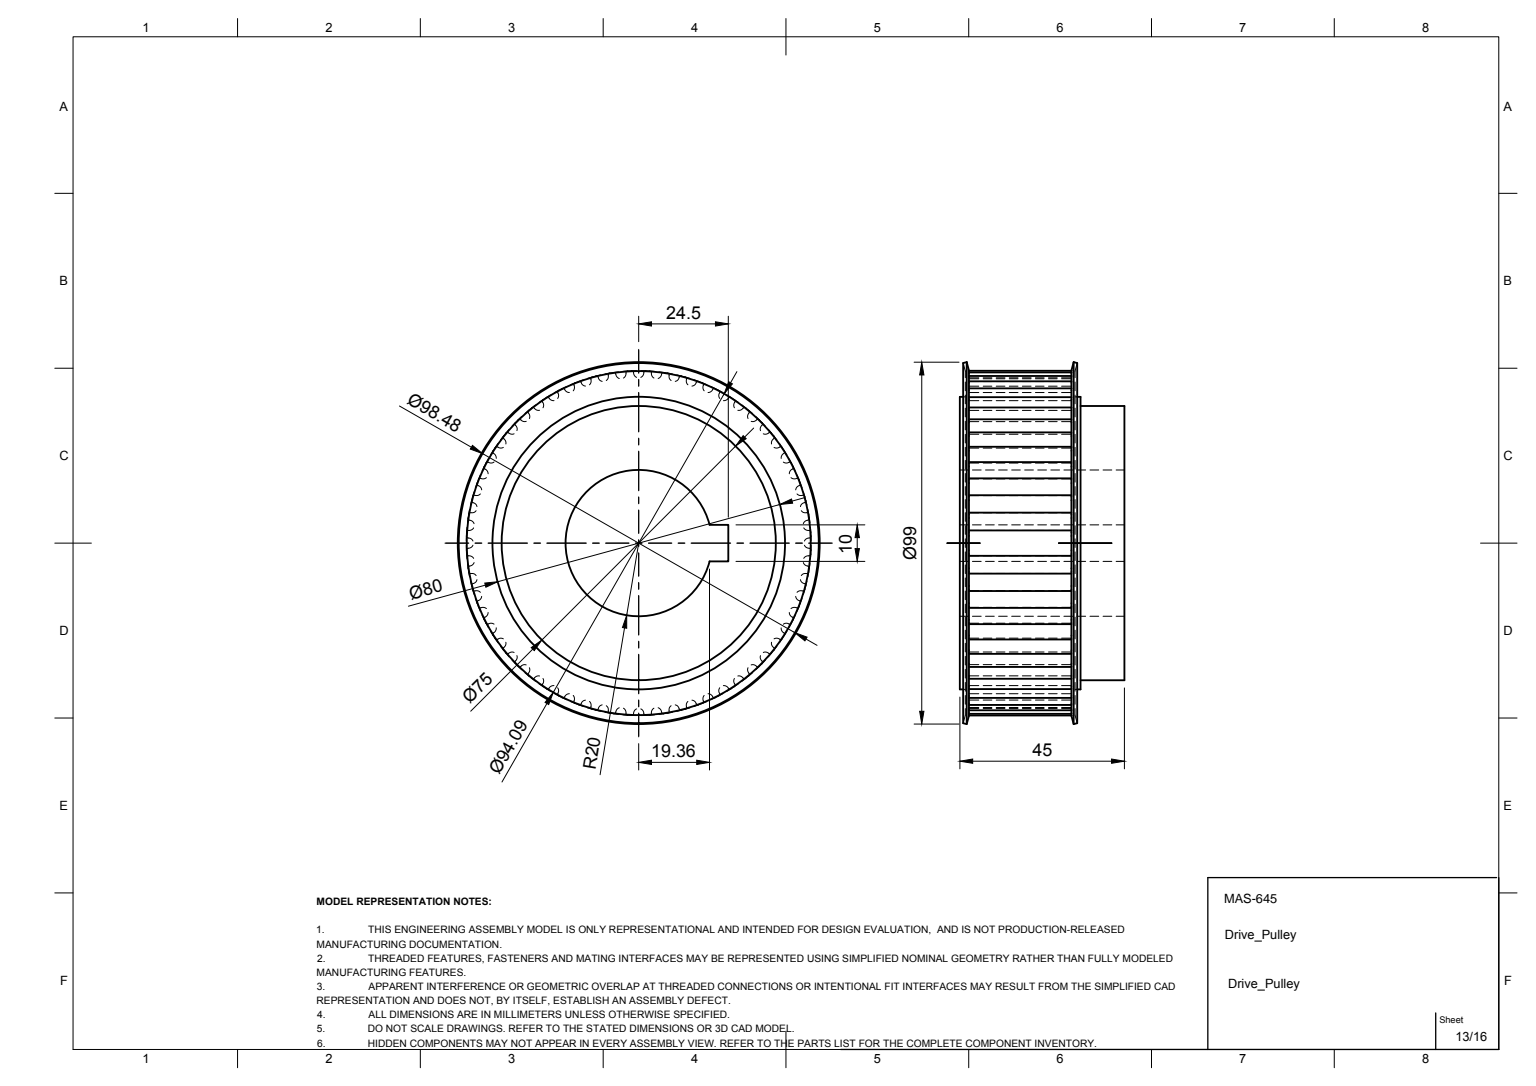
ISO-10303-21;
HEADER;
FILE_DESCRIPTION((''),'2;1');
FILE_NAME('Drive_Pulley.step','2026-10-09T10:54:55-07:00',(''),(''),'','','');
FILE_SCHEMA (('AUTOMOTIVE_DESIGN { 1 0 10303 214 3 1 1 }'));
ENDSEC;
DATA;
#10=MECHANICAL_DESIGN_GEOMETRIC_PRESENTATION_REPRESENTATION('',(#603),#63824);
#573=SHAPE_REPRESENTATION_RELATIONSHIP('SRR','None',#63887,#588) ;
#588=ADVANCED_BREP_SHAPE_REPRESENTATION('',(#618),#63817) ;
#603=STYLED_ITEM('',(#63965),#618) ;
#618=MANIFOLD_SOLID_BREP('Body1',#15502) ;
#750=FACE_BOUND('',#2823,.T.) ;
#751=FACE_BOUND('',#2886,.T.) ;
#752=FACE_BOUND('',#2894,.T.) ;
#753=FACE_BOUND('',#2897,.T.) ;
#754=FACE_BOUND('',#2900,.T.) ;
#908=PLANE('',#16209) ;
#909=PLANE('',#16210) ;
#910=PLANE('',#16211) ;
#911=PLANE('',#16212) ;
#912=PLANE('',#16397) ;
#913=PLANE('',#16536) ;
#914=PLANE('',#16540) ;
#915=PLANE('',#16544) ;
#916=PLANE('',#16546) ;
#917=PLANE('',#16550) ;
#918=PLANE('',#16557) ;
#919=PLANE('',#16561) ;
#920=PLANE('',#16568) ;
#921=PLANE('',#16572) ;
#922=PLANE('',#16579) ;
#923=PLANE('',#16583) ;
#924=PLANE('',#16590) ;
#925=PLANE('',#16594) ;
#926=PLANE('',#16601) ;
#927=PLANE('',#16605) ;
#928=PLANE('',#16612) ;
#929=PLANE('',#16616) ;
#930=PLANE('',#16623) ;
#931=PLANE('',#16627) ;
#932=PLANE('',#16634) ;
#933=PLANE('',#16638) ;
#934=PLANE('',#16645) ;
#935=PLANE('',#16649) ;
#936=PLANE('',#16656) ;
#937=PLANE('',#16660) ;
#938=PLANE('',#16667) ;
#939=PLANE('',#16671) ;
#940=PLANE('',#16678) ;
#941=PLANE('',#16682) ;
#942=PLANE('',#16689) ;
#943=PLANE('',#16693) ;
#944=PLANE('',#16700) ;
#945=PLANE('',#16704) ;
#946=PLANE('',#16711) ;
#947=PLANE('',#16715) ;
#948=PLANE('',#16722) ;
#949=PLANE('',#16726) ;
#950=PLANE('',#16733) ;
#951=PLANE('',#16737) ;
#952=PLANE('',#16744) ;
#953=PLANE('',#16748) ;
#954=PLANE('',#16755) ;
#955=PLANE('',#16759) ;
#956=PLANE('',#16766) ;
#957=PLANE('',#16770) ;
#958=PLANE('',#16777) ;
#959=PLANE('',#16781) ;
#960=PLANE('',#16788) ;
#961=PLANE('',#16792) ;
#962=PLANE('',#16799) ;
#963=PLANE('',#16803) ;
#964=PLANE('',#16810) ;
#965=PLANE('',#16814) ;
#966=PLANE('',#16821) ;
#967=PLANE('',#16825) ;
#968=PLANE('',#16832) ;
#969=PLANE('',#16836) ;
#970=PLANE('',#16843) ;
#971=PLANE('',#16847) ;
#972=PLANE('',#16854) ;
#973=PLANE('',#16858) ;
#974=PLANE('',#16865) ;
#975=PLANE('',#16869) ;
#976=PLANE('',#16876) ;
#977=PLANE('',#16880) ;
#978=PLANE('',#16887) ;
#979=PLANE('',#16891) ;
#980=PLANE('',#16898) ;
#981=PLANE('',#16902) ;
#982=PLANE('',#16909) ;
#983=PLANE('',#16913) ;
#984=PLANE('',#16920) ;
#985=PLANE('',#16924) ;
#986=PLANE('',#16931) ;
#987=PLANE('',#16935) ;
#988=PLANE('',#16942) ;
#989=PLANE('',#16946) ;
#990=PLANE('',#16953) ;
#991=PLANE('',#16957) ;
#992=PLANE('',#16964) ;
#993=PLANE('',#16968) ;
#994=PLANE('',#16975) ;
#995=PLANE('',#16979) ;
#996=PLANE('',#16986) ;
#997=PLANE('',#16990) ;
#998=PLANE('',#16997) ;
#999=PLANE('',#17001) ;
#1000=PLANE('',#17008) ;
#1001=PLANE('',#17012) ;
#1002=PLANE('',#17019) ;
#1003=PLANE('',#17023) ;
#1004=PLANE('',#17030) ;
#1005=PLANE('',#17034) ;
#1006=PLANE('',#17041) ;
#1007=PLANE('',#17045) ;
#1008=PLANE('',#17052) ;
#1009=PLANE('',#17056) ;
#1010=PLANE('',#17063) ;
#1011=PLANE('',#17067) ;
#1012=PLANE('',#17074) ;
#1013=PLANE('',#17078) ;
#1014=PLANE('',#17085) ;
#1015=PLANE('',#17089) ;
#1016=PLANE('',#17096) ;
#1017=PLANE('',#17100) ;
#1018=PLANE('',#17107) ;
#1019=PLANE('',#17111) ;
#1020=PLANE('',#17118) ;
#1021=PLANE('',#17122) ;
#1022=PLANE('',#17129) ;
#1023=PLANE('',#17133) ;
#1024=PLANE('',#17140) ;
#1025=PLANE('',#17144) ;
#1026=PLANE('',#17151) ;
#1027=PLANE('',#17155) ;
#1028=PLANE('',#17162) ;
#1029=PLANE('',#17166) ;
#1030=PLANE('',#17173) ;
#1031=PLANE('',#17177) ;
#1032=PLANE('',#17184) ;
#1033=PLANE('',#17188) ;
#1034=PLANE('',#17195) ;
#1035=PLANE('',#17199) ;
#1264=CYLINDRICAL_SURFACE('',#16215,47.175) ;
#1265=CYLINDRICAL_SURFACE('',#16218,47.175) ;
#1266=CYLINDRICAL_SURFACE('',#16221,47.175) ;
#1267=CYLINDRICAL_SURFACE('',#16224,47.175) ;
#1268=CYLINDRICAL_SURFACE('',#16227,47.175) ;
#1269=CYLINDRICAL_SURFACE('',#16230,47.175) ;
#1270=CYLINDRICAL_SURFACE('',#16233,47.175) ;
#1271=CYLINDRICAL_SURFACE('',#16236,47.175) ;
#1272=CYLINDRICAL_SURFACE('',#16239,47.175) ;
#1273=CYLINDRICAL_SURFACE('',#16242,47.175) ;
#1274=CYLINDRICAL_SURFACE('',#16245,47.175) ;
#1275=CYLINDRICAL_SURFACE('',#16248,47.175) ;
#1276=CYLINDRICAL_SURFACE('',#16251,47.175) ;
#1277=CYLINDRICAL_SURFACE('',#16254,47.175) ;
#1278=CYLINDRICAL_SURFACE('',#16257,47.175) ;
#1279=CYLINDRICAL_SURFACE('',#16260,47.175) ;
#1280=CYLINDRICAL_SURFACE('',#16263,47.175) ;
#1281=CYLINDRICAL_SURFACE('',#16266,47.175) ;
#1282=CYLINDRICAL_SURFACE('',#16269,47.175) ;
#1283=CYLINDRICAL_SURFACE('',#16272,47.175) ;
#1284=CYLINDRICAL_SURFACE('',#16275,47.175) ;
#1285=CYLINDRICAL_SURFACE('',#16278,47.175) ;
#1286=CYLINDRICAL_SURFACE('',#16281,47.175) ;
#1287=CYLINDRICAL_SURFACE('',#16284,47.175) ;
#1288=CYLINDRICAL_SURFACE('',#16287,47.175) ;
#1289=CYLINDRICAL_SURFACE('',#16290,47.175) ;
#1290=CYLINDRICAL_SURFACE('',#16293,47.175) ;
#1291=CYLINDRICAL_SURFACE('',#16296,47.175) ;
#1292=CYLINDRICAL_SURFACE('',#16299,47.175) ;
#1293=CYLINDRICAL_SURFACE('',#16302,47.175) ;
#1294=CYLINDRICAL_SURFACE('',#16305,47.175) ;
#1295=CYLINDRICAL_SURFACE('',#16308,47.175) ;
#1296=CYLINDRICAL_SURFACE('',#16311,47.175) ;
#1297=CYLINDRICAL_SURFACE('',#16314,47.175) ;
#1298=CYLINDRICAL_SURFACE('',#16317,47.175) ;
#1299=CYLINDRICAL_SURFACE('',#16320,47.175) ;
#1300=CYLINDRICAL_SURFACE('',#16323,47.175) ;
#1301=CYLINDRICAL_SURFACE('',#16326,47.175) ;
#1302=CYLINDRICAL_SURFACE('',#16329,47.175) ;
#1303=CYLINDRICAL_SURFACE('',#16332,47.175) ;
#1304=CYLINDRICAL_SURFACE('',#16335,47.175) ;
#1305=CYLINDRICAL_SURFACE('',#16338,47.175) ;
#1306=CYLINDRICAL_SURFACE('',#16341,47.175) ;
#1307=CYLINDRICAL_SURFACE('',#16344,47.175) ;
#1308=CYLINDRICAL_SURFACE('',#16347,47.175) ;
#1309=CYLINDRICAL_SURFACE('',#16350,47.175) ;
#1310=CYLINDRICAL_SURFACE('',#16353,47.175) ;
#1311=CYLINDRICAL_SURFACE('',#16356,47.175) ;
#1312=CYLINDRICAL_SURFACE('',#16359,47.175) ;
#1313=CYLINDRICAL_SURFACE('',#16362,47.175) ;
#1314=CYLINDRICAL_SURFACE('',#16365,47.175) ;
#1315=CYLINDRICAL_SURFACE('',#16368,47.175) ;
#1316=CYLINDRICAL_SURFACE('',#16371,47.175) ;
#1317=CYLINDRICAL_SURFACE('',#16374,47.175) ;
#1318=CYLINDRICAL_SURFACE('',#16377,47.175) ;
#1319=CYLINDRICAL_SURFACE('',#16380,47.175) ;
#1320=CYLINDRICAL_SURFACE('',#16383,47.175) ;
#1321=CYLINDRICAL_SURFACE('',#16386,47.175) ;
#1322=CYLINDRICAL_SURFACE('',#16389,47.175) ;
#1323=CYLINDRICAL_SURFACE('',#16392,47.175) ;
#1324=CYLINDRICAL_SURFACE('',#16395,40.) ;
#1325=CYLINDRICAL_SURFACE('',#16538,40.) ;
#1326=CYLINDRICAL_SURFACE('',#16542,37.5) ;
#1327=CYLINDRICAL_SURFACE('',#16554,0.539999999999996) ;
#1328=CYLINDRICAL_SURFACE('',#16555,1.4) ;
#1329=CYLINDRICAL_SURFACE('',#16556,0.539999999999986) ;
#1330=CYLINDRICAL_SURFACE('',#16565,0.539999999999996) ;
#1331=CYLINDRICAL_SURFACE('',#16566,1.4) ;
#1332=CYLINDRICAL_SURFACE('',#16567,0.539999999999986) ;
#1333=CYLINDRICAL_SURFACE('',#16576,0.539999999999996) ;
#1334=CYLINDRICAL_SURFACE('',#16577,1.4) ;
#1335=CYLINDRICAL_SURFACE('',#16578,0.539999999999986) ;
#1336=CYLINDRICAL_SURFACE('',#16587,0.539999999999996) ;
#1337=CYLINDRICAL_SURFACE('',#16588,1.4) ;
#1338=CYLINDRICAL_SURFACE('',#16589,0.539999999999986) ;
#1339=CYLINDRICAL_SURFACE('',#16598,0.539999999999996) ;
#1340=CYLINDRICAL_SURFACE('',#16599,1.4) ;
#1341=CYLINDRICAL_SURFACE('',#16600,0.539999999999986) ;
#1342=CYLINDRICAL_SURFACE('',#16609,0.539999999999996) ;
#1343=CYLINDRICAL_SURFACE('',#16610,1.4) ;
#1344=CYLINDRICAL_SURFACE('',#16611,0.539999999999986) ;
#1345=CYLINDRICAL_SURFACE('',#16620,0.539999999999996) ;
#1346=CYLINDRICAL_SURFACE('',#16621,1.4) ;
#1347=CYLINDRICAL_SURFACE('',#16622,0.539999999999986) ;
#1348=CYLINDRICAL_SURFACE('',#16631,0.539999999999996) ;
#1349=CYLINDRICAL_SURFACE('',#16632,1.4) ;
#1350=CYLINDRICAL_SURFACE('',#16633,0.539999999999986) ;
#1351=CYLINDRICAL_SURFACE('',#16642,0.539999999999996) ;
#1352=CYLINDRICAL_SURFACE('',#16643,1.4) ;
#1353=CYLINDRICAL_SURFACE('',#16644,0.539999999999986) ;
#1354=CYLINDRICAL_SURFACE('',#16653,0.539999999999996) ;
#1355=CYLINDRICAL_SURFACE('',#16654,1.4) ;
#1356=CYLINDRICAL_SURFACE('',#16655,0.539999999999986) ;
#1357=CYLINDRICAL_SURFACE('',#16664,0.539999999999996) ;
#1358=CYLINDRICAL_SURFACE('',#16665,1.4) ;
#1359=CYLINDRICAL_SURFACE('',#16666,0.539999999999986) ;
#1360=CYLINDRICAL_SURFACE('',#16675,0.539999999999996) ;
#1361=CYLINDRICAL_SURFACE('',#16676,1.4) ;
#1362=CYLINDRICAL_SURFACE('',#16677,0.539999999999986) ;
#1363=CYLINDRICAL_SURFACE('',#16686,0.539999999999996) ;
#1364=CYLINDRICAL_SURFACE('',#16687,1.4) ;
#1365=CYLINDRICAL_SURFACE('',#16688,0.539999999999986) ;
#1366=CYLINDRICAL_SURFACE('',#16697,0.539999999999996) ;
#1367=CYLINDRICAL_SURFACE('',#16698,1.4) ;
#1368=CYLINDRICAL_SURFACE('',#16699,0.539999999999986) ;
#1369=CYLINDRICAL_SURFACE('',#16708,0.539999999999996) ;
#1370=CYLINDRICAL_SURFACE('',#16709,1.4) ;
#1371=CYLINDRICAL_SURFACE('',#16710,0.539999999999986) ;
#1372=CYLINDRICAL_SURFACE('',#16719,0.539999999999996) ;
#1373=CYLINDRICAL_SURFACE('',#16720,1.4) ;
#1374=CYLINDRICAL_SURFACE('',#16721,0.539999999999986) ;
#1375=CYLINDRICAL_SURFACE('',#16730,0.539999999999996) ;
#1376=CYLINDRICAL_SURFACE('',#16731,1.4) ;
#1377=CYLINDRICAL_SURFACE('',#16732,0.539999999999986) ;
#1378=CYLINDRICAL_SURFACE('',#16741,0.539999999999996) ;
#1379=CYLINDRICAL_SURFACE('',#16742,1.4) ;
#1380=CYLINDRICAL_SURFACE('',#16743,0.539999999999986) ;
#1381=CYLINDRICAL_SURFACE('',#16752,0.539999999999996) ;
#1382=CYLINDRICAL_SURFACE('',#16753,1.4) ;
#1383=CYLINDRICAL_SURFACE('',#16754,0.539999999999986) ;
#1384=CYLINDRICAL_SURFACE('',#16763,0.539999999999996) ;
#1385=CYLINDRICAL_SURFACE('',#16764,1.4) ;
#1386=CYLINDRICAL_SURFACE('',#16765,0.539999999999986) ;
#1387=CYLINDRICAL_SURFACE('',#16774,0.539999999999996) ;
#1388=CYLINDRICAL_SURFACE('',#16775,1.4) ;
#1389=CYLINDRICAL_SURFACE('',#16776,0.539999999999986) ;
#1390=CYLINDRICAL_SURFACE('',#16785,0.539999999999996) ;
#1391=CYLINDRICAL_SURFACE('',#16786,1.4) ;
#1392=CYLINDRICAL_SURFACE('',#16787,0.539999999999986) ;
#1393=CYLINDRICAL_SURFACE('',#16796,0.539999999999996) ;
#1394=CYLINDRICAL_SURFACE('',#16797,1.4) ;
#1395=CYLINDRICAL_SURFACE('',#16798,0.539999999999986) ;
#1396=CYLINDRICAL_SURFACE('',#16807,0.539999999999996) ;
#1397=CYLINDRICAL_SURFACE('',#16808,1.4) ;
#1398=CYLINDRICAL_SURFACE('',#16809,0.539999999999986) ;
#1399=CYLINDRICAL_SURFACE('',#16818,0.539999999999996) ;
#1400=CYLINDRICAL_SURFACE('',#16819,1.4) ;
#1401=CYLINDRICAL_SURFACE('',#16820,0.539999999999986) ;
#1402=CYLINDRICAL_SURFACE('',#16829,0.539999999999996) ;
#1403=CYLINDRICAL_SURFACE('',#16830,1.4) ;
#1404=CYLINDRICAL_SURFACE('',#16831,0.539999999999986) ;
#1405=CYLINDRICAL_SURFACE('',#16840,0.539999999999996) ;
#1406=CYLINDRICAL_SURFACE('',#16841,1.4) ;
#1407=CYLINDRICAL_SURFACE('',#16842,0.539999999999986) ;
#1408=CYLINDRICAL_SURFACE('',#16851,0.539999999999996) ;
#1409=CYLINDRICAL_SURFACE('',#16852,1.4) ;
#1410=CYLINDRICAL_SURFACE('',#16853,0.539999999999986) ;
#1411=CYLINDRICAL_SURFACE('',#16862,0.539999999999996) ;
#1412=CYLINDRICAL_SURFACE('',#16863,1.4) ;
#1413=CYLINDRICAL_SURFACE('',#16864,0.539999999999986) ;
#1414=CYLINDRICAL_SURFACE('',#16873,0.539999999999996) ;
#1415=CYLINDRICAL_SURFACE('',#16874,1.4) ;
#1416=CYLINDRICAL_SURFACE('',#16875,0.539999999999986) ;
#1417=CYLINDRICAL_SURFACE('',#16884,0.539999999999996) ;
#1418=CYLINDRICAL_SURFACE('',#16885,1.4) ;
#1419=CYLINDRICAL_SURFACE('',#16886,0.539999999999986) ;
#1420=CYLINDRICAL_SURFACE('',#16895,0.539999999999996) ;
#1421=CYLINDRICAL_SURFACE('',#16896,1.4) ;
#1422=CYLINDRICAL_SURFACE('',#16897,0.539999999999986) ;
#1423=CYLINDRICAL_SURFACE('',#16906,0.539999999999996) ;
#1424=CYLINDRICAL_SURFACE('',#16907,1.4) ;
#1425=CYLINDRICAL_SURFACE('',#16908,0.539999999999986) ;
#1426=CYLINDRICAL_SURFACE('',#16917,0.539999999999996) ;
#1427=CYLINDRICAL_SURFACE('',#16918,1.4) ;
#1428=CYLINDRICAL_SURFACE('',#16919,0.539999999999986) ;
#1429=CYLINDRICAL_SURFACE('',#16928,0.539999999999996) ;
#1430=CYLINDRICAL_SURFACE('',#16929,1.4) ;
#1431=CYLINDRICAL_SURFACE('',#16930,0.539999999999986) ;
#1432=CYLINDRICAL_SURFACE('',#16939,0.539999999999996) ;
#1433=CYLINDRICAL_SURFACE('',#16940,1.4) ;
#1434=CYLINDRICAL_SURFACE('',#16941,0.539999999999986) ;
#1435=CYLINDRICAL_SURFACE('',#16950,0.539999999999996) ;
#1436=CYLINDRICAL_SURFACE('',#16951,1.4) ;
#1437=CYLINDRICAL_SURFACE('',#16952,0.539999999999986) ;
#1438=CYLINDRICAL_SURFACE('',#16961,0.539999999999996) ;
#1439=CYLINDRICAL_SURFACE('',#16962,1.4) ;
#1440=CYLINDRICAL_SURFACE('',#16963,0.539999999999986) ;
#1441=CYLINDRICAL_SURFACE('',#16972,0.539999999999996) ;
#1442=CYLINDRICAL_SURFACE('',#16973,1.4) ;
#1443=CYLINDRICAL_SURFACE('',#16974,0.539999999999986) ;
#1444=CYLINDRICAL_SURFACE('',#16983,0.539999999999996) ;
#1445=CYLINDRICAL_SURFACE('',#16984,1.4) ;
#1446=CYLINDRICAL_SURFACE('',#16985,0.539999999999986) ;
#1447=CYLINDRICAL_SURFACE('',#16994,0.539999999999996) ;
#1448=CYLINDRICAL_SURFACE('',#16995,1.4) ;
#1449=CYLINDRICAL_SURFACE('',#16996,0.539999999999986) ;
#1450=CYLINDRICAL_SURFACE('',#17005,0.539999999999996) ;
#1451=CYLINDRICAL_SURFACE('',#17006,1.4) ;
#1452=CYLINDRICAL_SURFACE('',#17007,0.539999999999986) ;
#1453=CYLINDRICAL_SURFACE('',#17016,0.539999999999996) ;
#1454=CYLINDRICAL_SURFACE('',#17017,1.4) ;
#1455=CYLINDRICAL_SURFACE('',#17018,0.539999999999986) ;
#1456=CYLINDRICAL_SURFACE('',#17027,0.539999999999996) ;
#1457=CYLINDRICAL_SURFACE('',#17028,1.4) ;
#1458=CYLINDRICAL_SURFACE('',#17029,0.539999999999986) ;
#1459=CYLINDRICAL_SURFACE('',#17038,0.539999999999996) ;
#1460=CYLINDRICAL_SURFACE('',#17039,1.4) ;
#1461=CYLINDRICAL_SURFACE('',#17040,0.539999999999986) ;
#1462=CYLINDRICAL_SURFACE('',#17049,0.539999999999996) ;
#1463=CYLINDRICAL_SURFACE('',#17050,1.4) ;
#1464=CYLINDRICAL_SURFACE('',#17051,0.539999999999986) ;
#1465=CYLINDRICAL_SURFACE('',#17060,0.539999999999996) ;
#1466=CYLINDRICAL_SURFACE('',#17061,1.4) ;
#1467=CYLINDRICAL_SURFACE('',#17062,0.539999999999986) ;
#1468=CYLINDRICAL_SURFACE('',#17071,0.539999999999996) ;
#1469=CYLINDRICAL_SURFACE('',#17072,1.4) ;
#1470=CYLINDRICAL_SURFACE('',#17073,0.539999999999986) ;
#1471=CYLINDRICAL_SURFACE('',#17082,0.539999999999996) ;
#1472=CYLINDRICAL_SURFACE('',#17083,1.4) ;
#1473=CYLINDRICAL_SURFACE('',#17084,0.539999999999986) ;
#1474=CYLINDRICAL_SURFACE('',#17093,0.539999999999996) ;
#1475=CYLINDRICAL_SURFACE('',#17094,1.4) ;
#1476=CYLINDRICAL_SURFACE('',#17095,0.539999999999986) ;
#1477=CYLINDRICAL_SURFACE('',#17104,0.539999999999996) ;
#1478=CYLINDRICAL_SURFACE('',#17105,1.4) ;
#1479=CYLINDRICAL_SURFACE('',#17106,0.539999999999986) ;
#1480=CYLINDRICAL_SURFACE('',#17115,0.539999999999996) ;
#1481=CYLINDRICAL_SURFACE('',#17116,1.4) ;
#1482=CYLINDRICAL_SURFACE('',#17117,0.539999999999986) ;
#1483=CYLINDRICAL_SURFACE('',#17126,0.539999999999996) ;
#1484=CYLINDRICAL_SURFACE('',#17127,1.4) ;
#1485=CYLINDRICAL_SURFACE('',#17128,0.539999999999986) ;
#1486=CYLINDRICAL_SURFACE('',#17137,0.539999999999996) ;
#1487=CYLINDRICAL_SURFACE('',#17138,1.4) ;
#1488=CYLINDRICAL_SURFACE('',#17139,0.539999999999986) ;
#1489=CYLINDRICAL_SURFACE('',#17148,0.539999999999996) ;
#1490=CYLINDRICAL_SURFACE('',#17149,1.4) ;
#1491=CYLINDRICAL_SURFACE('',#17150,0.539999999999986) ;
#1492=CYLINDRICAL_SURFACE('',#17159,0.539999999999996) ;
#1493=CYLINDRICAL_SURFACE('',#17160,1.4) ;
#1494=CYLINDRICAL_SURFACE('',#17161,0.539999999999986) ;
#1495=CYLINDRICAL_SURFACE('',#17170,0.539999999999996) ;
#1496=CYLINDRICAL_SURFACE('',#17171,1.4) ;
#1497=CYLINDRICAL_SURFACE('',#17172,0.539999999999986) ;
#1498=CYLINDRICAL_SURFACE('',#17181,0.539999999999996) ;
#1499=CYLINDRICAL_SURFACE('',#17182,1.4) ;
#1500=CYLINDRICAL_SURFACE('',#17183,0.539999999999986) ;
#1501=CYLINDRICAL_SURFACE('',#17192,0.539999999999996) ;
#1502=CYLINDRICAL_SURFACE('',#17193,1.4) ;
#1503=CYLINDRICAL_SURFACE('',#17194,0.539999999999986) ;
#1504=CYLINDRICAL_SURFACE('',#17203,0.539999999999996) ;
#1505=CYLINDRICAL_SURFACE('',#17204,1.4) ;
#1506=CYLINDRICAL_SURFACE('',#17205,0.539999999999986) ;
#1507=CYLINDRICAL_SURFACE('',#17206,20.) ;
#1833=FACE_OUTER_BOUND('',#2819,.T.) ;
#1834=FACE_OUTER_BOUND('',#2820,.T.) ;
#1835=FACE_OUTER_BOUND('',#2821,.T.) ;
#1836=FACE_OUTER_BOUND('',#2822,.T.) ;
#1837=FACE_OUTER_BOUND('',#2824,.T.) ;
#1838=FACE_OUTER_BOUND('',#2825,.T.) ;
#1839=FACE_OUTER_BOUND('',#2826,.T.) ;
#1840=FACE_OUTER_BOUND('',#2827,.T.) ;
#1841=FACE_OUTER_BOUND('',#2828,.T.) ;
#1842=FACE_OUTER_BOUND('',#2829,.T.) ;
#1843=FACE_OUTER_BOUND('',#2830,.T.) ;
#1844=FACE_OUTER_BOUND('',#2831,.T.) ;
#1845=FACE_OUTER_BOUND('',#2832,.T.) ;
#1846=FACE_OUTER_BOUND('',#2833,.T.) ;
#1847=FACE_OUTER_BOUND('',#2834,.T.) ;
#1848=FACE_OUTER_BOUND('',#2835,.T.) ;
#1849=FACE_OUTER_BOUND('',#2836,.T.) ;
#1850=FACE_OUTER_BOUND('',#2837,.T.) ;
#1851=FACE_OUTER_BOUND('',#2838,.T.) ;
#1852=FACE_OUTER_BOUND('',#2839,.T.) ;
#1853=FACE_OUTER_BOUND('',#2840,.T.) ;
#1854=FACE_OUTER_BOUND('',#2841,.T.) ;
#1855=FACE_OUTER_BOUND('',#2842,.T.) ;
#1856=FACE_OUTER_BOUND('',#2843,.T.) ;
#1857=FACE_OUTER_BOUND('',#2844,.T.) ;
#1858=FACE_OUTER_BOUND('',#2845,.T.) ;
#1859=FACE_OUTER_BOUND('',#2846,.T.) ;
#1860=FACE_OUTER_BOUND('',#2847,.T.) ;
#1861=FACE_OUTER_BOUND('',#2848,.T.) ;
#1862=FACE_OUTER_BOUND('',#2849,.T.) ;
#1863=FACE_OUTER_BOUND('',#2850,.T.) ;
#1864=FACE_OUTER_BOUND('',#2851,.T.) ;
#1865=FACE_OUTER_BOUND('',#2852,.T.) ;
#1866=FACE_OUTER_BOUND('',#2853,.T.) ;
#1867=FACE_OUTER_BOUND('',#2854,.T.) ;
#1868=FACE_OUTER_BOUND('',#2855,.T.) ;
#1869=FACE_OUTER_BOUND('',#2856,.T.) ;
#1870=FACE_OUTER_BOUND('',#2857,.T.) ;
#1871=FACE_OUTER_BOUND('',#2858,.T.) ;
#1872=FACE_OUTER_BOUND('',#2859,.T.) ;
#1873=FACE_OUTER_BOUND('',#2860,.T.) ;
#1874=FACE_OUTER_BOUND('',#2861,.T.) ;
#1875=FACE_OUTER_BOUND('',#2862,.T.) ;
#1876=FACE_OUTER_BOUND('',#2863,.T.) ;
#1877=FACE_OUTER_BOUND('',#2864,.T.) ;
#1878=FACE_OUTER_BOUND('',#2865,.T.) ;
#1879=FACE_OUTER_BOUND('',#2866,.T.) ;
#1880=FACE_OUTER_BOUND('',#2867,.T.) ;
#1881=FACE_OUTER_BOUND('',#2868,.T.) ;
#1882=FACE_OUTER_BOUND('',#2869,.T.) ;
#1883=FACE_OUTER_BOUND('',#2870,.T.) ;
#1884=FACE_OUTER_BOUND('',#2871,.T.) ;
#1885=FACE_OUTER_BOUND('',#2872,.T.) ;
#1886=FACE_OUTER_BOUND('',#2873,.T.) ;
#1887=FACE_OUTER_BOUND('',#2874,.T.) ;
#1888=FACE_OUTER_BOUND('',#2875,.T.) ;
#1889=FACE_OUTER_BOUND('',#2876,.T.) ;
#1890=FACE_OUTER_BOUND('',#2877,.T.) ;
#1891=FACE_OUTER_BOUND('',#2878,.T.) ;
#1892=FACE_OUTER_BOUND('',#2879,.T.) ;
#1893=FACE_OUTER_BOUND('',#2880,.T.) ;
#1894=FACE_OUTER_BOUND('',#2881,.T.) ;
#1895=FACE_OUTER_BOUND('',#2882,.T.) ;
#1896=FACE_OUTER_BOUND('',#2883,.T.) ;
#1897=FACE_OUTER_BOUND('',#2884,.T.) ;
#1898=FACE_OUTER_BOUND('',#2885,.T.) ;
#1899=FACE_OUTER_BOUND('',#2887,.T.) ;
#1900=FACE_OUTER_BOUND('',#2888,.T.) ;
#1901=FACE_OUTER_BOUND('',#2889,.T.) ;
#1902=FACE_OUTER_BOUND('',#2890,.T.) ;
#1903=FACE_OUTER_BOUND('',#2891,.T.) ;
#1904=FACE_OUTER_BOUND('',#2892,.T.) ;
#1905=FACE_OUTER_BOUND('',#2893,.T.) ;
#1906=FACE_OUTER_BOUND('',#2895,.T.) ;
#1907=FACE_OUTER_BOUND('',#2896,.T.) ;
#1908=FACE_OUTER_BOUND('',#2898,.T.) ;
#1909=FACE_OUTER_BOUND('',#2899,.T.) ;
#1910=FACE_OUTER_BOUND('',#2901,.T.) ;
#1911=FACE_OUTER_BOUND('',#2902,.T.) ;
#1912=FACE_OUTER_BOUND('',#2903,.T.) ;
#1913=FACE_OUTER_BOUND('',#2904,.T.) ;
#1914=FACE_OUTER_BOUND('',#2905,.T.) ;
#1915=FACE_OUTER_BOUND('',#2906,.T.) ;
#1916=FACE_OUTER_BOUND('',#2907,.T.) ;
#1917=FACE_OUTER_BOUND('',#2908,.T.) ;
#1918=FACE_OUTER_BOUND('',#2909,.T.) ;
#1919=FACE_OUTER_BOUND('',#2910,.T.) ;
#1920=FACE_OUTER_BOUND('',#2911,.T.) ;
#1921=FACE_OUTER_BOUND('',#2912,.T.) ;
#1922=FACE_OUTER_BOUND('',#2913,.T.) ;
#1923=FACE_OUTER_BOUND('',#2914,.T.) ;
#1924=FACE_OUTER_BOUND('',#2915,.T.) ;
#1925=FACE_OUTER_BOUND('',#2916,.T.) ;
#1926=FACE_OUTER_BOUND('',#2917,.T.) ;
#1927=FACE_OUTER_BOUND('',#2918,.T.) ;
#1928=FACE_OUTER_BOUND('',#2919,.T.) ;
#1929=FACE_OUTER_BOUND('',#2920,.T.) ;
#1930=FACE_OUTER_BOUND('',#2921,.T.) ;
#1931=FACE_OUTER_BOUND('',#2922,.T.) ;
#1932=FACE_OUTER_BOUND('',#2923,.T.) ;
#1933=FACE_OUTER_BOUND('',#2924,.T.) ;
#1934=FACE_OUTER_BOUND('',#2925,.T.) ;
#1935=FACE_OUTER_BOUND('',#2926,.T.) ;
#1936=FACE_OUTER_BOUND('',#2927,.T.) ;
#1937=FACE_OUTER_BOUND('',#2928,.T.) ;
#1938=FACE_OUTER_BOUND('',#2929,.T.) ;
#1939=FACE_OUTER_BOUND('',#2930,.T.) ;
#1940=FACE_OUTER_BOUND('',#2931,.T.) ;
#1941=FACE_OUTER_BOUND('',#2932,.T.) ;
#1942=FACE_OUTER_BOUND('',#2933,.T.) ;
#1943=FACE_OUTER_BOUND('',#2934,.T.) ;
#1944=FACE_OUTER_BOUND('',#2935,.T.) ;
#1945=FACE_OUTER_BOUND('',#2936,.T.) ;
#1946=FACE_OUTER_BOUND('',#2937,.T.) ;
#1947=FACE_OUTER_BOUND('',#2938,.T.) ;
#1948=FACE_OUTER_BOUND('',#2939,.T.) ;
#1949=FACE_OUTER_BOUND('',#2940,.T.) ;
#1950=FACE_OUTER_BOUND('',#2941,.T.) ;
#1951=FACE_OUTER_BOUND('',#2942,.T.) ;
#1952=FACE_OUTER_BOUND('',#2943,.T.) ;
#1953=FACE_OUTER_BOUND('',#2944,.T.) ;
#1954=FACE_OUTER_BOUND('',#2945,.T.) ;
#1955=FACE_OUTER_BOUND('',#2946,.T.) ;
#1956=FACE_OUTER_BOUND('',#2947,.T.) ;
#1957=FACE_OUTER_BOUND('',#2948,.T.) ;
#1958=FACE_OUTER_BOUND('',#2949,.T.) ;
#1959=FACE_OUTER_BOUND('',#2950,.T.) ;
#1960=FACE_OUTER_BOUND('',#2951,.T.) ;
#1961=FACE_OUTER_BOUND('',#2952,.T.) ;
#1962=FACE_OUTER_BOUND('',#2953,.T.) ;
#1963=FACE_OUTER_BOUND('',#2954,.T.) ;
#1964=FACE_OUTER_BOUND('',#2955,.T.) ;
#1965=FACE_OUTER_BOUND('',#2956,.T.) ;
#1966=FACE_OUTER_BOUND('',#2957,.T.) ;
#1967=FACE_OUTER_BOUND('',#2958,.T.) ;
#1968=FACE_OUTER_BOUND('',#2959,.T.) ;
#1969=FACE_OUTER_BOUND('',#2960,.T.) ;
#1970=FACE_OUTER_BOUND('',#2961,.T.) ;
#1971=FACE_OUTER_BOUND('',#2962,.T.) ;
#1972=FACE_OUTER_BOUND('',#2963,.T.) ;
#1973=FACE_OUTER_BOUND('',#2964,.T.) ;
#1974=FACE_OUTER_BOUND('',#2965,.T.) ;
#1975=FACE_OUTER_BOUND('',#2966,.T.) ;
#1976=FACE_OUTER_BOUND('',#2967,.T.) ;
#1977=FACE_OUTER_BOUND('',#2968,.T.) ;
#1978=FACE_OUTER_BOUND('',#2969,.T.) ;
#1979=FACE_OUTER_BOUND('',#2970,.T.) ;
#1980=FACE_OUTER_BOUND('',#2971,.T.) ;
#1981=FACE_OUTER_BOUND('',#2972,.T.) ;
#1982=FACE_OUTER_BOUND('',#2973,.T.) ;
#1983=FACE_OUTER_BOUND('',#2974,.T.) ;
#1984=FACE_OUTER_BOUND('',#2975,.T.) ;
#1985=FACE_OUTER_BOUND('',#2976,.T.) ;
#1986=FACE_OUTER_BOUND('',#2977,.T.) ;
#1987=FACE_OUTER_BOUND('',#2978,.T.) ;
#1988=FACE_OUTER_BOUND('',#2979,.T.) ;
#1989=FACE_OUTER_BOUND('',#2980,.T.) ;
#1990=FACE_OUTER_BOUND('',#2981,.T.) ;
#1991=FACE_OUTER_BOUND('',#2982,.T.) ;
#1992=FACE_OUTER_BOUND('',#2983,.T.) ;
#1993=FACE_OUTER_BOUND('',#2984,.T.) ;
#1994=FACE_OUTER_BOUND('',#2985,.T.) ;
#1995=FACE_OUTER_BOUND('',#2986,.T.) ;
#1996=FACE_OUTER_BOUND('',#2987,.T.) ;
#1997=FACE_OUTER_BOUND('',#2988,.T.) ;
#1998=FACE_OUTER_BOUND('',#2989,.T.) ;
#1999=FACE_OUTER_BOUND('',#2990,.T.) ;
#2000=FACE_OUTER_BOUND('',#2991,.T.) ;
#2001=FACE_OUTER_BOUND('',#2992,.T.) ;
#2002=FACE_OUTER_BOUND('',#2993,.T.) ;
#2003=FACE_OUTER_BOUND('',#2994,.T.) ;
#2004=FACE_OUTER_BOUND('',#2995,.T.) ;
#2005=FACE_OUTER_BOUND('',#2996,.T.) ;
#2006=FACE_OUTER_BOUND('',#2997,.T.) ;
#2007=FACE_OUTER_BOUND('',#2998,.T.) ;
#2008=FACE_OUTER_BOUND('',#2999,.T.) ;
#2009=FACE_OUTER_BOUND('',#3000,.T.) ;
#2010=FACE_OUTER_BOUND('',#3001,.T.) ;
#2011=FACE_OUTER_BOUND('',#3002,.T.) ;
#2012=FACE_OUTER_BOUND('',#3003,.T.) ;
#2013=FACE_OUTER_BOUND('',#3004,.T.) ;
#2014=FACE_OUTER_BOUND('',#3005,.T.) ;
#2015=FACE_OUTER_BOUND('',#3006,.T.) ;
#2016=FACE_OUTER_BOUND('',#3007,.T.) ;
#2017=FACE_OUTER_BOUND('',#3008,.T.) ;
#2018=FACE_OUTER_BOUND('',#3009,.T.) ;
#2019=FACE_OUTER_BOUND('',#3010,.T.) ;
#2020=FACE_OUTER_BOUND('',#3011,.T.) ;
#2021=FACE_OUTER_BOUND('',#3012,.T.) ;
#2022=FACE_OUTER_BOUND('',#3013,.T.) ;
#2023=FACE_OUTER_BOUND('',#3014,.T.) ;
#2024=FACE_OUTER_BOUND('',#3015,.T.) ;
#2025=FACE_OUTER_BOUND('',#3016,.T.) ;
#2026=FACE_OUTER_BOUND('',#3017,.T.) ;
#2027=FACE_OUTER_BOUND('',#3018,.T.) ;
#2028=FACE_OUTER_BOUND('',#3019,.T.) ;
#2029=FACE_OUTER_BOUND('',#3020,.T.) ;
#2030=FACE_OUTER_BOUND('',#3021,.T.) ;
#2031=FACE_OUTER_BOUND('',#3022,.T.) ;
#2032=FACE_OUTER_BOUND('',#3023,.T.) ;
#2033=FACE_OUTER_BOUND('',#3024,.T.) ;
#2034=FACE_OUTER_BOUND('',#3025,.T.) ;
#2035=FACE_OUTER_BOUND('',#3026,.T.) ;
#2036=FACE_OUTER_BOUND('',#3027,.T.) ;
#2037=FACE_OUTER_BOUND('',#3028,.T.) ;
#2038=FACE_OUTER_BOUND('',#3029,.T.) ;
#2039=FACE_OUTER_BOUND('',#3030,.T.) ;
#2040=FACE_OUTER_BOUND('',#3031,.T.) ;
#2041=FACE_OUTER_BOUND('',#3032,.T.) ;
#2042=FACE_OUTER_BOUND('',#3033,.T.) ;
#2043=FACE_OUTER_BOUND('',#3034,.T.) ;
#2044=FACE_OUTER_BOUND('',#3035,.T.) ;
#2045=FACE_OUTER_BOUND('',#3036,.T.) ;
#2046=FACE_OUTER_BOUND('',#3037,.T.) ;
#2047=FACE_OUTER_BOUND('',#3038,.T.) ;
#2048=FACE_OUTER_BOUND('',#3039,.T.) ;
#2049=FACE_OUTER_BOUND('',#3040,.T.) ;
#2050=FACE_OUTER_BOUND('',#3041,.T.) ;
#2051=FACE_OUTER_BOUND('',#3042,.T.) ;
#2052=FACE_OUTER_BOUND('',#3043,.T.) ;
#2053=FACE_OUTER_BOUND('',#3044,.T.) ;
#2054=FACE_OUTER_BOUND('',#3045,.T.) ;
#2055=FACE_OUTER_BOUND('',#3046,.T.) ;
#2056=FACE_OUTER_BOUND('',#3047,.T.) ;
#2057=FACE_OUTER_BOUND('',#3048,.T.) ;
#2058=FACE_OUTER_BOUND('',#3049,.T.) ;
#2059=FACE_OUTER_BOUND('',#3050,.T.) ;
#2060=FACE_OUTER_BOUND('',#3051,.T.) ;
#2061=FACE_OUTER_BOUND('',#3052,.T.) ;
#2062=FACE_OUTER_BOUND('',#3053,.T.) ;
#2063=FACE_OUTER_BOUND('',#3054,.T.) ;
#2064=FACE_OUTER_BOUND('',#3055,.T.) ;
#2065=FACE_OUTER_BOUND('',#3056,.T.) ;
#2066=FACE_OUTER_BOUND('',#3057,.T.) ;
#2067=FACE_OUTER_BOUND('',#3058,.T.) ;
#2068=FACE_OUTER_BOUND('',#3059,.T.) ;
#2069=FACE_OUTER_BOUND('',#3060,.T.) ;
#2070=FACE_OUTER_BOUND('',#3061,.T.) ;
#2071=FACE_OUTER_BOUND('',#3062,.T.) ;
#2072=FACE_OUTER_BOUND('',#3063,.T.) ;
#2073=FACE_OUTER_BOUND('',#3064,.T.) ;
#2074=FACE_OUTER_BOUND('',#3065,.T.) ;
#2075=FACE_OUTER_BOUND('',#3066,.T.) ;
#2076=FACE_OUTER_BOUND('',#3067,.T.) ;
#2077=FACE_OUTER_BOUND('',#3068,.T.) ;
#2078=FACE_OUTER_BOUND('',#3069,.T.) ;
#2079=FACE_OUTER_BOUND('',#3070,.T.) ;
#2080=FACE_OUTER_BOUND('',#3071,.T.) ;
#2081=FACE_OUTER_BOUND('',#3072,.T.) ;
#2082=FACE_OUTER_BOUND('',#3073,.T.) ;
#2083=FACE_OUTER_BOUND('',#3074,.T.) ;
#2084=FACE_OUTER_BOUND('',#3075,.T.) ;
#2085=FACE_OUTER_BOUND('',#3076,.T.) ;
#2086=FACE_OUTER_BOUND('',#3077,.T.) ;
#2087=FACE_OUTER_BOUND('',#3078,.T.) ;
#2088=FACE_OUTER_BOUND('',#3079,.T.) ;
#2089=FACE_OUTER_BOUND('',#3080,.T.) ;
#2090=FACE_OUTER_BOUND('',#3081,.T.) ;
#2091=FACE_OUTER_BOUND('',#3082,.T.) ;
#2092=FACE_OUTER_BOUND('',#3083,.T.) ;
#2093=FACE_OUTER_BOUND('',#3084,.T.) ;
#2094=FACE_OUTER_BOUND('',#3085,.T.) ;
#2095=FACE_OUTER_BOUND('',#3086,.T.) ;
#2096=FACE_OUTER_BOUND('',#3087,.T.) ;
#2097=FACE_OUTER_BOUND('',#3088,.T.) ;
#2098=FACE_OUTER_BOUND('',#3089,.T.) ;
#2099=FACE_OUTER_BOUND('',#3090,.T.) ;
#2100=FACE_OUTER_BOUND('',#3091,.T.) ;
#2101=FACE_OUTER_BOUND('',#3092,.T.) ;
#2102=FACE_OUTER_BOUND('',#3093,.T.) ;
#2103=FACE_OUTER_BOUND('',#3094,.T.) ;
#2104=FACE_OUTER_BOUND('',#3095,.T.) ;
#2105=FACE_OUTER_BOUND('',#3096,.T.) ;
#2106=FACE_OUTER_BOUND('',#3097,.T.) ;
#2107=FACE_OUTER_BOUND('',#3098,.T.) ;
#2108=FACE_OUTER_BOUND('',#3099,.T.) ;
#2109=FACE_OUTER_BOUND('',#3100,.T.) ;
#2110=FACE_OUTER_BOUND('',#3101,.T.) ;
#2111=FACE_OUTER_BOUND('',#3102,.T.) ;
#2112=FACE_OUTER_BOUND('',#3103,.T.) ;
#2113=FACE_OUTER_BOUND('',#3104,.T.) ;
#2114=FACE_OUTER_BOUND('',#3105,.T.) ;
#2115=FACE_OUTER_BOUND('',#3106,.T.) ;
#2116=FACE_OUTER_BOUND('',#3107,.T.) ;
#2117=FACE_OUTER_BOUND('',#3108,.T.) ;
#2118=FACE_OUTER_BOUND('',#3109,.T.) ;
#2119=FACE_OUTER_BOUND('',#3110,.T.) ;
#2120=FACE_OUTER_BOUND('',#3111,.T.) ;
#2121=FACE_OUTER_BOUND('',#3112,.T.) ;
#2122=FACE_OUTER_BOUND('',#3113,.T.) ;
#2123=FACE_OUTER_BOUND('',#3114,.T.) ;
#2124=FACE_OUTER_BOUND('',#3115,.T.) ;
#2125=FACE_OUTER_BOUND('',#3116,.T.) ;
#2126=FACE_OUTER_BOUND('',#3117,.T.) ;
#2127=FACE_OUTER_BOUND('',#3118,.T.) ;
#2128=FACE_OUTER_BOUND('',#3119,.T.) ;
#2129=FACE_OUTER_BOUND('',#3120,.T.) ;
#2130=FACE_OUTER_BOUND('',#3121,.T.) ;
#2131=FACE_OUTER_BOUND('',#3122,.T.) ;
#2132=FACE_OUTER_BOUND('',#3123,.T.) ;
#2133=FACE_OUTER_BOUND('',#3124,.T.) ;
#2134=FACE_OUTER_BOUND('',#3125,.T.) ;
#2135=FACE_OUTER_BOUND('',#3126,.T.) ;
#2136=FACE_OUTER_BOUND('',#3127,.T.) ;
#2137=FACE_OUTER_BOUND('',#3128,.T.) ;
#2138=FACE_OUTER_BOUND('',#3129,.T.) ;
#2139=FACE_OUTER_BOUND('',#3130,.T.) ;
#2140=FACE_OUTER_BOUND('',#3131,.T.) ;
#2141=FACE_OUTER_BOUND('',#3132,.T.) ;
#2142=FACE_OUTER_BOUND('',#3133,.T.) ;
#2143=FACE_OUTER_BOUND('',#3134,.T.) ;
#2144=FACE_OUTER_BOUND('',#3135,.T.) ;
#2145=FACE_OUTER_BOUND('',#3136,.T.) ;
#2146=FACE_OUTER_BOUND('',#3137,.T.) ;
#2147=FACE_OUTER_BOUND('',#3138,.T.) ;
#2148=FACE_OUTER_BOUND('',#3139,.T.) ;
#2149=FACE_OUTER_BOUND('',#3140,.T.) ;
#2150=FACE_OUTER_BOUND('',#3141,.T.) ;
#2151=FACE_OUTER_BOUND('',#3142,.T.) ;
#2152=FACE_OUTER_BOUND('',#3143,.T.) ;
#2153=FACE_OUTER_BOUND('',#3144,.T.) ;
#2154=FACE_OUTER_BOUND('',#3145,.T.) ;
#2155=FACE_OUTER_BOUND('',#3146,.T.) ;
#2156=FACE_OUTER_BOUND('',#3147,.T.) ;
#2157=FACE_OUTER_BOUND('',#3148,.T.) ;
#2158=FACE_OUTER_BOUND('',#3149,.T.) ;
#2159=FACE_OUTER_BOUND('',#3150,.T.) ;
#2160=FACE_OUTER_BOUND('',#3151,.T.) ;
#2161=FACE_OUTER_BOUND('',#3152,.T.) ;
#2162=FACE_OUTER_BOUND('',#3153,.T.) ;
#2163=FACE_OUTER_BOUND('',#3154,.T.) ;
#2164=FACE_OUTER_BOUND('',#3155,.T.) ;
#2165=FACE_OUTER_BOUND('',#3156,.T.) ;
#2166=FACE_OUTER_BOUND('',#3157,.T.) ;
#2167=FACE_OUTER_BOUND('',#3158,.T.) ;
#2168=FACE_OUTER_BOUND('',#3159,.T.) ;
#2169=FACE_OUTER_BOUND('',#3160,.T.) ;
#2170=FACE_OUTER_BOUND('',#3161,.T.) ;
#2171=FACE_OUTER_BOUND('',#3162,.T.) ;
#2172=FACE_OUTER_BOUND('',#3163,.T.) ;
#2173=FACE_OUTER_BOUND('',#3164,.T.) ;
#2174=FACE_OUTER_BOUND('',#3165,.T.) ;
#2175=FACE_OUTER_BOUND('',#3166,.T.) ;
#2176=FACE_OUTER_BOUND('',#3167,.T.) ;
#2177=FACE_OUTER_BOUND('',#3168,.T.) ;
#2178=FACE_OUTER_BOUND('',#3169,.T.) ;
#2179=FACE_OUTER_BOUND('',#3170,.T.) ;
#2180=FACE_OUTER_BOUND('',#3171,.T.) ;
#2181=FACE_OUTER_BOUND('',#3172,.T.) ;
#2182=FACE_OUTER_BOUND('',#3173,.T.) ;
#2183=FACE_OUTER_BOUND('',#3174,.T.) ;
#2184=FACE_OUTER_BOUND('',#3175,.T.) ;
#2185=FACE_OUTER_BOUND('',#3176,.T.) ;
#2186=FACE_OUTER_BOUND('',#3177,.T.) ;
#2187=FACE_OUTER_BOUND('',#3178,.T.) ;
#2188=FACE_OUTER_BOUND('',#3179,.T.) ;
#2189=FACE_OUTER_BOUND('',#3180,.T.) ;
#2190=FACE_OUTER_BOUND('',#3181,.T.) ;
#2191=FACE_OUTER_BOUND('',#3182,.T.) ;
#2192=FACE_OUTER_BOUND('',#3183,.T.) ;
#2193=FACE_OUTER_BOUND('',#3184,.T.) ;
#2194=FACE_OUTER_BOUND('',#3185,.T.) ;
#2195=FACE_OUTER_BOUND('',#3186,.T.) ;
#2196=FACE_OUTER_BOUND('',#3187,.T.) ;
#2197=FACE_OUTER_BOUND('',#3188,.T.) ;
#2198=FACE_OUTER_BOUND('',#3189,.T.) ;
#2199=FACE_OUTER_BOUND('',#3190,.T.) ;
#2200=FACE_OUTER_BOUND('',#3191,.T.) ;
#2201=FACE_OUTER_BOUND('',#3192,.T.) ;
#2202=FACE_OUTER_BOUND('',#3193,.T.) ;
#2203=FACE_OUTER_BOUND('',#3194,.T.) ;
#2204=FACE_OUTER_BOUND('',#3195,.T.) ;
#2205=FACE_OUTER_BOUND('',#3196,.T.) ;
#2206=FACE_OUTER_BOUND('',#3197,.T.) ;
#2207=FACE_OUTER_BOUND('',#3198,.T.) ;
#2208=FACE_OUTER_BOUND('',#3199,.T.) ;
#2209=FACE_OUTER_BOUND('',#3200,.T.) ;
#2210=FACE_OUTER_BOUND('',#3201,.T.) ;
#2819=EDGE_LOOP('',(#11058,#11059,#11060,#11061)) ;
#2820=EDGE_LOOP('',(#11062,#11063,#11064,#11065)) ;
#2821=EDGE_LOOP('',(#11066,#11067,#11068,#11069)) ;
#2822=EDGE_LOOP('',(#11070)) ;
#2823=EDGE_LOOP('',(#11071,#11072,#11073,#11074)) ;
#2824=EDGE_LOOP('',(#11075,#11076,#11077,#11078)) ;
#2825=EDGE_LOOP('',(#11079,#11080,#11081,#11082)) ;
#2826=EDGE_LOOP('',(#11083,#11084,#11085,#11086)) ;
#2827=EDGE_LOOP('',(#11087,#11088,#11089,#11090)) ;
#2828=EDGE_LOOP('',(#11091,#11092,#11093,#11094)) ;
#2829=EDGE_LOOP('',(#11095,#11096,#11097,#11098)) ;
#2830=EDGE_LOOP('',(#11099,#11100,#11101,#11102)) ;
#2831=EDGE_LOOP('',(#11103,#11104,#11105,#11106)) ;
#2832=EDGE_LOOP('',(#11107,#11108,#11109,#11110)) ;
#2833=EDGE_LOOP('',(#11111,#11112,#11113,#11114)) ;
#2834=EDGE_LOOP('',(#11115,#11116,#11117,#11118)) ;
#2835=EDGE_LOOP('',(#11119,#11120,#11121,#11122)) ;
#2836=EDGE_LOOP('',(#11123,#11124,#11125,#11126)) ;
#2837=EDGE_LOOP('',(#11127,#11128,#11129,#11130)) ;
#2838=EDGE_LOOP('',(#11131,#11132,#11133,#11134)) ;
#2839=EDGE_LOOP('',(#11135,#11136,#11137,#11138)) ;
#2840=EDGE_LOOP('',(#11139,#11140,#11141,#11142)) ;
#2841=EDGE_LOOP('',(#11143,#11144,#11145,#11146)) ;
#2842=EDGE_LOOP('',(#11147,#11148,#11149,#11150)) ;
#2843=EDGE_LOOP('',(#11151,#11152,#11153,#11154)) ;
#2844=EDGE_LOOP('',(#11155,#11156,#11157,#11158)) ;
#2845=EDGE_LOOP('',(#11159,#11160,#11161,#11162)) ;
#2846=EDGE_LOOP('',(#11163,#11164,#11165,#11166)) ;
#2847=EDGE_LOOP('',(#11167,#11168,#11169,#11170)) ;
#2848=EDGE_LOOP('',(#11171,#11172,#11173,#11174)) ;
#2849=EDGE_LOOP('',(#11175,#11176,#11177,#11178)) ;
#2850=EDGE_LOOP('',(#11179,#11180,#11181,#11182)) ;
#2851=EDGE_LOOP('',(#11183,#11184,#11185,#11186)) ;
#2852=EDGE_LOOP('',(#11187,#11188,#11189,#11190)) ;
#2853=EDGE_LOOP('',(#11191,#11192,#11193,#11194)) ;
#2854=EDGE_LOOP('',(#11195,#11196,#11197,#11198)) ;
#2855=EDGE_LOOP('',(#11199,#11200,#11201,#11202)) ;
#2856=EDGE_LOOP('',(#11203,#11204,#11205,#11206)) ;
#2857=EDGE_LOOP('',(#11207,#11208,#11209,#11210)) ;
#2858=EDGE_LOOP('',(#11211,#11212,#11213,#11214)) ;
#2859=EDGE_LOOP('',(#11215,#11216,#11217,#11218)) ;
#2860=EDGE_LOOP('',(#11219,#11220,#11221,#11222)) ;
#2861=EDGE_LOOP('',(#11223,#11224,#11225,#11226)) ;
#2862=EDGE_LOOP('',(#11227,#11228,#11229,#11230)) ;
#2863=EDGE_LOOP('',(#11231,#11232,#11233,#11234)) ;
#2864=EDGE_LOOP('',(#11235,#11236,#11237,#11238)) ;
#2865=EDGE_LOOP('',(#11239,#11240,#11241,#11242)) ;
#2866=EDGE_LOOP('',(#11243,#11244,#11245,#11246)) ;
#2867=EDGE_LOOP('',(#11247,#11248,#11249,#11250)) ;
#2868=EDGE_LOOP('',(#11251,#11252,#11253,#11254)) ;
#2869=EDGE_LOOP('',(#11255,#11256,#11257,#11258)) ;
#2870=EDGE_LOOP('',(#11259,#11260,#11261,#11262)) ;
#2871=EDGE_LOOP('',(#11263,#11264,#11265,#11266)) ;
#2872=EDGE_LOOP('',(#11267,#11268,#11269,#11270)) ;
#2873=EDGE_LOOP('',(#11271,#11272,#11273,#11274)) ;
#2874=EDGE_LOOP('',(#11275,#11276,#11277,#11278)) ;
#2875=EDGE_LOOP('',(#11279,#11280,#11281,#11282)) ;
#2876=EDGE_LOOP('',(#11283,#11284,#11285,#11286)) ;
#2877=EDGE_LOOP('',(#11287,#11288,#11289,#11290)) ;
#2878=EDGE_LOOP('',(#11291,#11292,#11293,#11294)) ;
#2879=EDGE_LOOP('',(#11295,#11296,#11297,#11298)) ;
#2880=EDGE_LOOP('',(#11299,#11300,#11301,#11302)) ;
#2881=EDGE_LOOP('',(#11303,#11304,#11305,#11306)) ;
#2882=EDGE_LOOP('',(#11307,#11308,#11309,#11310)) ;
#2883=EDGE_LOOP('',(#11311,#11312,#11313,#11314)) ;
#2884=EDGE_LOOP('',(#11315,#11316,#11317,#11318)) ;
#2885=EDGE_LOOP('',(#11319)) ;
#2886=EDGE_LOOP('',(#11320)) ;
#2887=EDGE_LOOP('',(#11321,#11322,#11323,#11324,#11325)) ;
#2888=EDGE_LOOP('',(#11326,#11327,#11328,#11329,#11330,#11331)) ;
#2889=EDGE_LOOP('',(#11332,#11333,#11334,#11335,#11336,#11337,#11338,#11339,
#11340,#11341,#11342,#11343,#11344,#11345,#11346,#11347,#11348,#11349,#11350,
#11351,#11352,#11353,#11354,#11355,#11356,#11357,#11358,#11359,#11360,#11361,
#11362,#11363,#11364,#11365,#11366,#11367,#11368,#11369,#11370,#11371,#11372,
#11373,#11374,#11375,#11376,#11377,#11378,#11379,#11380,#11381,#11382,#11383,
#11384,#11385,#11386,#11387,#11388,#11389,#11390,#11391,#11392,#11393,#11394,
#11395,#11396,#11397,#11398,#11399,#11400,#11401,#11402,#11403,#11404,#11405,
#11406,#11407,#11408,#11409,#11410,#11411,#11412,#11413,#11414,#11415,#11416,
#11417,#11418,#11419,#11420,#11421,#11422,#11423,#11424,#11425,#11426,#11427,
#11428,#11429,#11430,#11431,#11432,#11433,#11434,#11435,#11436,#11437,#11438,
#11439,#11440,#11441,#11442,#11443,#11444,#11445,#11446,#11447,#11448,#11449,
#11450,#11451,#11452,#11453,#11454,#11455,#11456)) ;
#2890=EDGE_LOOP('',(#11457,#11458,#11459,#11460,#11461,#11462,#11463,#11464,
#11465,#11466,#11467,#11468,#11469,#11470,#11471,#11472,#11473,#11474,#11475,
#11476,#11477,#11478,#11479,#11480,#11481,#11482,#11483,#11484,#11485,#11486,
#11487,#11488,#11489,#11490,#11491,#11492,#11493,#11494,#11495,#11496,#11497,
#11498,#11499,#11500,#11501,#11502,#11503,#11504,#11505,#11506,#11507,#11508,
#11509,#11510,#11511,#11512,#11513,#11514,#11515,#11516,#11517,#11518,#11519,
#11520,#11521,#11522,#11523,#11524,#11525,#11526,#11527,#11528,#11529,#11530,
#11531,#11532,#11533,#11534,#11535,#11536,#11537,#11538,#11539,#11540,#11541,
#11542,#11543,#11544,#11545,#11546,#11547,#11548,#11549,#11550,#11551,#11552,
#11553,#11554,#11555,#11556,#11557,#11558,#11559,#11560,#11561,#11562,#11563,
#11564,#11565,#11566,#11567,#11568,#11569,#11570,#11571,#11572,#11573,#11574,
#11575,#11576,#11577,#11578,#11579,#11580,#11581)) ;
#2891=EDGE_LOOP('',(#11582,#11583,#11584,#11585,#11586,#11587)) ;
#2892=EDGE_LOOP('',(#11588,#11589,#11590,#11591,#11592)) ;
#2893=EDGE_LOOP('',(#11593)) ;
#2894=EDGE_LOOP('',(#11594)) ;
#2895=EDGE_LOOP('',(#11595,#11596,#11597,#11598)) ;
#2896=EDGE_LOOP('',(#11599)) ;
#2897=EDGE_LOOP('',(#11600)) ;
#2898=EDGE_LOOP('',(#11601,#11602,#11603,#11604)) ;
#2899=EDGE_LOOP('',(#11605)) ;
#2900=EDGE_LOOP('',(#11606,#11607,#11608,#11609)) ;
#2901=EDGE_LOOP('',(#11610,#11611,#11612,#11613)) ;
#2902=EDGE_LOOP('',(#11614,#11615,#11616,#11617)) ;
#2903=EDGE_LOOP('',(#11618,#11619,#11620,#11621)) ;
#2904=EDGE_LOOP('',(#11622,#11623,#11624,#11625)) ;
#2905=EDGE_LOOP('',(#11626,#11627,#11628,#11629)) ;
#2906=EDGE_LOOP('',(#11630,#11631,#11632,#11633)) ;
#2907=EDGE_LOOP('',(#11634,#11635,#11636,#11637)) ;
#2908=EDGE_LOOP('',(#11638,#11639,#11640,#11641)) ;
#2909=EDGE_LOOP('',(#11642,#11643,#11644,#11645)) ;
#2910=EDGE_LOOP('',(#11646,#11647,#11648,#11649)) ;
#2911=EDGE_LOOP('',(#11650,#11651,#11652,#11653)) ;
#2912=EDGE_LOOP('',(#11654,#11655,#11656,#11657)) ;
#2913=EDGE_LOOP('',(#11658,#11659,#11660,#11661)) ;
#2914=EDGE_LOOP('',(#11662,#11663,#11664,#11665)) ;
#2915=EDGE_LOOP('',(#11666,#11667,#11668,#11669)) ;
#2916=EDGE_LOOP('',(#11670,#11671,#11672,#11673)) ;
#2917=EDGE_LOOP('',(#11674,#11675,#11676,#11677)) ;
#2918=EDGE_LOOP('',(#11678,#11679,#11680,#11681)) ;
#2919=EDGE_LOOP('',(#11682,#11683,#11684,#11685)) ;
#2920=EDGE_LOOP('',(#11686,#11687,#11688,#11689)) ;
#2921=EDGE_LOOP('',(#11690,#11691,#11692,#11693)) ;
#2922=EDGE_LOOP('',(#11694,#11695,#11696,#11697)) ;
#2923=EDGE_LOOP('',(#11698,#11699,#11700,#11701)) ;
#2924=EDGE_LOOP('',(#11702,#11703,#11704,#11705)) ;
#2925=EDGE_LOOP('',(#11706,#11707,#11708,#11709)) ;
#2926=EDGE_LOOP('',(#11710,#11711,#11712,#11713)) ;
#2927=EDGE_LOOP('',(#11714,#11715,#11716,#11717)) ;
#2928=EDGE_LOOP('',(#11718,#11719,#11720,#11721)) ;
#2929=EDGE_LOOP('',(#11722,#11723,#11724,#11725)) ;
#2930=EDGE_LOOP('',(#11726,#11727,#11728,#11729)) ;
#2931=EDGE_LOOP('',(#11730,#11731,#11732,#11733)) ;
#2932=EDGE_LOOP('',(#11734,#11735,#11736,#11737)) ;
#2933=EDGE_LOOP('',(#11738,#11739,#11740,#11741)) ;
#2934=EDGE_LOOP('',(#11742,#11743,#11744,#11745)) ;
#2935=EDGE_LOOP('',(#11746,#11747,#11748,#11749)) ;
#2936=EDGE_LOOP('',(#11750,#11751,#11752,#11753)) ;
#2937=EDGE_LOOP('',(#11754,#11755,#11756,#11757)) ;
#2938=EDGE_LOOP('',(#11758,#11759,#11760,#11761)) ;
#2939=EDGE_LOOP('',(#11762,#11763,#11764,#11765)) ;
#2940=EDGE_LOOP('',(#11766,#11767,#11768,#11769)) ;
#2941=EDGE_LOOP('',(#11770,#11771,#11772,#11773)) ;
#2942=EDGE_LOOP('',(#11774,#11775,#11776,#11777)) ;
#2943=EDGE_LOOP('',(#11778,#11779,#11780,#11781)) ;
#2944=EDGE_LOOP('',(#11782,#11783,#11784,#11785)) ;
#2945=EDGE_LOOP('',(#11786,#11787,#11788,#11789)) ;
#2946=EDGE_LOOP('',(#11790,#11791,#11792,#11793)) ;
#2947=EDGE_LOOP('',(#11794,#11795,#11796,#11797)) ;
#2948=EDGE_LOOP('',(#11798,#11799,#11800,#11801)) ;
#2949=EDGE_LOOP('',(#11802,#11803,#11804,#11805)) ;
#2950=EDGE_LOOP('',(#11806,#11807,#11808,#11809)) ;
#2951=EDGE_LOOP('',(#11810,#11811,#11812,#11813)) ;
#2952=EDGE_LOOP('',(#11814,#11815,#11816,#11817)) ;
#2953=EDGE_LOOP('',(#11818,#11819,#11820,#11821)) ;
#2954=EDGE_LOOP('',(#11822,#11823,#11824,#11825)) ;
#2955=EDGE_LOOP('',(#11826,#11827,#11828,#11829)) ;
#2956=EDGE_LOOP('',(#11830,#11831,#11832,#11833)) ;
#2957=EDGE_LOOP('',(#11834,#11835,#11836,#11837)) ;
#2958=EDGE_LOOP('',(#11838,#11839,#11840,#11841)) ;
#2959=EDGE_LOOP('',(#11842,#11843,#11844,#11845)) ;
#2960=EDGE_LOOP('',(#11846,#11847,#11848,#11849)) ;
#2961=EDGE_LOOP('',(#11850,#11851,#11852,#11853)) ;
#2962=EDGE_LOOP('',(#11854,#11855,#11856,#11857)) ;
#2963=EDGE_LOOP('',(#11858,#11859,#11860,#11861)) ;
#2964=EDGE_LOOP('',(#11862,#11863,#11864,#11865)) ;
#2965=EDGE_LOOP('',(#11866,#11867,#11868,#11869)) ;
#2966=EDGE_LOOP('',(#11870,#11871,#11872,#11873)) ;
#2967=EDGE_LOOP('',(#11874,#11875,#11876,#11877)) ;
#2968=EDGE_LOOP('',(#11878,#11879,#11880,#11881)) ;
#2969=EDGE_LOOP('',(#11882,#11883,#11884,#11885)) ;
#2970=EDGE_LOOP('',(#11886,#11887,#11888,#11889)) ;
#2971=EDGE_LOOP('',(#11890,#11891,#11892,#11893)) ;
#2972=EDGE_LOOP('',(#11894,#11895,#11896,#11897)) ;
#2973=EDGE_LOOP('',(#11898,#11899,#11900,#11901)) ;
#2974=EDGE_LOOP('',(#11902,#11903,#11904,#11905)) ;
#2975=EDGE_LOOP('',(#11906,#11907,#11908,#11909)) ;
#2976=EDGE_LOOP('',(#11910,#11911,#11912,#11913)) ;
#2977=EDGE_LOOP('',(#11914,#11915,#11916,#11917)) ;
#2978=EDGE_LOOP('',(#11918,#11919,#11920,#11921)) ;
#2979=EDGE_LOOP('',(#11922,#11923,#11924,#11925)) ;
#2980=EDGE_LOOP('',(#11926,#11927,#11928,#11929)) ;
#2981=EDGE_LOOP('',(#11930,#11931,#11932,#11933,#11934)) ;
#2982=EDGE_LOOP('',(#11935,#11936,#11937,#11938)) ;
#2983=EDGE_LOOP('',(#11939,#11940,#11941,#11942)) ;
#2984=EDGE_LOOP('',(#11943,#11944,#11945,#11946)) ;
#2985=EDGE_LOOP('',(#11947,#11948,#11949,#11950)) ;
#2986=EDGE_LOOP('',(#11951,#11952,#11953,#11954)) ;
#2987=EDGE_LOOP('',(#11955,#11956,#11957,#11958)) ;
#2988=EDGE_LOOP('',(#11959,#11960,#11961,#11962)) ;
#2989=EDGE_LOOP('',(#11963,#11964,#11965,#11966)) ;
#2990=EDGE_LOOP('',(#11967,#11968,#11969,#11970)) ;
#2991=EDGE_LOOP('',(#11971,#11972,#11973,#11974)) ;
#2992=EDGE_LOOP('',(#11975,#11976,#11977,#11978)) ;
#2993=EDGE_LOOP('',(#11979,#11980,#11981,#11982)) ;
#2994=EDGE_LOOP('',(#11983,#11984,#11985,#11986)) ;
#2995=EDGE_LOOP('',(#11987,#11988,#11989,#11990)) ;
#2996=EDGE_LOOP('',(#11991,#11992,#11993,#11994)) ;
#2997=EDGE_LOOP('',(#11995,#11996,#11997,#11998)) ;
#2998=EDGE_LOOP('',(#11999,#12000,#12001,#12002)) ;
#2999=EDGE_LOOP('',(#12003,#12004,#12005,#12006)) ;
#3000=EDGE_LOOP('',(#12007,#12008,#12009,#12010)) ;
#3001=EDGE_LOOP('',(#12011,#12012,#12013,#12014)) ;
#3002=EDGE_LOOP('',(#12015,#12016,#12017,#12018)) ;
#3003=EDGE_LOOP('',(#12019,#12020,#12021,#12022)) ;
#3004=EDGE_LOOP('',(#12023,#12024,#12025,#12026)) ;
#3005=EDGE_LOOP('',(#12027,#12028,#12029,#12030)) ;
#3006=EDGE_LOOP('',(#12031,#12032,#12033,#12034)) ;
#3007=EDGE_LOOP('',(#12035,#12036,#12037,#12038)) ;
#3008=EDGE_LOOP('',(#12039,#12040,#12041,#12042)) ;
#3009=EDGE_LOOP('',(#12043,#12044,#12045,#12046)) ;
#3010=EDGE_LOOP('',(#12047,#12048,#12049,#12050)) ;
#3011=EDGE_LOOP('',(#12051,#12052,#12053,#12054)) ;
#3012=EDGE_LOOP('',(#12055,#12056,#12057,#12058)) ;
#3013=EDGE_LOOP('',(#12059,#12060,#12061,#12062)) ;
#3014=EDGE_LOOP('',(#12063,#12064,#12065,#12066)) ;
#3015=EDGE_LOOP('',(#12067,#12068,#12069,#12070)) ;
#3016=EDGE_LOOP('',(#12071,#12072,#12073,#12074)) ;
#3017=EDGE_LOOP('',(#12075,#12076,#12077,#12078)) ;
#3018=EDGE_LOOP('',(#12079,#12080,#12081,#12082)) ;
#3019=EDGE_LOOP('',(#12083,#12084,#12085,#12086)) ;
#3020=EDGE_LOOP('',(#12087,#12088,#12089,#12090)) ;
#3021=EDGE_LOOP('',(#12091,#12092,#12093,#12094)) ;
#3022=EDGE_LOOP('',(#12095,#12096,#12097,#12098)) ;
#3023=EDGE_LOOP('',(#12099,#12100,#12101,#12102)) ;
#3024=EDGE_LOOP('',(#12103,#12104,#12105,#12106)) ;
#3025=EDGE_LOOP('',(#12107,#12108,#12109,#12110)) ;
#3026=EDGE_LOOP('',(#12111,#12112,#12113,#12114)) ;
#3027=EDGE_LOOP('',(#12115,#12116,#12117,#12118)) ;
#3028=EDGE_LOOP('',(#12119,#12120,#12121,#12122)) ;
#3029=EDGE_LOOP('',(#12123,#12124,#12125,#12126)) ;
#3030=EDGE_LOOP('',(#12127,#12128,#12129,#12130)) ;
#3031=EDGE_LOOP('',(#12131,#12132,#12133,#12134)) ;
#3032=EDGE_LOOP('',(#12135,#12136,#12137,#12138)) ;
#3033=EDGE_LOOP('',(#12139,#12140,#12141,#12142)) ;
#3034=EDGE_LOOP('',(#12143,#12144,#12145,#12146)) ;
#3035=EDGE_LOOP('',(#12147,#12148,#12149,#12150)) ;
#3036=EDGE_LOOP('',(#12151,#12152,#12153,#12154)) ;
#3037=EDGE_LOOP('',(#12155,#12156,#12157,#12158)) ;
#3038=EDGE_LOOP('',(#12159,#12160,#12161,#12162)) ;
#3039=EDGE_LOOP('',(#12163,#12164,#12165,#12166)) ;
#3040=EDGE_LOOP('',(#12167,#12168,#12169,#12170)) ;
#3041=EDGE_LOOP('',(#12171,#12172,#12173,#12174)) ;
#3042=EDGE_LOOP('',(#12175,#12176,#12177,#12178)) ;
#3043=EDGE_LOOP('',(#12179,#12180,#12181,#12182)) ;
#3044=EDGE_LOOP('',(#12183,#12184,#12185,#12186)) ;
#3045=EDGE_LOOP('',(#12187,#12188,#12189,#12190)) ;
#3046=EDGE_LOOP('',(#12191,#12192,#12193,#12194)) ;
#3047=EDGE_LOOP('',(#12195,#12196,#12197,#12198)) ;
#3048=EDGE_LOOP('',(#12199,#12200,#12201,#12202)) ;
#3049=EDGE_LOOP('',(#12203,#12204,#12205,#12206)) ;
#3050=EDGE_LOOP('',(#12207,#12208,#12209,#12210)) ;
#3051=EDGE_LOOP('',(#12211,#12212,#12213,#12214)) ;
#3052=EDGE_LOOP('',(#12215,#12216,#12217,#12218)) ;
#3053=EDGE_LOOP('',(#12219,#12220,#12221,#12222)) ;
#3054=EDGE_LOOP('',(#12223,#12224,#12225,#12226)) ;
#3055=EDGE_LOOP('',(#12227,#12228,#12229,#12230)) ;
#3056=EDGE_LOOP('',(#12231,#12232,#12233,#12234)) ;
#3057=EDGE_LOOP('',(#12235,#12236,#12237,#12238)) ;
#3058=EDGE_LOOP('',(#12239,#12240,#12241,#12242)) ;
#3059=EDGE_LOOP('',(#12243,#12244,#12245,#12246)) ;
#3060=EDGE_LOOP('',(#12247,#12248,#12249,#12250)) ;
#3061=EDGE_LOOP('',(#12251,#12252,#12253,#12254)) ;
#3062=EDGE_LOOP('',(#12255,#12256,#12257,#12258)) ;
#3063=EDGE_LOOP('',(#12259,#12260,#12261,#12262)) ;
#3064=EDGE_LOOP('',(#12263,#12264,#12265,#12266)) ;
#3065=EDGE_LOOP('',(#12267,#12268,#12269,#12270)) ;
#3066=EDGE_LOOP('',(#12271,#12272,#12273,#12274)) ;
#3067=EDGE_LOOP('',(#12275,#12276,#12277,#12278)) ;
#3068=EDGE_LOOP('',(#12279,#12280,#12281,#12282)) ;
#3069=EDGE_LOOP('',(#12283,#12284,#12285,#12286)) ;
#3070=EDGE_LOOP('',(#12287,#12288,#12289,#12290)) ;
#3071=EDGE_LOOP('',(#12291,#12292,#12293,#12294)) ;
#3072=EDGE_LOOP('',(#12295,#12296,#12297,#12298)) ;
#3073=EDGE_LOOP('',(#12299,#12300,#12301,#12302)) ;
#3074=EDGE_LOOP('',(#12303,#12304,#12305,#12306)) ;
#3075=EDGE_LOOP('',(#12307,#12308,#12309,#12310)) ;
#3076=EDGE_LOOP('',(#12311,#12312,#12313,#12314)) ;
#3077=EDGE_LOOP('',(#12315,#12316,#12317,#12318)) ;
#3078=EDGE_LOOP('',(#12319,#12320,#12321,#12322)) ;
#3079=EDGE_LOOP('',(#12323,#12324,#12325,#12326)) ;
#3080=EDGE_LOOP('',(#12327,#12328,#12329,#12330)) ;
#3081=EDGE_LOOP('',(#12331,#12332,#12333,#12334)) ;
#3082=EDGE_LOOP('',(#12335,#12336,#12337,#12338)) ;
#3083=EDGE_LOOP('',(#12339,#12340,#12341,#12342)) ;
#3084=EDGE_LOOP('',(#12343,#12344,#12345,#12346)) ;
#3085=EDGE_LOOP('',(#12347,#12348,#12349,#12350)) ;
#3086=EDGE_LOOP('',(#12351,#12352,#12353,#12354)) ;
#3087=EDGE_LOOP('',(#12355,#12356,#12357,#12358)) ;
#3088=EDGE_LOOP('',(#12359,#12360,#12361,#12362)) ;
#3089=EDGE_LOOP('',(#12363,#12364,#12365,#12366)) ;
#3090=EDGE_LOOP('',(#12367,#12368,#12369,#12370)) ;
#3091=EDGE_LOOP('',(#12371,#12372,#12373,#12374)) ;
#3092=EDGE_LOOP('',(#12375,#12376,#12377,#12378)) ;
#3093=EDGE_LOOP('',(#12379,#12380,#12381,#12382)) ;
#3094=EDGE_LOOP('',(#12383,#12384,#12385,#12386)) ;
#3095=EDGE_LOOP('',(#12387,#12388,#12389,#12390)) ;
#3096=EDGE_LOOP('',(#12391,#12392,#12393,#12394)) ;
#3097=EDGE_LOOP('',(#12395,#12396,#12397,#12398)) ;
#3098=EDGE_LOOP('',(#12399,#12400,#12401,#12402)) ;
#3099=EDGE_LOOP('',(#12403,#12404,#12405,#12406)) ;
#3100=EDGE_LOOP('',(#12407,#12408,#12409,#12410)) ;
#3101=EDGE_LOOP('',(#12411,#12412,#12413,#12414)) ;
#3102=EDGE_LOOP('',(#12415,#12416,#12417,#12418)) ;
#3103=EDGE_LOOP('',(#12419,#12420,#12421,#12422)) ;
#3104=EDGE_LOOP('',(#12423,#12424,#12425,#12426)) ;
#3105=EDGE_LOOP('',(#12427,#12428,#12429,#12430)) ;
#3106=EDGE_LOOP('',(#12431,#12432,#12433,#12434)) ;
#3107=EDGE_LOOP('',(#12435,#12436,#12437,#12438)) ;
#3108=EDGE_LOOP('',(#12439,#12440,#12441,#12442)) ;
#3109=EDGE_LOOP('',(#12443,#12444,#12445,#12446)) ;
#3110=EDGE_LOOP('',(#12447,#12448,#12449,#12450)) ;
#3111=EDGE_LOOP('',(#12451,#12452,#12453,#12454)) ;
#3112=EDGE_LOOP('',(#12455,#12456,#12457,#12458)) ;
#3113=EDGE_LOOP('',(#12459,#12460,#12461,#12462)) ;
#3114=EDGE_LOOP('',(#12463,#12464,#12465,#12466)) ;
#3115=EDGE_LOOP('',(#12467,#12468,#12469,#12470)) ;
#3116=EDGE_LOOP('',(#12471,#12472,#12473,#12474)) ;
#3117=EDGE_LOOP('',(#12475,#12476,#12477,#12478)) ;
#3118=EDGE_LOOP('',(#12479,#12480,#12481,#12482)) ;
#3119=EDGE_LOOP('',(#12483,#12484,#12485,#12486)) ;
#3120=EDGE_LOOP('',(#12487,#12488,#12489,#12490)) ;
#3121=EDGE_LOOP('',(#12491,#12492,#12493,#12494)) ;
#3122=EDGE_LOOP('',(#12495,#12496,#12497,#12498)) ;
#3123=EDGE_LOOP('',(#12499,#12500,#12501,#12502)) ;
#3124=EDGE_LOOP('',(#12503,#12504,#12505,#12506)) ;
#3125=EDGE_LOOP('',(#12507,#12508,#12509,#12510)) ;
#3126=EDGE_LOOP('',(#12511,#12512,#12513,#12514)) ;
#3127=EDGE_LOOP('',(#12515,#12516,#12517,#12518)) ;
#3128=EDGE_LOOP('',(#12519,#12520,#12521,#12522)) ;
#3129=EDGE_LOOP('',(#12523,#12524,#12525,#12526)) ;
#3130=EDGE_LOOP('',(#12527,#12528,#12529,#12530)) ;
#3131=EDGE_LOOP('',(#12531,#12532,#12533,#12534)) ;
#3132=EDGE_LOOP('',(#12535,#12536,#12537,#12538,#12539)) ;
#3133=EDGE_LOOP('',(#12540,#12541,#12542,#12543)) ;
#3134=EDGE_LOOP('',(#12544,#12545,#12546,#12547)) ;
#3135=EDGE_LOOP('',(#12548,#12549,#12550,#12551)) ;
#3136=EDGE_LOOP('',(#12552,#12553,#12554,#12555)) ;
#3137=EDGE_LOOP('',(#12556,#12557,#12558,#12559)) ;
#3138=EDGE_LOOP('',(#12560,#12561,#12562,#12563)) ;
#3139=EDGE_LOOP('',(#12564,#12565,#12566,#12567)) ;
#3140=EDGE_LOOP('',(#12568,#12569,#12570,#12571)) ;
#3141=EDGE_LOOP('',(#12572,#12573,#12574,#12575)) ;
#3142=EDGE_LOOP('',(#12576,#12577,#12578,#12579)) ;
#3143=EDGE_LOOP('',(#12580,#12581,#12582,#12583)) ;
#3144=EDGE_LOOP('',(#12584,#12585,#12586,#12587)) ;
#3145=EDGE_LOOP('',(#12588,#12589,#12590,#12591)) ;
#3146=EDGE_LOOP('',(#12592,#12593,#12594,#12595)) ;
#3147=EDGE_LOOP('',(#12596,#12597,#12598,#12599)) ;
#3148=EDGE_LOOP('',(#12600,#12601,#12602,#12603)) ;
#3149=EDGE_LOOP('',(#12604,#12605,#12606,#12607)) ;
#3150=EDGE_LOOP('',(#12608,#12609,#12610,#12611)) ;
#3151=EDGE_LOOP('',(#12612,#12613,#12614,#12615)) ;
#3152=EDGE_LOOP('',(#12616,#12617,#12618,#12619)) ;
#3153=EDGE_LOOP('',(#12620,#12621,#12622,#12623)) ;
#3154=EDGE_LOOP('',(#12624,#12625,#12626,#12627)) ;
#3155=EDGE_LOOP('',(#12628,#12629,#12630,#12631)) ;
#3156=EDGE_LOOP('',(#12632,#12633,#12634,#12635)) ;
#3157=EDGE_LOOP('',(#12636,#12637,#12638,#12639)) ;
#3158=EDGE_LOOP('',(#12640,#12641,#12642,#12643)) ;
#3159=EDGE_LOOP('',(#12644,#12645,#12646,#12647)) ;
#3160=EDGE_LOOP('',(#12648,#12649,#12650,#12651)) ;
#3161=EDGE_LOOP('',(#12652,#12653,#12654,#12655)) ;
#3162=EDGE_LOOP('',(#12656,#12657,#12658,#12659)) ;
#3163=EDGE_LOOP('',(#12660,#12661,#12662,#12663)) ;
#3164=EDGE_LOOP('',(#12664,#12665,#12666,#12667)) ;
#3165=EDGE_LOOP('',(#12668,#12669,#12670,#12671)) ;
#3166=EDGE_LOOP('',(#12672,#12673,#12674,#12675)) ;
#3167=EDGE_LOOP('',(#12676,#12677,#12678,#12679)) ;
#3168=EDGE_LOOP('',(#12680,#12681,#12682,#12683)) ;
#3169=EDGE_LOOP('',(#12684,#12685,#12686,#12687)) ;
#3170=EDGE_LOOP('',(#12688,#12689,#12690,#12691)) ;
#3171=EDGE_LOOP('',(#12692,#12693,#12694,#12695)) ;
#3172=EDGE_LOOP('',(#12696,#12697,#12698,#12699)) ;
#3173=EDGE_LOOP('',(#12700,#12701,#12702,#12703)) ;
#3174=EDGE_LOOP('',(#12704,#12705,#12706,#12707)) ;
#3175=EDGE_LOOP('',(#12708,#12709,#12710,#12711)) ;
#3176=EDGE_LOOP('',(#12712,#12713,#12714,#12715)) ;
#3177=EDGE_LOOP('',(#12716,#12717,#12718,#12719)) ;
#3178=EDGE_LOOP('',(#12720,#12721,#12722,#12723)) ;
#3179=EDGE_LOOP('',(#12724,#12725,#12726,#12727)) ;
#3180=EDGE_LOOP('',(#12728,#12729,#12730,#12731)) ;
#3181=EDGE_LOOP('',(#12732,#12733,#12734,#12735)) ;
#3182=EDGE_LOOP('',(#12736,#12737,#12738,#12739)) ;
#3183=EDGE_LOOP('',(#12740,#12741,#12742,#12743)) ;
#3184=EDGE_LOOP('',(#12744,#12745,#12746,#12747)) ;
#3185=EDGE_LOOP('',(#12748,#12749,#12750,#12751)) ;
#3186=EDGE_LOOP('',(#12752,#12753,#12754,#12755)) ;
#3187=EDGE_LOOP('',(#12756,#12757,#12758,#12759)) ;
#3188=EDGE_LOOP('',(#12760,#12761,#12762,#12763)) ;
#3189=EDGE_LOOP('',(#12764,#12765,#12766,#12767)) ;
#3190=EDGE_LOOP('',(#12768,#12769,#12770,#12771)) ;
#3191=EDGE_LOOP('',(#12772,#12773,#12774,#12775)) ;
#3192=EDGE_LOOP('',(#12776,#12777,#12778,#12779)) ;
#3193=EDGE_LOOP('',(#12780,#12781,#12782,#12783)) ;
#3194=EDGE_LOOP('',(#12784,#12785,#12786,#12787)) ;
#3195=EDGE_LOOP('',(#12788,#12789,#12790,#12791)) ;
#3196=EDGE_LOOP('',(#12792,#12793,#12794,#12795)) ;
#3197=EDGE_LOOP('',(#12796,#12797,#12798,#12799)) ;
#3198=EDGE_LOOP('',(#12800,#12801,#12802,#12803)) ;
#3199=EDGE_LOOP('',(#12804,#12805,#12806,#12807)) ;
#3200=EDGE_LOOP('',(#12808,#12809,#12810,#12811)) ;
#3201=EDGE_LOOP('',(#12812,#12813,#12814,#12815)) ;
#3709=CIRCLE('',#16213,40.) ;
#3710=CIRCLE('',#16214,20.) ;
#3711=CIRCLE('',#16216,47.175) ;
#3712=CIRCLE('',#16217,47.175) ;
#3713=CIRCLE('',#16219,47.175) ;
#3714=CIRCLE('',#16220,47.175) ;
#3715=CIRCLE('',#16222,47.175) ;
#3716=CIRCLE('',#16223,47.175) ;
#3717=CIRCLE('',#16225,47.175) ;
#3718=CIRCLE('',#16226,47.175) ;
#3719=CIRCLE('',#16228,47.175) ;
#3720=CIRCLE('',#16229,47.175) ;
#3721=CIRCLE('',#16231,47.175) ;
#3722=CIRCLE('',#16232,47.175) ;
#3723=CIRCLE('',#16234,47.175) ;
#3724=CIRCLE('',#16235,47.175) ;
#3725=CIRCLE('',#16237,47.175) ;
#3726=CIRCLE('',#16238,47.175) ;
#3727=CIRCLE('',#16240,47.175) ;
#3728=CIRCLE('',#16241,47.175) ;
#3729=CIRCLE('',#16243,47.175) ;
#3730=CIRCLE('',#16244,47.175) ;
#3731=CIRCLE('',#16246,47.175) ;
#3732=CIRCLE('',#16247,47.175) ;
#3733=CIRCLE('',#16249,47.175) ;
#3734=CIRCLE('',#16250,47.175) ;
#3735=CIRCLE('',#16252,47.175) ;
#3736=CIRCLE('',#16253,47.175) ;
#3737=CIRCLE('',#16255,47.175) ;
#3738=CIRCLE('',#16256,47.175) ;
#3739=CIRCLE('',#16258,47.175) ;
#3740=CIRCLE('',#16259,47.175) ;
#3741=CIRCLE('',#16261,47.175) ;
#3742=CIRCLE('',#16262,47.175) ;
#3743=CIRCLE('',#16264,47.175) ;
#3744=CIRCLE('',#16265,47.175) ;
#3745=CIRCLE('',#16267,47.175) ;
#3746=CIRCLE('',#16268,47.175) ;
#3747=CIRCLE('',#16270,47.175) ;
#3748=CIRCLE('',#16271,47.175) ;
#3749=CIRCLE('',#16273,47.175) ;
#3750=CIRCLE('',#16274,47.175) ;
#3751=CIRCLE('',#16276,47.175) ;
#3752=CIRCLE('',#16277,47.175) ;
#3753=CIRCLE('',#16279,47.175) ;
#3754=CIRCLE('',#16280,47.175) ;
#3755=CIRCLE('',#16282,47.175) ;
#3756=CIRCLE('',#16283,47.175) ;
#3757=CIRCLE('',#16285,47.175) ;
#3758=CIRCLE('',#16286,47.175) ;
#3759=CIRCLE('',#16288,47.175) ;
#3760=CIRCLE('',#16289,47.175) ;
#3761=CIRCLE('',#16291,47.175) ;
#3762=CIRCLE('',#16292,47.175) ;
#3763=CIRCLE('',#16294,47.175) ;
#3764=CIRCLE('',#16295,47.175) ;
#3765=CIRCLE('',#16297,47.175) ;
#3766=CIRCLE('',#16298,47.175) ;
#3767=CIRCLE('',#16300,47.175) ;
#3768=CIRCLE('',#16301,47.175) ;
#3769=CIRCLE('',#16303,47.175) ;
#3770=CIRCLE('',#16304,47.175) ;
#3771=CIRCLE('',#16306,47.175) ;
#3772=CIRCLE('',#16307,47.175) ;
#3773=CIRCLE('',#16309,47.175) ;
#3774=CIRCLE('',#16310,47.175) ;
#3775=CIRCLE('',#16312,47.175) ;
#3776=CIRCLE('',#16313,47.175) ;
#3777=CIRCLE('',#16315,47.175) ;
#3778=CIRCLE('',#16316,47.175) ;
#3779=CIRCLE('',#16318,47.175) ;
#3780=CIRCLE('',#16319,47.175) ;
#3781=CIRCLE('',#16321,47.175) ;
#3782=CIRCLE('',#16322,47.175) ;
#3783=CIRCLE('',#16324,47.175) ;
#3784=CIRCLE('',#16325,47.175) ;
#3785=CIRCLE('',#16327,47.175) ;
#3786=CIRCLE('',#16328,47.175) ;
#3787=CIRCLE('',#16330,47.175) ;
#3788=CIRCLE('',#16331,47.175) ;
#3789=CIRCLE('',#16333,47.175) ;
#3790=CIRCLE('',#16334,47.175) ;
#3791=CIRCLE('',#16336,47.175) ;
#3792=CIRCLE('',#16337,47.175) ;
#3793=CIRCLE('',#16339,47.175) ;
#3794=CIRCLE('',#16340,47.175) ;
#3795=CIRCLE('',#16342,47.175) ;
#3796=CIRCLE('',#16343,47.175) ;
#3797=CIRCLE('',#16345,47.175) ;
#3798=CIRCLE('',#16346,47.175) ;
#3799=CIRCLE('',#16348,47.175) ;
#3800=CIRCLE('',#16349,47.175) ;
#3801=CIRCLE('',#16351,47.175) ;
#3802=CIRCLE('',#16352,47.175) ;
#3803=CIRCLE('',#16354,47.175) ;
#3804=CIRCLE('',#16355,47.175) ;
#3805=CIRCLE('',#16357,47.175) ;
#3806=CIRCLE('',#16358,47.175) ;
#3807=CIRCLE('',#16360,47.175) ;
#3808=CIRCLE('',#16361,47.175) ;
#3809=CIRCLE('',#16363,47.175) ;
#3810=CIRCLE('',#16364,47.175) ;
#3811=CIRCLE('',#16366,47.175) ;
#3812=CIRCLE('',#16367,47.175) ;
#3813=CIRCLE('',#16369,47.175) ;
#3814=CIRCLE('',#16370,47.175) ;
#3815=CIRCLE('',#16372,47.175) ;
#3816=CIRCLE('',#16373,47.175) ;
#3817=CIRCLE('',#16375,47.175) ;
#3818=CIRCLE('',#16376,47.175) ;
#3819=CIRCLE('',#16378,47.175) ;
#3820=CIRCLE('',#16379,47.175) ;
#3821=CIRCLE('',#16381,47.175) ;
#3822=CIRCLE('',#16382,47.175) ;
#3823=CIRCLE('',#16384,47.175) ;
#3824=CIRCLE('',#16385,47.175) ;
#3825=CIRCLE('',#16387,47.175) ;
#3826=CIRCLE('',#16388,47.175) ;
#3827=CIRCLE('',#16390,47.175) ;
#3828=CIRCLE('',#16391,47.175) ;
#3829=CIRCLE('',#16393,47.175) ;
#3830=CIRCLE('',#16394,47.175) ;
#3831=CIRCLE('',#16396,40.) ;
#3832=CIRCLE('',#16398,47.0433475024125) ;
#3833=CIRCLE('',#16400,49.2411809548974) ;
#3834=CIRCLE('',#16401,49.2411809548974) ;
#3835=CIRCLE('',#16403,49.5) ;
#3836=CIRCLE('',#16404,49.5) ;
#3837=CIRCLE('',#16406,47.175) ;
#3838=CIRCLE('',#16407,47.175) ;
#3839=CIRCLE('',#16408,47.175) ;
#3840=CIRCLE('',#16409,47.175) ;
#3841=CIRCLE('',#16410,47.175) ;
#3842=CIRCLE('',#16411,47.175) ;
#3843=CIRCLE('',#16412,47.175) ;
#3844=CIRCLE('',#16413,47.175) ;
#3845=CIRCLE('',#16414,47.175) ;
#3846=CIRCLE('',#16415,47.175) ;
#3847=CIRCLE('',#16416,47.175) ;
#3848=CIRCLE('',#16417,47.175) ;
#3849=CIRCLE('',#16418,47.175) ;
#3850=CIRCLE('',#16419,47.175) ;
#3851=CIRCLE('',#16420,47.175) ;
#3852=CIRCLE('',#16421,47.175) ;
#3853=CIRCLE('',#16422,47.175) ;
#3854=CIRCLE('',#16423,47.175) ;
#3855=CIRCLE('',#16424,47.175) ;
#3856=CIRCLE('',#16425,47.175) ;
#3857=CIRCLE('',#16426,47.175) ;
#3858=CIRCLE('',#16427,47.175) ;
#3859=CIRCLE('',#16428,47.175) ;
#3860=CIRCLE('',#16429,47.175) ;
#3861=CIRCLE('',#16430,47.175) ;
#3862=CIRCLE('',#16431,47.175) ;
#3863=CIRCLE('',#16432,47.175) ;
#3864=CIRCLE('',#16433,47.175) ;
#3865=CIRCLE('',#16434,47.175) ;
#3866=CIRCLE('',#16435,47.175) ;
#3867=CIRCLE('',#16436,47.175) ;
#3868=CIRCLE('',#16437,47.175) ;
#3869=CIRCLE('',#16438,47.175) ;
#3870=CIRCLE('',#16439,47.175) ;
#3871=CIRCLE('',#16440,47.175) ;
#3872=CIRCLE('',#16441,47.175) ;
#3873=CIRCLE('',#16442,47.175) ;
#3874=CIRCLE('',#16443,47.175) ;
#3875=CIRCLE('',#16444,47.175) ;
#3876=CIRCLE('',#16445,47.175) ;
#3877=CIRCLE('',#16446,47.175) ;
#3878=CIRCLE('',#16447,47.175) ;
#3879=CIRCLE('',#16448,47.175) ;
#3880=CIRCLE('',#16449,47.175) ;
#3881=CIRCLE('',#16450,47.175) ;
#3882=CIRCLE('',#16451,47.175) ;
#3883=CIRCLE('',#16452,47.175) ;
#3884=CIRCLE('',#16453,47.175) ;
#3885=CIRCLE('',#16454,47.175) ;
#3886=CIRCLE('',#16455,47.175) ;
#3887=CIRCLE('',#16456,47.175) ;
#3888=CIRCLE('',#16457,47.175) ;
#3889=CIRCLE('',#16458,47.175) ;
#3890=CIRCLE('',#16459,47.175) ;
#3891=CIRCLE('',#16460,47.175) ;
#3892=CIRCLE('',#16461,47.175) ;
#3893=CIRCLE('',#16462,47.175) ;
#3894=CIRCLE('',#16463,47.175) ;
#3895=CIRCLE('',#16464,47.175) ;
#3896=CIRCLE('',#16465,47.175) ;
#3897=CIRCLE('',#16466,47.175) ;
#3898=CIRCLE('',#16468,49.5) ;
#3899=CIRCLE('',#16469,49.5) ;
#3900=CIRCLE('',#16470,47.175) ;
#3901=CIRCLE('',#16471,47.175) ;
#3902=CIRCLE('',#16472,47.175) ;
#3903=CIRCLE('',#16473,47.175) ;
#3904=CIRCLE('',#16474,47.175) ;
#3905=CIRCLE('',#16475,47.175) ;
#3906=CIRCLE('',#16476,47.175) ;
#3907=CIRCLE('',#16477,47.175) ;
#3908=CIRCLE('',#16478,47.175) ;
#3909=CIRCLE('',#16479,47.175) ;
#3910=CIRCLE('',#16480,47.175) ;
#3911=CIRCLE('',#16481,47.175) ;
#3912=CIRCLE('',#16482,47.175) ;
#3913=CIRCLE('',#16483,47.175) ;
#3914=CIRCLE('',#16484,47.175) ;
#3915=CIRCLE('',#16485,47.175) ;
#3916=CIRCLE('',#16486,47.175) ;
#3917=CIRCLE('',#16487,47.175) ;
#3918=CIRCLE('',#16488,47.175) ;
#3919=CIRCLE('',#16489,47.175) ;
#3920=CIRCLE('',#16490,47.175) ;
#3921=CIRCLE('',#16491,47.175) ;
#3922=CIRCLE('',#16492,47.175) ;
#3923=CIRCLE('',#16493,47.175) ;
#3924=CIRCLE('',#16494,47.175) ;
#3925=CIRCLE('',#16495,47.175) ;
#3926=CIRCLE('',#16496,47.175) ;
#3927=CIRCLE('',#16497,47.175) ;
#3928=CIRCLE('',#16498,47.175) ;
#3929=CIRCLE('',#16499,47.175) ;
#3930=CIRCLE('',#16500,47.175) ;
#3931=CIRCLE('',#16501,47.175) ;
#3932=CIRCLE('',#16502,47.175) ;
#3933=CIRCLE('',#16503,47.175) ;
#3934=CIRCLE('',#16504,47.175) ;
#3935=CIRCLE('',#16505,47.175) ;
#3936=CIRCLE('',#16506,47.175) ;
#3937=CIRCLE('',#16507,47.175) ;
#3938=CIRCLE('',#16508,47.175) ;
#3939=CIRCLE('',#16509,47.175) ;
#3940=CIRCLE('',#16510,47.175) ;
#3941=CIRCLE('',#16511,47.175) ;
#3942=CIRCLE('',#16512,47.175) ;
#3943=CIRCLE('',#16513,47.175) ;
#3944=CIRCLE('',#16514,47.175) ;
#3945=CIRCLE('',#16515,47.175) ;
#3946=CIRCLE('',#16516,47.175) ;
#3947=CIRCLE('',#16517,47.175) ;
#3948=CIRCLE('',#16518,47.175) ;
#3949=CIRCLE('',#16519,47.175) ;
#3950=CIRCLE('',#16520,47.175) ;
#3951=CIRCLE('',#16521,47.175) ;
#3952=CIRCLE('',#16522,47.175) ;
#3953=CIRCLE('',#16523,47.175) ;
#3954=CIRCLE('',#16524,47.175) ;
#3955=CIRCLE('',#16525,47.175) ;
#3956=CIRCLE('',#16526,47.175) ;
#3957=CIRCLE('',#16527,47.175) ;
#3958=CIRCLE('',#16528,47.175) ;
#3959=CIRCLE('',#16529,47.175) ;
#3960=CIRCLE('',#16530,47.175) ;
#3961=CIRCLE('',#16532,49.2411809548975) ;
#3962=CIRCLE('',#16533,49.2411809548975) ;
#3963=CIRCLE('',#16535,47.0433475024126) ;
#3964=CIRCLE('',#16537,40.) ;
#3965=CIRCLE('',#16539,40.) ;
#3966=CIRCLE('',#16541,37.5) ;
#3967=CIRCLE('',#16543,37.5) ;
#3968=CIRCLE('',#16545,20.) ;
#3969=CIRCLE('',#16547,0.539999999999986) ;
#3970=CIRCLE('',#16548,0.539999999999996) ;
#3971=CIRCLE('',#16549,1.4) ;
#3972=CIRCLE('',#16551,0.539999999999986) ;
#3973=CIRCLE('',#16552,1.4) ;
#3974=CIRCLE('',#16553,0.539999999999996) ;
#3975=CIRCLE('',#16558,0.539999999999996) ;
#3976=CIRCLE('',#16559,1.4) ;
#3977=CIRCLE('',#16560,0.539999999999986) ;
#3978=CIRCLE('',#16562,0.539999999999986) ;
#3979=CIRCLE('',#16563,1.4) ;
#3980=CIRCLE('',#16564,0.539999999999996) ;
#3981=CIRCLE('',#16569,0.539999999999996) ;
#3982=CIRCLE('',#16570,1.4) ;
#3983=CIRCLE('',#16571,0.539999999999986) ;
#3984=CIRCLE('',#16573,0.539999999999986) ;
#3985=CIRCLE('',#16574,1.4) ;
#3986=CIRCLE('',#16575,0.539999999999996) ;
#3987=CIRCLE('',#16580,0.539999999999996) ;
#3988=CIRCLE('',#16581,1.4) ;
#3989=CIRCLE('',#16582,0.539999999999986) ;
#3990=CIRCLE('',#16584,0.539999999999986) ;
#3991=CIRCLE('',#16585,1.4) ;
#3992=CIRCLE('',#16586,0.539999999999996) ;
#3993=CIRCLE('',#16591,0.539999999999996) ;
#3994=CIRCLE('',#16592,1.4) ;
#3995=CIRCLE('',#16593,0.539999999999986) ;
#3996=CIRCLE('',#16595,0.539999999999986) ;
#3997=CIRCLE('',#16596,1.4) ;
#3998=CIRCLE('',#16597,0.539999999999996) ;
#3999=CIRCLE('',#16602,0.539999999999996) ;
#4000=CIRCLE('',#16603,1.4) ;
#4001=CIRCLE('',#16604,0.539999999999986) ;
#4002=CIRCLE('',#16606,0.539999999999986) ;
#4003=CIRCLE('',#16607,1.4) ;
#4004=CIRCLE('',#16608,0.539999999999996) ;
#4005=CIRCLE('',#16613,0.539999999999996) ;
#4006=CIRCLE('',#16614,1.4) ;
#4007=CIRCLE('',#16615,0.539999999999986) ;
#4008=CIRCLE('',#16617,0.539999999999986) ;
#4009=CIRCLE('',#16618,1.4) ;
#4010=CIRCLE('',#16619,0.539999999999996) ;
#4011=CIRCLE('',#16624,0.539999999999996) ;
#4012=CIRCLE('',#16625,1.4) ;
#4013=CIRCLE('',#16626,0.539999999999986) ;
#4014=CIRCLE('',#16628,0.539999999999986) ;
#4015=CIRCLE('',#16629,1.4) ;
#4016=CIRCLE('',#16630,0.539999999999996) ;
#4017=CIRCLE('',#16635,0.539999999999996) ;
#4018=CIRCLE('',#16636,1.4) ;
#4019=CIRCLE('',#16637,0.539999999999986) ;
#4020=CIRCLE('',#16639,0.539999999999986) ;
#4021=CIRCLE('',#16640,1.4) ;
#4022=CIRCLE('',#16641,0.539999999999996) ;
#4023=CIRCLE('',#16646,0.539999999999996) ;
#4024=CIRCLE('',#16647,1.4) ;
#4025=CIRCLE('',#16648,0.539999999999986) ;
#4026=CIRCLE('',#16650,0.539999999999986) ;
#4027=CIRCLE('',#16651,1.4) ;
#4028=CIRCLE('',#16652,0.539999999999996) ;
#4029=CIRCLE('',#16657,0.539999999999996) ;
#4030=CIRCLE('',#16658,1.4) ;
#4031=CIRCLE('',#16659,0.539999999999986) ;
#4032=CIRCLE('',#16661,0.539999999999986) ;
#4033=CIRCLE('',#16662,1.4) ;
#4034=CIRCLE('',#16663,0.539999999999996) ;
#4035=CIRCLE('',#16668,0.539999999999996) ;
#4036=CIRCLE('',#16669,1.4) ;
#4037=CIRCLE('',#16670,0.539999999999986) ;
#4038=CIRCLE('',#16672,0.539999999999986) ;
#4039=CIRCLE('',#16673,1.4) ;
#4040=CIRCLE('',#16674,0.539999999999996) ;
#4041=CIRCLE('',#16679,0.539999999999996) ;
#4042=CIRCLE('',#16680,1.4) ;
#4043=CIRCLE('',#16681,0.539999999999986) ;
#4044=CIRCLE('',#16683,0.539999999999986) ;
#4045=CIRCLE('',#16684,1.4) ;
#4046=CIRCLE('',#16685,0.539999999999996) ;
#4047=CIRCLE('',#16690,0.539999999999996) ;
#4048=CIRCLE('',#16691,1.4) ;
#4049=CIRCLE('',#16692,0.539999999999986) ;
#4050=CIRCLE('',#16694,0.539999999999986) ;
#4051=CIRCLE('',#16695,1.4) ;
#4052=CIRCLE('',#16696,0.539999999999996) ;
#4053=CIRCLE('',#16701,0.539999999999996) ;
#4054=CIRCLE('',#16702,1.4) ;
#4055=CIRCLE('',#16703,0.539999999999986) ;
#4056=CIRCLE('',#16705,0.539999999999986) ;
#4057=CIRCLE('',#16706,1.4) ;
#4058=CIRCLE('',#16707,0.539999999999996) ;
#4059=CIRCLE('',#16712,0.539999999999996) ;
#4060=CIRCLE('',#16713,1.4) ;
#4061=CIRCLE('',#16714,0.539999999999986) ;
#4062=CIRCLE('',#16716,0.539999999999986) ;
#4063=CIRCLE('',#16717,1.4) ;
#4064=CIRCLE('',#16718,0.539999999999996) ;
#4065=CIRCLE('',#16723,0.539999999999996) ;
#4066=CIRCLE('',#16724,1.4) ;
#4067=CIRCLE('',#16725,0.539999999999986) ;
#4068=CIRCLE('',#16727,0.539999999999986) ;
#4069=CIRCLE('',#16728,1.4) ;
#4070=CIRCLE('',#16729,0.539999999999996) ;
#4071=CIRCLE('',#16734,0.539999999999996) ;
#4072=CIRCLE('',#16735,1.4) ;
#4073=CIRCLE('',#16736,0.539999999999986) ;
#4074=CIRCLE('',#16738,0.539999999999986) ;
#4075=CIRCLE('',#16739,1.4) ;
#4076=CIRCLE('',#16740,0.539999999999996) ;
#4077=CIRCLE('',#16745,0.539999999999996) ;
#4078=CIRCLE('',#16746,1.4) ;
#4079=CIRCLE('',#16747,0.539999999999986) ;
#4080=CIRCLE('',#16749,0.539999999999986) ;
#4081=CIRCLE('',#16750,1.4) ;
#4082=CIRCLE('',#16751,0.539999999999996) ;
#4083=CIRCLE('',#16756,0.539999999999996) ;
#4084=CIRCLE('',#16757,1.4) ;
#4085=CIRCLE('',#16758,0.539999999999986) ;
#4086=CIRCLE('',#16760,0.539999999999986) ;
#4087=CIRCLE('',#16761,1.4) ;
#4088=CIRCLE('',#16762,0.539999999999996) ;
#4089=CIRCLE('',#16767,0.539999999999996) ;
#4090=CIRCLE('',#16768,1.4) ;
#4091=CIRCLE('',#16769,0.539999999999986) ;
#4092=CIRCLE('',#16771,0.539999999999986) ;
#4093=CIRCLE('',#16772,1.4) ;
#4094=CIRCLE('',#16773,0.539999999999996) ;
#4095=CIRCLE('',#16778,0.539999999999996) ;
#4096=CIRCLE('',#16779,1.4) ;
#4097=CIRCLE('',#16780,0.539999999999986) ;
#4098=CIRCLE('',#16782,0.539999999999986) ;
#4099=CIRCLE('',#16783,1.4) ;
#4100=CIRCLE('',#16784,0.539999999999996) ;
#4101=CIRCLE('',#16789,0.539999999999996) ;
#4102=CIRCLE('',#16790,1.4) ;
#4103=CIRCLE('',#16791,0.539999999999986) ;
#4104=CIRCLE('',#16793,0.539999999999986) ;
#4105=CIRCLE('',#16794,1.4) ;
#4106=CIRCLE('',#16795,0.539999999999996) ;
#4107=CIRCLE('',#16800,0.539999999999996) ;
#4108=CIRCLE('',#16801,1.4) ;
#4109=CIRCLE('',#16802,0.539999999999986) ;
#4110=CIRCLE('',#16804,0.539999999999986) ;
#4111=CIRCLE('',#16805,1.4) ;
#4112=CIRCLE('',#16806,0.539999999999996) ;
#4113=CIRCLE('',#16811,0.539999999999996) ;
#4114=CIRCLE('',#16812,1.4) ;
#4115=CIRCLE('',#16813,0.539999999999986) ;
#4116=CIRCLE('',#16815,0.539999999999986) ;
#4117=CIRCLE('',#16816,1.4) ;
#4118=CIRCLE('',#16817,0.539999999999996) ;
#4119=CIRCLE('',#16822,0.539999999999996) ;
#4120=CIRCLE('',#16823,1.4) ;
#4121=CIRCLE('',#16824,0.539999999999986) ;
#4122=CIRCLE('',#16826,0.539999999999986) ;
#4123=CIRCLE('',#16827,1.4) ;
#4124=CIRCLE('',#16828,0.539999999999996) ;
#4125=CIRCLE('',#16833,0.539999999999996) ;
#4126=CIRCLE('',#16834,1.4) ;
#4127=CIRCLE('',#16835,0.539999999999986) ;
#4128=CIRCLE('',#16837,0.539999999999986) ;
#4129=CIRCLE('',#16838,1.4) ;
#4130=CIRCLE('',#16839,0.539999999999996) ;
#4131=CIRCLE('',#16844,0.539999999999996) ;
#4132=CIRCLE('',#16845,1.4) ;
#4133=CIRCLE('',#16846,0.539999999999986) ;
#4134=CIRCLE('',#16848,0.539999999999986) ;
#4135=CIRCLE('',#16849,1.4) ;
#4136=CIRCLE('',#16850,0.539999999999996) ;
#4137=CIRCLE('',#16855,0.539999999999996) ;
#4138=CIRCLE('',#16856,1.4) ;
#4139=CIRCLE('',#16857,0.539999999999986) ;
#4140=CIRCLE('',#16859,0.539999999999986) ;
#4141=CIRCLE('',#16860,1.4) ;
#4142=CIRCLE('',#16861,0.539999999999996) ;
#4143=CIRCLE('',#16866,0.539999999999996) ;
#4144=CIRCLE('',#16867,1.4) ;
#4145=CIRCLE('',#16868,0.539999999999986) ;
#4146=CIRCLE('',#16870,0.539999999999986) ;
#4147=CIRCLE('',#16871,1.4) ;
#4148=CIRCLE('',#16872,0.539999999999996) ;
#4149=CIRCLE('',#16877,0.539999999999996) ;
#4150=CIRCLE('',#16878,1.4) ;
#4151=CIRCLE('',#16879,0.539999999999986) ;
#4152=CIRCLE('',#16881,0.539999999999986) ;
#4153=CIRCLE('',#16882,1.4) ;
#4154=CIRCLE('',#16883,0.539999999999996) ;
#4155=CIRCLE('',#16888,0.539999999999996) ;
#4156=CIRCLE('',#16889,1.4) ;
#4157=CIRCLE('',#16890,0.539999999999986) ;
#4158=CIRCLE('',#16892,0.539999999999986) ;
#4159=CIRCLE('',#16893,1.4) ;
#4160=CIRCLE('',#16894,0.539999999999996) ;
#4161=CIRCLE('',#16899,0.539999999999996) ;
#4162=CIRCLE('',#16900,1.4) ;
#4163=CIRCLE('',#16901,0.539999999999986) ;
#4164=CIRCLE('',#16903,0.539999999999986) ;
#4165=CIRCLE('',#16904,1.4) ;
#4166=CIRCLE('',#16905,0.539999999999996) ;
#4167=CIRCLE('',#16910,0.539999999999996) ;
#4168=CIRCLE('',#16911,1.4) ;
#4169=CIRCLE('',#16912,0.539999999999986) ;
#4170=CIRCLE('',#16914,0.539999999999986) ;
#4171=CIRCLE('',#16915,1.4) ;
#4172=CIRCLE('',#16916,0.539999999999996) ;
#4173=CIRCLE('',#16921,0.539999999999996) ;
#4174=CIRCLE('',#16922,1.4) ;
#4175=CIRCLE('',#16923,0.539999999999986) ;
#4176=CIRCLE('',#16925,0.539999999999986) ;
#4177=CIRCLE('',#16926,1.4) ;
#4178=CIRCLE('',#16927,0.539999999999996) ;
#4179=CIRCLE('',#16932,0.539999999999996) ;
#4180=CIRCLE('',#16933,1.4) ;
#4181=CIRCLE('',#16934,0.539999999999986) ;
#4182=CIRCLE('',#16936,0.539999999999986) ;
#4183=CIRCLE('',#16937,1.4) ;
#4184=CIRCLE('',#16938,0.539999999999996) ;
#4185=CIRCLE('',#16943,0.539999999999996) ;
#4186=CIRCLE('',#16944,1.4) ;
#4187=CIRCLE('',#16945,0.539999999999986) ;
#4188=CIRCLE('',#16947,0.539999999999986) ;
#4189=CIRCLE('',#16948,1.4) ;
#4190=CIRCLE('',#16949,0.539999999999996) ;
#4191=CIRCLE('',#16954,0.539999999999996) ;
#4192=CIRCLE('',#16955,1.4) ;
#4193=CIRCLE('',#16956,0.539999999999986) ;
#4194=CIRCLE('',#16958,0.539999999999986) ;
#4195=CIRCLE('',#16959,1.4) ;
#4196=CIRCLE('',#16960,0.539999999999996) ;
#4197=CIRCLE('',#16965,0.539999999999996) ;
#4198=CIRCLE('',#16966,1.4) ;
#4199=CIRCLE('',#16967,0.539999999999986) ;
#4200=CIRCLE('',#16969,0.539999999999986) ;
#4201=CIRCLE('',#16970,1.4) ;
#4202=CIRCLE('',#16971,0.539999999999996) ;
#4203=CIRCLE('',#16976,0.539999999999996) ;
#4204=CIRCLE('',#16977,1.4) ;
#4205=CIRCLE('',#16978,0.539999999999986) ;
#4206=CIRCLE('',#16980,0.539999999999986) ;
#4207=CIRCLE('',#16981,1.4) ;
#4208=CIRCLE('',#16982,0.539999999999996) ;
#4209=CIRCLE('',#16987,0.539999999999996) ;
#4210=CIRCLE('',#16988,1.4) ;
#4211=CIRCLE('',#16989,0.539999999999986) ;
#4212=CIRCLE('',#16991,0.539999999999986) ;
#4213=CIRCLE('',#16992,1.4) ;
#4214=CIRCLE('',#16993,0.539999999999996) ;
#4215=CIRCLE('',#16998,0.539999999999996) ;
#4216=CIRCLE('',#16999,1.4) ;
#4217=CIRCLE('',#17000,0.539999999999986) ;
#4218=CIRCLE('',#17002,0.539999999999986) ;
#4219=CIRCLE('',#17003,1.4) ;
#4220=CIRCLE('',#17004,0.539999999999996) ;
#4221=CIRCLE('',#17009,0.539999999999996) ;
#4222=CIRCLE('',#17010,1.4) ;
#4223=CIRCLE('',#17011,0.539999999999986) ;
#4224=CIRCLE('',#17013,0.539999999999986) ;
#4225=CIRCLE('',#17014,1.4) ;
#4226=CIRCLE('',#17015,0.539999999999996) ;
#4227=CIRCLE('',#17020,0.539999999999996) ;
#4228=CIRCLE('',#17021,1.4) ;
#4229=CIRCLE('',#17022,0.539999999999986) ;
#4230=CIRCLE('',#17024,0.539999999999986) ;
#4231=CIRCLE('',#17025,1.4) ;
#4232=CIRCLE('',#17026,0.539999999999996) ;
#4233=CIRCLE('',#17031,0.539999999999996) ;
#4234=CIRCLE('',#17032,1.4) ;
#4235=CIRCLE('',#17033,0.539999999999986) ;
#4236=CIRCLE('',#17035,0.539999999999986) ;
#4237=CIRCLE('',#17036,1.4) ;
#4238=CIRCLE('',#17037,0.539999999999996) ;
#4239=CIRCLE('',#17042,0.539999999999996) ;
#4240=CIRCLE('',#17043,1.4) ;
#4241=CIRCLE('',#17044,0.539999999999986) ;
#4242=CIRCLE('',#17046,0.539999999999986) ;
#4243=CIRCLE('',#17047,1.4) ;
#4244=CIRCLE('',#17048,0.539999999999996) ;
#4245=CIRCLE('',#17053,0.539999999999996) ;
#4246=CIRCLE('',#17054,1.4) ;
#4247=CIRCLE('',#17055,0.539999999999986) ;
#4248=CIRCLE('',#17057,0.539999999999986) ;
#4249=CIRCLE('',#17058,1.4) ;
#4250=CIRCLE('',#17059,0.539999999999996) ;
#4251=CIRCLE('',#17064,0.539999999999996) ;
#4252=CIRCLE('',#17065,1.4) ;
#4253=CIRCLE('',#17066,0.539999999999986) ;
#4254=CIRCLE('',#17068,0.539999999999986) ;
#4255=CIRCLE('',#17069,1.4) ;
#4256=CIRCLE('',#17070,0.539999999999996) ;
#4257=CIRCLE('',#17075,0.539999999999996) ;
#4258=CIRCLE('',#17076,1.4) ;
#4259=CIRCLE('',#17077,0.539999999999986) ;
#4260=CIRCLE('',#17079,0.539999999999986) ;
#4261=CIRCLE('',#17080,1.4) ;
#4262=CIRCLE('',#17081,0.539999999999996) ;
#4263=CIRCLE('',#17086,0.539999999999996) ;
#4264=CIRCLE('',#17087,1.4) ;
#4265=CIRCLE('',#17088,0.539999999999986) ;
#4266=CIRCLE('',#17090,0.539999999999986) ;
#4267=CIRCLE('',#17091,1.4) ;
#4268=CIRCLE('',#17092,0.539999999999996) ;
#4269=CIRCLE('',#17097,0.539999999999996) ;
#4270=CIRCLE('',#17098,1.4) ;
#4271=CIRCLE('',#17099,0.539999999999986) ;
#4272=CIRCLE('',#17101,0.539999999999986) ;
#4273=CIRCLE('',#17102,1.4) ;
#4274=CIRCLE('',#17103,0.539999999999996) ;
#4275=CIRCLE('',#17108,0.539999999999996) ;
#4276=CIRCLE('',#17109,1.4) ;
#4277=CIRCLE('',#17110,0.539999999999986) ;
#4278=CIRCLE('',#17112,0.539999999999986) ;
#4279=CIRCLE('',#17113,1.4) ;
#4280=CIRCLE('',#17114,0.539999999999996) ;
#4281=CIRCLE('',#17119,0.539999999999996) ;
#4282=CIRCLE('',#17120,1.4) ;
#4283=CIRCLE('',#17121,0.539999999999986) ;
#4284=CIRCLE('',#17123,0.539999999999986) ;
#4285=CIRCLE('',#17124,1.4) ;
#4286=CIRCLE('',#17125,0.539999999999996) ;
#4287=CIRCLE('',#17130,0.539999999999996) ;
#4288=CIRCLE('',#17131,1.4) ;
#4289=CIRCLE('',#17132,0.539999999999986) ;
#4290=CIRCLE('',#17134,0.539999999999986) ;
#4291=CIRCLE('',#17135,1.4) ;
#4292=CIRCLE('',#17136,0.539999999999996) ;
#4293=CIRCLE('',#17141,0.539999999999996) ;
#4294=CIRCLE('',#17142,1.4) ;
#4295=CIRCLE('',#17143,0.539999999999986) ;
#4296=CIRCLE('',#17145,0.539999999999986) ;
#4297=CIRCLE('',#17146,1.4) ;
#4298=CIRCLE('',#17147,0.539999999999996) ;
#4299=CIRCLE('',#17152,0.539999999999996) ;
#4300=CIRCLE('',#17153,1.4) ;
#4301=CIRCLE('',#17154,0.539999999999986) ;
#4302=CIRCLE('',#17156,0.539999999999986) ;
#4303=CIRCLE('',#17157,1.4) ;
#4304=CIRCLE('',#17158,0.539999999999996) ;
#4305=CIRCLE('',#17163,0.539999999999996) ;
#4306=CIRCLE('',#17164,1.4) ;
#4307=CIRCLE('',#17165,0.539999999999986) ;
#4308=CIRCLE('',#17167,0.539999999999986) ;
#4309=CIRCLE('',#17168,1.4) ;
#4310=CIRCLE('',#17169,0.539999999999996) ;
#4311=CIRCLE('',#17174,0.539999999999996) ;
#4312=CIRCLE('',#17175,1.4) ;
#4313=CIRCLE('',#17176,0.539999999999986) ;
#4314=CIRCLE('',#17178,0.539999999999986) ;
#4315=CIRCLE('',#17179,1.4) ;
#4316=CIRCLE('',#17180,0.539999999999996) ;
#4317=CIRCLE('',#17185,0.539999999999996) ;
#4318=CIRCLE('',#17186,1.4) ;
#4319=CIRCLE('',#17187,0.539999999999986) ;
#4320=CIRCLE('',#17189,0.539999999999986) ;
#4321=CIRCLE('',#17190,1.4) ;
#4322=CIRCLE('',#17191,0.539999999999996) ;
#4323=CIRCLE('',#17196,0.539999999999996) ;
#4324=CIRCLE('',#17197,1.4) ;
#4325=CIRCLE('',#17198,0.539999999999986) ;
#4326=CIRCLE('',#17200,0.539999999999986) ;
#4327=CIRCLE('',#17201,1.4) ;
#4328=CIRCLE('',#17202,0.539999999999996) ;
#4964=LINE('',#51953,#5620) ;
#4965=LINE('',#51955,#5621) ;
#4966=LINE('',#51957,#5622) ;
#4967=LINE('',#51958,#5623) ;
#4968=LINE('',#51961,#5624) ;
#4969=LINE('',#51963,#5625) ;
#4970=LINE('',#51964,#5626) ;
#4971=LINE('',#51968,#5627) ;
#4972=LINE('',#51969,#5628) ;
#4973=LINE('',#51970,#5629) ;
#4974=LINE('',#51978,#5630) ;
#4975=LINE('',#51982,#5631) ;
#4976=LINE('',#51989,#5632) ;
#4977=LINE('',#51992,#5633) ;
#4978=LINE('',#51998,#5634) ;
#4979=LINE('',#52001,#5635) ;
#4980=LINE('',#52007,#5636) ;
#4981=LINE('',#52010,#5637) ;
#4982=LINE('',#52014,#5638) ;
#4983=LINE('',#52018,#5639) ;
#4984=LINE('',#52023,#5640) ;
#4985=LINE('',#52027,#5641) ;
#4986=LINE('',#52032,#5642) ;
#4987=LINE('',#52036,#5643) ;
#4988=LINE('',#52043,#5644) ;
#4989=LINE('',#52046,#5645) ;
#4990=LINE('',#52052,#5646) ;
#4991=LINE('',#52055,#5647) ;
#4992=LINE('',#52061,#5648) ;
#4993=LINE('',#52064,#5649) ;
#4994=LINE('',#52070,#5650) ;
#4995=LINE('',#52073,#5651) ;
#4996=LINE('',#52079,#5652) ;
#4997=LINE('',#52082,#5653) ;
#4998=LINE('',#52088,#5654) ;
#4999=LINE('',#52091,#5655) ;
#5000=LINE('',#52097,#5656) ;
#5001=LINE('',#52100,#5657) ;
#5002=LINE('',#52106,#5658) ;
#5003=LINE('',#52109,#5659) ;
#5004=LINE('',#52115,#5660) ;
#5005=LINE('',#52118,#5661) ;
#5006=LINE('',#52124,#5662) ;
#5007=LINE('',#52127,#5663) ;
#5008=LINE('',#52133,#5664) ;
#5009=LINE('',#52136,#5665) ;
#5010=LINE('',#52142,#5666) ;
#5011=LINE('',#52145,#5667) ;
#5012=LINE('',#52151,#5668) ;
#5013=LINE('',#52154,#5669) ;
#5014=LINE('',#52158,#5670) ;
#5015=LINE('',#52162,#5671) ;
#5016=LINE('',#52169,#5672) ;
#5017=LINE('',#52172,#5673) ;
#5018=LINE('',#52178,#5674) ;
#5019=LINE('',#52181,#5675) ;
#5020=LINE('',#52187,#5676) ;
#5021=LINE('',#52190,#5677) ;
#5022=LINE('',#52196,#5678) ;
#5023=LINE('',#52199,#5679) ;
#5024=LINE('',#52205,#5680) ;
#5025=LINE('',#52208,#5681) ;
#5026=LINE('',#52214,#5682) ;
#5027=LINE('',#52217,#5683) ;
#5028=LINE('',#52223,#5684) ;
#5029=LINE('',#52226,#5685) ;
#5030=LINE('',#52232,#5686) ;
#5031=LINE('',#52235,#5687) ;
#5032=LINE('',#52241,#5688) ;
#5033=LINE('',#52244,#5689) ;
#5034=LINE('',#52250,#5690) ;
#5035=LINE('',#52253,#5691) ;
#5036=LINE('',#52259,#5692) ;
#5037=LINE('',#52262,#5693) ;
#5038=LINE('',#52266,#5694) ;
#5039=LINE('',#52270,#5695) ;
#5040=LINE('',#52275,#5696) ;
#5041=LINE('',#52279,#5697) ;
#5042=LINE('',#52284,#5698) ;
#5043=LINE('',#52288,#5699) ;
#5044=LINE('',#52293,#5700) ;
#5045=LINE('',#52297,#5701) ;
#5046=LINE('',#52302,#5702) ;
#5047=LINE('',#52306,#5703) ;
#5048=LINE('',#52311,#5704) ;
#5049=LINE('',#52315,#5705) ;
#5050=LINE('',#52320,#5706) ;
#5051=LINE('',#52324,#5707) ;
#5052=LINE('',#52331,#5708) ;
#5053=LINE('',#52334,#5709) ;
#5054=LINE('',#52340,#5710) ;
#5055=LINE('',#52343,#5711) ;
#5056=LINE('',#52349,#5712) ;
#5057=LINE('',#52352,#5713) ;
#5058=LINE('',#52358,#5714) ;
#5059=LINE('',#52361,#5715) ;
#5060=LINE('',#52367,#5716) ;
#5061=LINE('',#52370,#5717) ;
#5062=LINE('',#52376,#5718) ;
#5063=LINE('',#52379,#5719) ;
#5064=LINE('',#52385,#5720) ;
#5065=LINE('',#52388,#5721) ;
#5066=LINE('',#52394,#5722) ;
#5067=LINE('',#52397,#5723) ;
#5068=LINE('',#52403,#5724) ;
#5069=LINE('',#52406,#5725) ;
#5070=LINE('',#52412,#5726) ;
#5071=LINE('',#52415,#5727) ;
#5072=LINE('',#52421,#5728) ;
#5073=LINE('',#52424,#5729) ;
#5074=LINE('',#52428,#5730) ;
#5075=LINE('',#52432,#5731) ;
#5076=LINE('',#52439,#5732) ;
#5077=LINE('',#52442,#5733) ;
#5078=LINE('',#52448,#5734) ;
#5079=LINE('',#52451,#5735) ;
#5080=LINE('',#52457,#5736) ;
#5081=LINE('',#52460,#5737) ;
#5082=LINE('',#52466,#5738) ;
#5083=LINE('',#52469,#5739) ;
#5084=LINE('',#52475,#5740) ;
#5085=LINE('',#52478,#5741) ;
#5086=LINE('',#52484,#5742) ;
#5087=LINE('',#52487,#5743) ;
#5088=LINE('',#52493,#5744) ;
#5089=LINE('',#52496,#5745) ;
#5090=LINE('',#52500,#5746) ;
#5091=LINE('',#52504,#5747) ;
#5092=LINE('',#52511,#5748) ;
#5093=LINE('',#52514,#5749) ;
#5094=LINE('',#52518,#5750) ;
#5095=LINE('',#52524,#5751) ;
#5096=LINE('',#52533,#5752) ;
#5097=LINE('',#52536,#5753) ;
#5098=LINE('',#52604,#5754) ;
#5099=LINE('',#52668,#5755) ;
#5100=LINE('',#52675,#5756) ;
#5101=LINE('',#52682,#5757) ;
#5102=LINE('',#52689,#5758) ;
#5103=LINE('',#52705,#5759) ;
#5104=LINE('',#52707,#5760) ;
#5105=LINE('',#52722,#5761) ;
#5106=LINE('',#52724,#5762) ;
#5107=LINE('',#52739,#5763) ;
#5108=LINE('',#52741,#5764) ;
#5109=LINE('',#52756,#5765) ;
#5110=LINE('',#52758,#5766) ;
#5111=LINE('',#52773,#5767) ;
#5112=LINE('',#52775,#5768) ;
#5113=LINE('',#52790,#5769) ;
#5114=LINE('',#52792,#5770) ;
#5115=LINE('',#52807,#5771) ;
#5116=LINE('',#52809,#5772) ;
#5117=LINE('',#52824,#5773) ;
#5118=LINE('',#52826,#5774) ;
#5119=LINE('',#52841,#5775) ;
#5120=LINE('',#52843,#5776) ;
#5121=LINE('',#52858,#5777) ;
#5122=LINE('',#52860,#5778) ;
#5123=LINE('',#52875,#5779) ;
#5124=LINE('',#52877,#5780) ;
#5125=LINE('',#52892,#5781) ;
#5126=LINE('',#52894,#5782) ;
#5127=LINE('',#52909,#5783) ;
#5128=LINE('',#52911,#5784) ;
#5129=LINE('',#52926,#5785) ;
#5130=LINE('',#52928,#5786) ;
#5131=LINE('',#52943,#5787) ;
#5132=LINE('',#52945,#5788) ;
#5133=LINE('',#52960,#5789) ;
#5134=LINE('',#52962,#5790) ;
#5135=LINE('',#52977,#5791) ;
#5136=LINE('',#52979,#5792) ;
#5137=LINE('',#52994,#5793) ;
#5138=LINE('',#52996,#5794) ;
#5139=LINE('',#53011,#5795) ;
#5140=LINE('',#53013,#5796) ;
#5141=LINE('',#53028,#5797) ;
#5142=LINE('',#53030,#5798) ;
#5143=LINE('',#53045,#5799) ;
#5144=LINE('',#53047,#5800) ;
#5145=LINE('',#53062,#5801) ;
#5146=LINE('',#53064,#5802) ;
#5147=LINE('',#53079,#5803) ;
#5148=LINE('',#53081,#5804) ;
#5149=LINE('',#53096,#5805) ;
#5150=LINE('',#53098,#5806) ;
#5151=LINE('',#53113,#5807) ;
#5152=LINE('',#53115,#5808) ;
#5153=LINE('',#53130,#5809) ;
#5154=LINE('',#53132,#5810) ;
#5155=LINE('',#53147,#5811) ;
#5156=LINE('',#53149,#5812) ;
#5157=LINE('',#53164,#5813) ;
#5158=LINE('',#53166,#5814) ;
#5159=LINE('',#53181,#5815) ;
#5160=LINE('',#53183,#5816) ;
#5161=LINE('',#53198,#5817) ;
#5162=LINE('',#53200,#5818) ;
#5163=LINE('',#53215,#5819) ;
#5164=LINE('',#53217,#5820) ;
#5165=LINE('',#53232,#5821) ;
#5166=LINE('',#53234,#5822) ;
#5167=LINE('',#53249,#5823) ;
#5168=LINE('',#53251,#5824) ;
#5169=LINE('',#53266,#5825) ;
#5170=LINE('',#53268,#5826) ;
#5171=LINE('',#53283,#5827) ;
#5172=LINE('',#53285,#5828) ;
#5173=LINE('',#53300,#5829) ;
#5174=LINE('',#53302,#5830) ;
#5175=LINE('',#53317,#5831) ;
#5176=LINE('',#53319,#5832) ;
#5177=LINE('',#53334,#5833) ;
#5178=LINE('',#53336,#5834) ;
#5179=LINE('',#53351,#5835) ;
#5180=LINE('',#53353,#5836) ;
#5181=LINE('',#53368,#5837) ;
#5182=LINE('',#53370,#5838) ;
#5183=LINE('',#53385,#5839) ;
#5184=LINE('',#53387,#5840) ;
#5185=LINE('',#53402,#5841) ;
#5186=LINE('',#53404,#5842) ;
#5187=LINE('',#53419,#5843) ;
#5188=LINE('',#53421,#5844) ;
#5189=LINE('',#53436,#5845) ;
#5190=LINE('',#53438,#5846) ;
#5191=LINE('',#53453,#5847) ;
#5192=LINE('',#53455,#5848) ;
#5193=LINE('',#53470,#5849) ;
#5194=LINE('',#53472,#5850) ;
#5195=LINE('',#53487,#5851) ;
#5196=LINE('',#53489,#5852) ;
#5197=LINE('',#53504,#5853) ;
#5198=LINE('',#53506,#5854) ;
#5199=LINE('',#53521,#5855) ;
#5200=LINE('',#53523,#5856) ;
#5201=LINE('',#53538,#5857) ;
#5202=LINE('',#53540,#5858) ;
#5203=LINE('',#53555,#5859) ;
#5204=LINE('',#53557,#5860) ;
#5205=LINE('',#53572,#5861) ;
#5206=LINE('',#53574,#5862) ;
#5207=LINE('',#53589,#5863) ;
#5208=LINE('',#53591,#5864) ;
#5209=LINE('',#53606,#5865) ;
#5210=LINE('',#53608,#5866) ;
#5211=LINE('',#53623,#5867) ;
#5212=LINE('',#53625,#5868) ;
#5213=LINE('',#53640,#5869) ;
#5214=LINE('',#53642,#5870) ;
#5215=LINE('',#53657,#5871) ;
#5216=LINE('',#53659,#5872) ;
#5217=LINE('',#53674,#5873) ;
#5218=LINE('',#53676,#5874) ;
#5219=LINE('',#53691,#5875) ;
#5220=LINE('',#53693,#5876) ;
#5221=LINE('',#53708,#5877) ;
#5222=LINE('',#53710,#5878) ;
#5620=VECTOR('',#19246,10.) ;
#5621=VECTOR('',#19247,10.) ;
#5622=VECTOR('',#19248,10.) ;
#5623=VECTOR('',#19249,10.) ;
#5624=VECTOR('',#19252,10.) ;
#5625=VECTOR('',#19253,10.) ;
#5626=VECTOR('',#19254,10.) ;
#5627=VECTOR('',#19257,10.) ;
#5628=VECTOR('',#19258,10.) ;
#5629=VECTOR('',#19259,10.) ;
#5630=VECTOR('',#19268,1000.) ;
#5631=VECTOR('',#19271,1000.) ;
#5632=VECTOR('',#19278,1000.) ;
#5633=VECTOR('',#19281,1000.) ;
#5634=VECTOR('',#19286,1000.) ;
#5635=VECTOR('',#19289,1000.) ;
#5636=VECTOR('',#19294,1000.) ;
#5637=VECTOR('',#19297,1000.) ;
#5638=VECTOR('',#19300,1000.) ;
#5639=VECTOR('',#19303,1000.) ;
#5640=VECTOR('',#19308,1000.) ;
#5641=VECTOR('',#19311,1000.) ;
#5642=VECTOR('',#19316,1000.) ;
#5643=VECTOR('',#19319,1000.) ;
#5644=VECTOR('',#19326,1000.) ;
#5645=VECTOR('',#19329,1000.) ;
#5646=VECTOR('',#19334,1000.) ;
#5647=VECTOR('',#19337,1000.) ;
#5648=VECTOR('',#19342,1000.) ;
#5649=VECTOR('',#19345,1000.) ;
#5650=VECTOR('',#19350,1000.) ;
#5651=VECTOR('',#19353,1000.) ;
#5652=VECTOR('',#19358,1000.) ;
#5653=VECTOR('',#19361,1000.) ;
#5654=VECTOR('',#19366,1000.) ;
#5655=VECTOR('',#19369,1000.) ;
#5656=VECTOR('',#19374,1000.) ;
#5657=VECTOR('',#19377,1000.) ;
#5658=VECTOR('',#19382,1000.) ;
#5659=VECTOR('',#19385,1000.) ;
#5660=VECTOR('',#19390,1000.) ;
#5661=VECTOR('',#19393,1000.) ;
#5662=VECTOR('',#19398,1000.) ;
#5663=VECTOR('',#19401,1000.) ;
#5664=VECTOR('',#19406,1000.) ;
#5665=VECTOR('',#19409,1000.) ;
#5666=VECTOR('',#19414,1000.) ;
#5667=VECTOR('',#19417,1000.) ;
#5668=VECTOR('',#19422,1000.) ;
#5669=VECTOR('',#19425,1000.) ;
#5670=VECTOR('',#19428,1000.) ;
#5671=VECTOR('',#19431,1000.) ;
#5672=VECTOR('',#19438,1000.) ;
#5673=VECTOR('',#19441,1000.) ;
#5674=VECTOR('',#19446,1000.) ;
#5675=VECTOR('',#19449,1000.) ;
#5676=VECTOR('',#19454,1000.) ;
#5677=VECTOR('',#19457,1000.) ;
#5678=VECTOR('',#19462,1000.) ;
#5679=VECTOR('',#19465,1000.) ;
#5680=VECTOR('',#19470,1000.) ;
#5681=VECTOR('',#19473,1000.) ;
#5682=VECTOR('',#19478,1000.) ;
#5683=VECTOR('',#19481,1000.) ;
#5684=VECTOR('',#19486,1000.) ;
#5685=VECTOR('',#19489,1000.) ;
#5686=VECTOR('',#19494,1000.) ;
#5687=VECTOR('',#19497,1000.) ;
#5688=VECTOR('',#19502,1000.) ;
#5689=VECTOR('',#19505,1000.) ;
#5690=VECTOR('',#19510,1000.) ;
#5691=VECTOR('',#19513,1000.) ;
#5692=VECTOR('',#19518,1000.) ;
#5693=VECTOR('',#19521,1000.) ;
#5694=VECTOR('',#19524,1000.) ;
#5695=VECTOR('',#19527,1000.) ;
#5696=VECTOR('',#19532,1000.) ;
#5697=VECTOR('',#19535,1000.) ;
#5698=VECTOR('',#19540,1000.) ;
#5699=VECTOR('',#19543,1000.) ;
#5700=VECTOR('',#19548,1000.) ;
#5701=VECTOR('',#19551,1000.) ;
#5702=VECTOR('',#19556,1000.) ;
#5703=VECTOR('',#19559,1000.) ;
#5704=VECTOR('',#19564,1000.) ;
#5705=VECTOR('',#19567,1000.) ;
#5706=VECTOR('',#19572,1000.) ;
#5707=VECTOR('',#19575,1000.) ;
#5708=VECTOR('',#19582,1000.) ;
#5709=VECTOR('',#19585,1000.) ;
#5710=VECTOR('',#19590,1000.) ;
#5711=VECTOR('',#19593,1000.) ;
#5712=VECTOR('',#19598,1000.) ;
#5713=VECTOR('',#19601,1000.) ;
#5714=VECTOR('',#19606,1000.) ;
#5715=VECTOR('',#19609,1000.) ;
#5716=VECTOR('',#19614,1000.) ;
#5717=VECTOR('',#19617,1000.) ;
#5718=VECTOR('',#19622,1000.) ;
#5719=VECTOR('',#19625,1000.) ;
#5720=VECTOR('',#19630,1000.) ;
#5721=VECTOR('',#19633,1000.) ;
#5722=VECTOR('',#19638,1000.) ;
#5723=VECTOR('',#19641,1000.) ;
#5724=VECTOR('',#19646,1000.) ;
#5725=VECTOR('',#19649,1000.) ;
#5726=VECTOR('',#19654,1000.) ;
#5727=VECTOR('',#19657,1000.) ;
#5728=VECTOR('',#19662,1000.) ;
#5729=VECTOR('',#19665,1000.) ;
#5730=VECTOR('',#19668,1000.) ;
#5731=VECTOR('',#19671,1000.) ;
#5732=VECTOR('',#19678,1000.) ;
#5733=VECTOR('',#19681,1000.) ;
#5734=VECTOR('',#19686,1000.) ;
#5735=VECTOR('',#19689,1000.) ;
#5736=VECTOR('',#19694,1000.) ;
#5737=VECTOR('',#19697,1000.) ;
#5738=VECTOR('',#19702,1000.) ;
#5739=VECTOR('',#19705,1000.) ;
#5740=VECTOR('',#19710,1000.) ;
#5741=VECTOR('',#19713,1000.) ;
#5742=VECTOR('',#19718,1000.) ;
#5743=VECTOR('',#19721,1000.) ;
#5744=VECTOR('',#19726,1000.) ;
#5745=VECTOR('',#19729,1000.) ;
#5746=VECTOR('',#19732,1000.) ;
#5747=VECTOR('',#19735,1000.) ;
#5748=VECTOR('',#19742,1000.) ;
#5749=VECTOR('',#19745,1000.) ;
#5750=VECTOR('',#19750,40.) ;
#5751=VECTOR('',#19757,47.0433475024125) ;
#5752=VECTOR('',#19768,49.2411809548974) ;
#5753=VECTOR('',#19771,49.5) ;
#5754=VECTOR('',#19900,47.175) ;
#5755=VECTOR('',#20025,49.5) ;
#5756=VECTOR('',#20034,49.2411809548975) ;
#5757=VECTOR('',#20043,40.) ;
#5758=VECTOR('',#20052,37.5) ;
#5759=VECTOR('',#20075,1000.) ;
#5760=VECTOR('',#20078,1000.) ;
#5761=VECTOR('',#20099,1000.) ;
#5762=VECTOR('',#20102,1000.) ;
#5763=VECTOR('',#20123,1000.) ;
#5764=VECTOR('',#20126,1000.) ;
#5765=VECTOR('',#20147,1000.) ;
#5766=VECTOR('',#20150,1000.) ;
#5767=VECTOR('',#20171,1000.) ;
#5768=VECTOR('',#20174,1000.) ;
#5769=VECTOR('',#20195,1000.) ;
#5770=VECTOR('',#20198,1000.) ;
#5771=VECTOR('',#20219,1000.) ;
#5772=VECTOR('',#20222,1000.) ;
#5773=VECTOR('',#20243,1000.) ;
#5774=VECTOR('',#20246,1000.) ;
#5775=VECTOR('',#20267,1000.) ;
#5776=VECTOR('',#20270,1000.) ;
#5777=VECTOR('',#20291,1000.) ;
#5778=VECTOR('',#20294,1000.) ;
#5779=VECTOR('',#20315,1000.) ;
#5780=VECTOR('',#20318,1000.) ;
#5781=VECTOR('',#20339,1000.) ;
#5782=VECTOR('',#20342,1000.) ;
#5783=VECTOR('',#20363,1000.) ;
#5784=VECTOR('',#20366,1000.) ;
#5785=VECTOR('',#20387,1000.) ;
#5786=VECTOR('',#20390,1000.) ;
#5787=VECTOR('',#20411,1000.) ;
#5788=VECTOR('',#20414,1000.) ;
#5789=VECTOR('',#20435,1000.) ;
#5790=VECTOR('',#20438,1000.) ;
#5791=VECTOR('',#20459,1000.) ;
#5792=VECTOR('',#20462,1000.) ;
#5793=VECTOR('',#20483,1000.) ;
#5794=VECTOR('',#20486,1000.) ;
#5795=VECTOR('',#20507,1000.) ;
#5796=VECTOR('',#20510,1000.) ;
#5797=VECTOR('',#20531,1000.) ;
#5798=VECTOR('',#20534,1000.) ;
#5799=VECTOR('',#20555,1000.) ;
#5800=VECTOR('',#20558,1000.) ;
#5801=VECTOR('',#20579,1000.) ;
#5802=VECTOR('',#20582,1000.) ;
#5803=VECTOR('',#20603,1000.) ;
#5804=VECTOR('',#20606,1000.) ;
#5805=VECTOR('',#20627,1000.) ;
#5806=VECTOR('',#20630,1000.) ;
#5807=VECTOR('',#20651,1000.) ;
#5808=VECTOR('',#20654,1000.) ;
#5809=VECTOR('',#20675,1000.) ;
#5810=VECTOR('',#20678,1000.) ;
#5811=VECTOR('',#20699,1000.) ;
#5812=VECTOR('',#20702,1000.) ;
#5813=VECTOR('',#20723,1000.) ;
#5814=VECTOR('',#20726,1000.) ;
#5815=VECTOR('',#20747,1000.) ;
#5816=VECTOR('',#20750,1000.) ;
#5817=VECTOR('',#20771,1000.) ;
#5818=VECTOR('',#20774,1000.) ;
#5819=VECTOR('',#20795,1000.) ;
#5820=VECTOR('',#20798,1000.) ;
#5821=VECTOR('',#20819,1000.) ;
#5822=VECTOR('',#20822,1000.) ;
#5823=VECTOR('',#20843,1000.) ;
#5824=VECTOR('',#20846,1000.) ;
#5825=VECTOR('',#20867,1000.) ;
#5826=VECTOR('',#20870,1000.) ;
#5827=VECTOR('',#20891,1000.) ;
#5828=VECTOR('',#20894,1000.) ;
#5829=VECTOR('',#20915,1000.) ;
#5830=VECTOR('',#20918,1000.) ;
#5831=VECTOR('',#20939,1000.) ;
#5832=VECTOR('',#20942,1000.) ;
#5833=VECTOR('',#20963,1000.) ;
#5834=VECTOR('',#20966,1000.) ;
#5835=VECTOR('',#20987,1000.) ;
#5836=VECTOR('',#20990,1000.) ;
#5837=VECTOR('',#21011,1000.) ;
#5838=VECTOR('',#21014,1000.) ;
#5839=VECTOR('',#21035,1000.) ;
#5840=VECTOR('',#21038,1000.) ;
#5841=VECTOR('',#21059,1000.) ;
#5842=VECTOR('',#21062,1000.) ;
#5843=VECTOR('',#21083,1000.) ;
#5844=VECTOR('',#21086,1000.) ;
#5845=VECTOR('',#21107,1000.) ;
#5846=VECTOR('',#21110,1000.) ;
#5847=VECTOR('',#21131,1000.) ;
#5848=VECTOR('',#21134,1000.) ;
#5849=VECTOR('',#21155,1000.) ;
#5850=VECTOR('',#21158,1000.) ;
#5851=VECTOR('',#21179,1000.) ;
#5852=VECTOR('',#21182,1000.) ;
#5853=VECTOR('',#21203,1000.) ;
#5854=VECTOR('',#21206,1000.) ;
#5855=VECTOR('',#21227,1000.) ;
#5856=VECTOR('',#21230,1000.) ;
#5857=VECTOR('',#21251,1000.) ;
#5858=VECTOR('',#21254,1000.) ;
#5859=VECTOR('',#21275,1000.) ;
#5860=VECTOR('',#21278,1000.) ;
#5861=VECTOR('',#21299,1000.) ;
#5862=VECTOR('',#21302,1000.) ;
#5863=VECTOR('',#21323,1000.) ;
#5864=VECTOR('',#21326,1000.) ;
#5865=VECTOR('',#21347,1000.) ;
#5866=VECTOR('',#21350,1000.) ;
#5867=VECTOR('',#21371,1000.) ;
#5868=VECTOR('',#21374,1000.) ;
#5869=VECTOR('',#21395,1000.) ;
#5870=VECTOR('',#21398,1000.) ;
#5871=VECTOR('',#21419,1000.) ;
#5872=VECTOR('',#21422,1000.) ;
#5873=VECTOR('',#21443,1000.) ;
#5874=VECTOR('',#21446,1000.) ;
#5875=VECTOR('',#21467,1000.) ;
#5876=VECTOR('',#21470,1000.) ;
#5877=VECTOR('',#21491,1000.) ;
#5878=VECTOR('',#21494,1000.) ;
#6435=VERTEX_POINT('',#51951) ;
#6436=VERTEX_POINT('',#51952) ;
#6437=VERTEX_POINT('',#51954) ;
#6438=VERTEX_POINT('',#51956) ;
#6439=VERTEX_POINT('',#51960) ;
#6440=VERTEX_POINT('',#51962) ;
#6441=VERTEX_POINT('',#51966) ;
#6442=VERTEX_POINT('',#51967) ;
#6443=VERTEX_POINT('',#51972) ;
#6444=VERTEX_POINT('',#51976) ;
#6445=VERTEX_POINT('',#51977) ;
#6446=VERTEX_POINT('',#51979) ;
#6447=VERTEX_POINT('',#51981) ;
#6448=VERTEX_POINT('',#51985) ;
#6449=VERTEX_POINT('',#51986) ;
#6450=VERTEX_POINT('',#51988) ;
#6451=VERTEX_POINT('',#51990) ;
#6452=VERTEX_POINT('',#51994) ;
#6453=VERTEX_POINT('',#51995) ;
#6454=VERTEX_POINT('',#51997) ;
#6455=VERTEX_POINT('',#51999) ;
#6456=VERTEX_POINT('',#52003) ;
#6457=VERTEX_POINT('',#52004) ;
#6458=VERTEX_POINT('',#52006) ;
#6459=VERTEX_POINT('',#52008) ;
#6460=VERTEX_POINT('',#52012) ;
#6461=VERTEX_POINT('',#52013) ;
#6462=VERTEX_POINT('',#52015) ;
#6463=VERTEX_POINT('',#52017) ;
#6464=VERTEX_POINT('',#52021) ;
#6465=VERTEX_POINT('',#52022) ;
#6466=VERTEX_POINT('',#52024) ;
#6467=VERTEX_POINT('',#52026) ;
#6468=VERTEX_POINT('',#52030) ;
#6469=VERTEX_POINT('',#52031) ;
#6470=VERTEX_POINT('',#52033) ;
#6471=VERTEX_POINT('',#52035) ;
#6472=VERTEX_POINT('',#52039) ;
#6473=VERTEX_POINT('',#52040) ;
#6474=VERTEX_POINT('',#52042) ;
#6475=VERTEX_POINT('',#52044) ;
#6476=VERTEX_POINT('',#52048) ;
#6477=VERTEX_POINT('',#52049) ;
#6478=VERTEX_POINT('',#52051) ;
#6479=VERTEX_POINT('',#52053) ;
#6480=VERTEX_POINT('',#52057) ;
#6481=VERTEX_POINT('',#52058) ;
#6482=VERTEX_POINT('',#52060) ;
#6483=VERTEX_POINT('',#52062) ;
#6484=VERTEX_POINT('',#52066) ;
#6485=VERTEX_POINT('',#52067) ;
#6486=VERTEX_POINT('',#52069) ;
#6487=VERTEX_POINT('',#52071) ;
#6488=VERTEX_POINT('',#52075) ;
#6489=VERTEX_POINT('',#52076) ;
#6490=VERTEX_POINT('',#52078) ;
#6491=VERTEX_POINT('',#52080) ;
#6492=VERTEX_POINT('',#52084) ;
#6493=VERTEX_POINT('',#52085) ;
#6494=VERTEX_POINT('',#52087) ;
#6495=VERTEX_POINT('',#52089) ;
#6496=VERTEX_POINT('',#52093) ;
#6497=VERTEX_POINT('',#52094) ;
#6498=VERTEX_POINT('',#52096) ;
#6499=VERTEX_POINT('',#52098) ;
#6500=VERTEX_POINT('',#52102) ;
#6501=VERTEX_POINT('',#52103) ;
#6502=VERTEX_POINT('',#52105) ;
#6503=VERTEX_POINT('',#52107) ;
#6504=VERTEX_POINT('',#52111) ;
#6505=VERTEX_POINT('',#52112) ;
#6506=VERTEX_POINT('',#52114) ;
#6507=VERTEX_POINT('',#52116) ;
#6508=VERTEX_POINT('',#52120) ;
#6509=VERTEX_POINT('',#52121) ;
#6510=VERTEX_POINT('',#52123) ;
#6511=VERTEX_POINT('',#52125) ;
#6512=VERTEX_POINT('',#52129) ;
#6513=VERTEX_POINT('',#52130) ;
#6514=VERTEX_POINT('',#52132) ;
#6515=VERTEX_POINT('',#52134) ;
#6516=VERTEX_POINT('',#52138) ;
#6517=VERTEX_POINT('',#52139) ;
#6518=VERTEX_POINT('',#52141) ;
#6519=VERTEX_POINT('',#52143) ;
#6520=VERTEX_POINT('',#52147) ;
#6521=VERTEX_POINT('',#52148) ;
#6522=VERTEX_POINT('',#52150) ;
#6523=VERTEX_POINT('',#52152) ;
#6524=VERTEX_POINT('',#52156) ;
#6525=VERTEX_POINT('',#52157) ;
#6526=VERTEX_POINT('',#52159) ;
#6527=VERTEX_POINT('',#52161) ;
#6528=VERTEX_POINT('',#52165) ;
#6529=VERTEX_POINT('',#52166) ;
#6530=VERTEX_POINT('',#52168) ;
#6531=VERTEX_POINT('',#52170) ;
#6532=VERTEX_POINT('',#52174) ;
#6533=VERTEX_POINT('',#52175) ;
#6534=VERTEX_POINT('',#52177) ;
#6535=VERTEX_POINT('',#52179) ;
#6536=VERTEX_POINT('',#52183) ;
#6537=VERTEX_POINT('',#52184) ;
#6538=VERTEX_POINT('',#52186) ;
#6539=VERTEX_POINT('',#52188) ;
#6540=VERTEX_POINT('',#52192) ;
#6541=VERTEX_POINT('',#52193) ;
#6542=VERTEX_POINT('',#52195) ;
#6543=VERTEX_POINT('',#52197) ;
#6544=VERTEX_POINT('',#52201) ;
#6545=VERTEX_POINT('',#52202) ;
#6546=VERTEX_POINT('',#52204) ;
#6547=VERTEX_POINT('',#52206) ;
#6548=VERTEX_POINT('',#52210) ;
#6549=VERTEX_POINT('',#52211) ;
#6550=VERTEX_POINT('',#52213) ;
#6551=VERTEX_POINT('',#52215) ;
#6552=VERTEX_POINT('',#52219) ;
#6553=VERTEX_POINT('',#52220) ;
#6554=VERTEX_POINT('',#52222) ;
#6555=VERTEX_POINT('',#52224) ;
#6556=VERTEX_POINT('',#52228) ;
#6557=VERTEX_POINT('',#52229) ;
#6558=VERTEX_POINT('',#52231) ;
#6559=VERTEX_POINT('',#52233) ;
#6560=VERTEX_POINT('',#52237) ;
#6561=VERTEX_POINT('',#52238) ;
#6562=VERTEX_POINT('',#52240) ;
#6563=VERTEX_POINT('',#52242) ;
#6564=VERTEX_POINT('',#52246) ;
#6565=VERTEX_POINT('',#52247) ;
#6566=VERTEX_POINT('',#52249) ;
#6567=VERTEX_POINT('',#52251) ;
#6568=VERTEX_POINT('',#52255) ;
#6569=VERTEX_POINT('',#52256) ;
#6570=VERTEX_POINT('',#52258) ;
#6571=VERTEX_POINT('',#52260) ;
#6572=VERTEX_POINT('',#52264) ;
#6573=VERTEX_POINT('',#52265) ;
#6574=VERTEX_POINT('',#52267) ;
#6575=VERTEX_POINT('',#52269) ;
#6576=VERTEX_POINT('',#52273) ;
#6577=VERTEX_POINT('',#52274) ;
#6578=VERTEX_POINT('',#52276) ;
#6579=VERTEX_POINT('',#52278) ;
#6580=VERTEX_POINT('',#52282) ;
#6581=VERTEX_POINT('',#52283) ;
#6582=VERTEX_POINT('',#52285) ;
#6583=VERTEX_POINT('',#52287) ;
#6584=VERTEX_POINT('',#52291) ;
#6585=VERTEX_POINT('',#52292) ;
#6586=VERTEX_POINT('',#52294) ;
#6587=VERTEX_POINT('',#52296) ;
#6588=VERTEX_POINT('',#52300) ;
#6589=VERTEX_POINT('',#52301) ;
#6590=VERTEX_POINT('',#52303) ;
#6591=VERTEX_POINT('',#52305) ;
#6592=VERTEX_POINT('',#52309) ;
#6593=VERTEX_POINT('',#52310) ;
#6594=VERTEX_POINT('',#52312) ;
#6595=VERTEX_POINT('',#52314) ;
#6596=VERTEX_POINT('',#52318) ;
#6597=VERTEX_POINT('',#52319) ;
#6598=VERTEX_POINT('',#52321) ;
#6599=VERTEX_POINT('',#52323) ;
#6600=VERTEX_POINT('',#52327) ;
#6601=VERTEX_POINT('',#52328) ;
#6602=VERTEX_POINT('',#52330) ;
#6603=VERTEX_POINT('',#52332) ;
#6604=VERTEX_POINT('',#52336) ;
#6605=VERTEX_POINT('',#52337) ;
#6606=VERTEX_POINT('',#52339) ;
#6607=VERTEX_POINT('',#52341) ;
#6608=VERTEX_POINT('',#52345) ;
#6609=VERTEX_POINT('',#52346) ;
#6610=VERTEX_POINT('',#52348) ;
#6611=VERTEX_POINT('',#52350) ;
#6612=VERTEX_POINT('',#52354) ;
#6613=VERTEX_POINT('',#52355) ;
#6614=VERTEX_POINT('',#52357) ;
#6615=VERTEX_POINT('',#52359) ;
#6616=VERTEX_POINT('',#52363) ;
#6617=VERTEX_POINT('',#52364) ;
#6618=VERTEX_POINT('',#52366) ;
#6619=VERTEX_POINT('',#52368) ;
#6620=VERTEX_POINT('',#52372) ;
#6621=VERTEX_POINT('',#52373) ;
#6622=VERTEX_POINT('',#52375) ;
#6623=VERTEX_POINT('',#52377) ;
#6624=VERTEX_POINT('',#52381) ;
#6625=VERTEX_POINT('',#52382) ;
#6626=VERTEX_POINT('',#52384) ;
#6627=VERTEX_POINT('',#52386) ;
#6628=VERTEX_POINT('',#52390) ;
#6629=VERTEX_POINT('',#52391) ;
#6630=VERTEX_POINT('',#52393) ;
#6631=VERTEX_POINT('',#52395) ;
#6632=VERTEX_POINT('',#52399) ;
#6633=VERTEX_POINT('',#52400) ;
#6634=VERTEX_POINT('',#52402) ;
#6635=VERTEX_POINT('',#52404) ;
#6636=VERTEX_POINT('',#52408) ;
#6637=VERTEX_POINT('',#52409) ;
#6638=VERTEX_POINT('',#52411) ;
#6639=VERTEX_POINT('',#52413) ;
#6640=VERTEX_POINT('',#52417) ;
#6641=VERTEX_POINT('',#52418) ;
#6642=VERTEX_POINT('',#52420) ;
#6643=VERTEX_POINT('',#52422) ;
#6644=VERTEX_POINT('',#52426) ;
#6645=VERTEX_POINT('',#52427) ;
#6646=VERTEX_POINT('',#52429) ;
#6647=VERTEX_POINT('',#52431) ;
#6648=VERTEX_POINT('',#52435) ;
#6649=VERTEX_POINT('',#52436) ;
#6650=VERTEX_POINT('',#52438) ;
#6651=VERTEX_POINT('',#52440) ;
#6652=VERTEX_POINT('',#52444) ;
#6653=VERTEX_POINT('',#52445) ;
#6654=VERTEX_POINT('',#52447) ;
#6655=VERTEX_POINT('',#52449) ;
#6656=VERTEX_POINT('',#52453) ;
#6657=VERTEX_POINT('',#52454) ;
#6658=VERTEX_POINT('',#52456) ;
#6659=VERTEX_POINT('',#52458) ;
#6660=VERTEX_POINT('',#52462) ;
#6661=VERTEX_POINT('',#52463) ;
#6662=VERTEX_POINT('',#52465) ;
#6663=VERTEX_POINT('',#52467) ;
#6664=VERTEX_POINT('',#52471) ;
#6665=VERTEX_POINT('',#52472) ;
#6666=VERTEX_POINT('',#52474) ;
#6667=VERTEX_POINT('',#52476) ;
#6668=VERTEX_POINT('',#52480) ;
#6669=VERTEX_POINT('',#52481) ;
#6670=VERTEX_POINT('',#52483) ;
#6671=VERTEX_POINT('',#52485) ;
#6672=VERTEX_POINT('',#52489) ;
#6673=VERTEX_POINT('',#52490) ;
#6674=VERTEX_POINT('',#52492) ;
#6675=VERTEX_POINT('',#52494) ;
#6676=VERTEX_POINT('',#52498) ;
#6677=VERTEX_POINT('',#52499) ;
#6678=VERTEX_POINT('',#52501) ;
#6679=VERTEX_POINT('',#52503) ;
#6680=VERTEX_POINT('',#52507) ;
#6681=VERTEX_POINT('',#52508) ;
#6682=VERTEX_POINT('',#52510) ;
#6683=VERTEX_POINT('',#52512) ;
#6684=VERTEX_POINT('',#52516) ;
#6685=VERTEX_POINT('',#52520) ;
#6686=VERTEX_POINT('',#52523) ;
#6687=VERTEX_POINT('',#52525) ;
#6688=VERTEX_POINT('',#52529) ;
#6689=VERTEX_POINT('',#52530) ;
#6690=VERTEX_POINT('',#52535) ;
#6691=VERTEX_POINT('',#52599) ;
#6692=VERTEX_POINT('',#52600) ;
#6693=VERTEX_POINT('',#52603) ;
#6694=VERTEX_POINT('',#52667) ;
#6695=VERTEX_POINT('',#52669) ;
#6696=VERTEX_POINT('',#52673) ;
#6697=VERTEX_POINT('',#52677) ;
#6698=VERTEX_POINT('',#52680) ;
#6699=VERTEX_POINT('',#52684) ;
#6700=VERTEX_POINT('',#52687) ;
#6701=VERTEX_POINT('',#52693) ;
#6702=VERTEX_POINT('',#52695) ;
#6703=VERTEX_POINT('',#52699) ;
#6704=VERTEX_POINT('',#52701) ;
#6705=VERTEX_POINT('',#52710) ;
#6706=VERTEX_POINT('',#52712) ;
#6707=VERTEX_POINT('',#52716) ;
#6708=VERTEX_POINT('',#52718) ;
#6709=VERTEX_POINT('',#52727) ;
#6710=VERTEX_POINT('',#52729) ;
#6711=VERTEX_POINT('',#52733) ;
#6712=VERTEX_POINT('',#52735) ;
#6713=VERTEX_POINT('',#52744) ;
#6714=VERTEX_POINT('',#52746) ;
#6715=VERTEX_POINT('',#52750) ;
#6716=VERTEX_POINT('',#52752) ;
#6717=VERTEX_POINT('',#52761) ;
#6718=VERTEX_POINT('',#52763) ;
#6719=VERTEX_POINT('',#52767) ;
#6720=VERTEX_POINT('',#52769) ;
#6721=VERTEX_POINT('',#52778) ;
#6722=VERTEX_POINT('',#52780) ;
#6723=VERTEX_POINT('',#52784) ;
#6724=VERTEX_POINT('',#52786) ;
#6725=VERTEX_POINT('',#52795) ;
#6726=VERTEX_POINT('',#52797) ;
#6727=VERTEX_POINT('',#52801) ;
#6728=VERTEX_POINT('',#52803) ;
#6729=VERTEX_POINT('',#52812) ;
#6730=VERTEX_POINT('',#52814) ;
#6731=VERTEX_POINT('',#52818) ;
#6732=VERTEX_POINT('',#52820) ;
#6733=VERTEX_POINT('',#52829) ;
#6734=VERTEX_POINT('',#52831) ;
#6735=VERTEX_POINT('',#52835) ;
#6736=VERTEX_POINT('',#52837) ;
#6737=VERTEX_POINT('',#52846) ;
#6738=VERTEX_POINT('',#52848) ;
#6739=VERTEX_POINT('',#52852) ;
#6740=VERTEX_POINT('',#52854) ;
#6741=VERTEX_POINT('',#52863) ;
#6742=VERTEX_POINT('',#52865) ;
#6743=VERTEX_POINT('',#52869) ;
#6744=VERTEX_POINT('',#52871) ;
#6745=VERTEX_POINT('',#52880) ;
#6746=VERTEX_POINT('',#52882) ;
#6747=VERTEX_POINT('',#52886) ;
#6748=VERTEX_POINT('',#52888) ;
#6749=VERTEX_POINT('',#52897) ;
#6750=VERTEX_POINT('',#52899) ;
#6751=VERTEX_POINT('',#52903) ;
#6752=VERTEX_POINT('',#52905) ;
#6753=VERTEX_POINT('',#52914) ;
#6754=VERTEX_POINT('',#52916) ;
#6755=VERTEX_POINT('',#52920) ;
#6756=VERTEX_POINT('',#52922) ;
#6757=VERTEX_POINT('',#52931) ;
#6758=VERTEX_POINT('',#52933) ;
#6759=VERTEX_POINT('',#52937) ;
#6760=VERTEX_POINT('',#52939) ;
#6761=VERTEX_POINT('',#52948) ;
#6762=VERTEX_POINT('',#52950) ;
#6763=VERTEX_POINT('',#52954) ;
#6764=VERTEX_POINT('',#52956) ;
#6765=VERTEX_POINT('',#52965) ;
#6766=VERTEX_POINT('',#52967) ;
#6767=VERTEX_POINT('',#52971) ;
#6768=VERTEX_POINT('',#52973) ;
#6769=VERTEX_POINT('',#52982) ;
#6770=VERTEX_POINT('',#52984) ;
#6771=VERTEX_POINT('',#52988) ;
#6772=VERTEX_POINT('',#52990) ;
#6773=VERTEX_POINT('',#52999) ;
#6774=VERTEX_POINT('',#53001) ;
#6775=VERTEX_POINT('',#53005) ;
#6776=VERTEX_POINT('',#53007) ;
#6777=VERTEX_POINT('',#53016) ;
#6778=VERTEX_POINT('',#53018) ;
#6779=VERTEX_POINT('',#53022) ;
#6780=VERTEX_POINT('',#53024) ;
#6781=VERTEX_POINT('',#53033) ;
#6782=VERTEX_POINT('',#53035) ;
#6783=VERTEX_POINT('',#53039) ;
#6784=VERTEX_POINT('',#53041) ;
#6785=VERTEX_POINT('',#53050) ;
#6786=VERTEX_POINT('',#53052) ;
#6787=VERTEX_POINT('',#53056) ;
#6788=VERTEX_POINT('',#53058) ;
#6789=VERTEX_POINT('',#53067) ;
#6790=VERTEX_POINT('',#53069) ;
#6791=VERTEX_POINT('',#53073) ;
#6792=VERTEX_POINT('',#53075) ;
#6793=VERTEX_POINT('',#53084) ;
#6794=VERTEX_POINT('',#53086) ;
#6795=VERTEX_POINT('',#53090) ;
#6796=VERTEX_POINT('',#53092) ;
#6797=VERTEX_POINT('',#53101) ;
#6798=VERTEX_POINT('',#53103) ;
#6799=VERTEX_POINT('',#53107) ;
#6800=VERTEX_POINT('',#53109) ;
#6801=VERTEX_POINT('',#53118) ;
#6802=VERTEX_POINT('',#53120) ;
#6803=VERTEX_POINT('',#53124) ;
#6804=VERTEX_POINT('',#53126) ;
#6805=VERTEX_POINT('',#53135) ;
#6806=VERTEX_POINT('',#53137) ;
#6807=VERTEX_POINT('',#53141) ;
#6808=VERTEX_POINT('',#53143) ;
#6809=VERTEX_POINT('',#53152) ;
#6810=VERTEX_POINT('',#53154) ;
#6811=VERTEX_POINT('',#53158) ;
#6812=VERTEX_POINT('',#53160) ;
#6813=VERTEX_POINT('',#53169) ;
#6814=VERTEX_POINT('',#53171) ;
#6815=VERTEX_POINT('',#53175) ;
#6816=VERTEX_POINT('',#53177) ;
#6817=VERTEX_POINT('',#53186) ;
#6818=VERTEX_POINT('',#53188) ;
#6819=VERTEX_POINT('',#53192) ;
#6820=VERTEX_POINT('',#53194) ;
#6821=VERTEX_POINT('',#53203) ;
#6822=VERTEX_POINT('',#53205) ;
#6823=VERTEX_POINT('',#53209) ;
#6824=VERTEX_POINT('',#53211) ;
#6825=VERTEX_POINT('',#53220) ;
#6826=VERTEX_POINT('',#53222) ;
#6827=VERTEX_POINT('',#53226) ;
#6828=VERTEX_POINT('',#53228) ;
#6829=VERTEX_POINT('',#53237) ;
#6830=VERTEX_POINT('',#53239) ;
#6831=VERTEX_POINT('',#53243) ;
#6832=VERTEX_POINT('',#53245) ;
#6833=VERTEX_POINT('',#53254) ;
#6834=VERTEX_POINT('',#53256) ;
#6835=VERTEX_POINT('',#53260) ;
#6836=VERTEX_POINT('',#53262) ;
#6837=VERTEX_POINT('',#53271) ;
#6838=VERTEX_POINT('',#53273) ;
#6839=VERTEX_POINT('',#53277) ;
#6840=VERTEX_POINT('',#53279) ;
#6841=VERTEX_POINT('',#53288) ;
#6842=VERTEX_POINT('',#53290) ;
#6843=VERTEX_POINT('',#53294) ;
#6844=VERTEX_POINT('',#53296) ;
#6845=VERTEX_POINT('',#53305) ;
#6846=VERTEX_POINT('',#53307) ;
#6847=VERTEX_POINT('',#53311) ;
#6848=VERTEX_POINT('',#53313) ;
#6849=VERTEX_POINT('',#53322) ;
#6850=VERTEX_POINT('',#53324) ;
#6851=VERTEX_POINT('',#53328) ;
#6852=VERTEX_POINT('',#53330) ;
#6853=VERTEX_POINT('',#53339) ;
#6854=VERTEX_POINT('',#53341) ;
#6855=VERTEX_POINT('',#53345) ;
#6856=VERTEX_POINT('',#53347) ;
#6857=VERTEX_POINT('',#53356) ;
#6858=VERTEX_POINT('',#53358) ;
#6859=VERTEX_POINT('',#53362) ;
#6860=VERTEX_POINT('',#53364) ;
#6861=VERTEX_POINT('',#53373) ;
#6862=VERTEX_POINT('',#53375) ;
#6863=VERTEX_POINT('',#53379) ;
#6864=VERTEX_POINT('',#53381) ;
#6865=VERTEX_POINT('',#53390) ;
#6866=VERTEX_POINT('',#53392) ;
#6867=VERTEX_POINT('',#53396) ;
#6868=VERTEX_POINT('',#53398) ;
#6869=VERTEX_POINT('',#53407) ;
#6870=VERTEX_POINT('',#53409) ;
#6871=VERTEX_POINT('',#53413) ;
#6872=VERTEX_POINT('',#53415) ;
#6873=VERTEX_POINT('',#53424) ;
#6874=VERTEX_POINT('',#53426) ;
#6875=VERTEX_POINT('',#53430) ;
#6876=VERTEX_POINT('',#53432) ;
#6877=VERTEX_POINT('',#53441) ;
#6878=VERTEX_POINT('',#53443) ;
#6879=VERTEX_POINT('',#53447) ;
#6880=VERTEX_POINT('',#53449) ;
#6881=VERTEX_POINT('',#53458) ;
#6882=VERTEX_POINT('',#53460) ;
#6883=VERTEX_POINT('',#53464) ;
#6884=VERTEX_POINT('',#53466) ;
#6885=VERTEX_POINT('',#53475) ;
#6886=VERTEX_POINT('',#53477) ;
#6887=VERTEX_POINT('',#53481) ;
#6888=VERTEX_POINT('',#53483) ;
#6889=VERTEX_POINT('',#53492) ;
#6890=VERTEX_POINT('',#53494) ;
#6891=VERTEX_POINT('',#53498) ;
#6892=VERTEX_POINT('',#53500) ;
#6893=VERTEX_POINT('',#53509) ;
#6894=VERTEX_POINT('',#53511) ;
#6895=VERTEX_POINT('',#53515) ;
#6896=VERTEX_POINT('',#53517) ;
#6897=VERTEX_POINT('',#53526) ;
#6898=VERTEX_POINT('',#53528) ;
#6899=VERTEX_POINT('',#53532) ;
#6900=VERTEX_POINT('',#53534) ;
#6901=VERTEX_POINT('',#53543) ;
#6902=VERTEX_POINT('',#53545) ;
#6903=VERTEX_POINT('',#53549) ;
#6904=VERTEX_POINT('',#53551) ;
#6905=VERTEX_POINT('',#53560) ;
#6906=VERTEX_POINT('',#53562) ;
#6907=VERTEX_POINT('',#53566) ;
#6908=VERTEX_POINT('',#53568) ;
#6909=VERTEX_POINT('',#53577) ;
#6910=VERTEX_POINT('',#53579) ;
#6911=VERTEX_POINT('',#53583) ;
#6912=VERTEX_POINT('',#53585) ;
#6913=VERTEX_POINT('',#53594) ;
#6914=VERTEX_POINT('',#53596) ;
#6915=VERTEX_POINT('',#53600) ;
#6916=VERTEX_POINT('',#53602) ;
#6917=VERTEX_POINT('',#53611) ;
#6918=VERTEX_POINT('',#53613) ;
#6919=VERTEX_POINT('',#53617) ;
#6920=VERTEX_POINT('',#53619) ;
#6921=VERTEX_POINT('',#53628) ;
#6922=VERTEX_POINT('',#53630) ;
#6923=VERTEX_POINT('',#53634) ;
#6924=VERTEX_POINT('',#53636) ;
#6925=VERTEX_POINT('',#53645) ;
#6926=VERTEX_POINT('',#53647) ;
#6927=VERTEX_POINT('',#53651) ;
#6928=VERTEX_POINT('',#53653) ;
#6929=VERTEX_POINT('',#53662) ;
#6930=VERTEX_POINT('',#53664) ;
#6931=VERTEX_POINT('',#53668) ;
#6932=VERTEX_POINT('',#53670) ;
#6933=VERTEX_POINT('',#53679) ;
#6934=VERTEX_POINT('',#53681) ;
#6935=VERTEX_POINT('',#53685) ;
#6936=VERTEX_POINT('',#53687) ;
#6937=VERTEX_POINT('',#53696) ;
#6938=VERTEX_POINT('',#53698) ;
#6939=VERTEX_POINT('',#53702) ;
#6940=VERTEX_POINT('',#53704) ;
#8083=EDGE_CURVE('',#6435,#6436,#4964,.T.) ;
#8084=EDGE_CURVE('',#6437,#6435,#4965,.T.) ;
#8085=EDGE_CURVE('',#6437,#6438,#4966,.T.) ;
#8086=EDGE_CURVE('',#6436,#6438,#4967,.T.) ;
#8087=EDGE_CURVE('',#6439,#6437,#4968,.T.) ;
#8088=EDGE_CURVE('',#6439,#6440,#4969,.T.) ;
#8089=EDGE_CURVE('',#6438,#6440,#4970,.T.) ;
#8090=EDGE_CURVE('',#6441,#6442,#4971,.T.) ;
#8091=EDGE_CURVE('',#6440,#6441,#4972,.T.) ;
#8092=EDGE_CURVE('',#6442,#6439,#4973,.T.) ;
#8093=EDGE_CURVE('',#6443,#6443,#3709,.T.) ;
#8094=EDGE_CURVE('',#6435,#6442,#3710,.T.) ;
#8095=EDGE_CURVE('',#6444,#6445,#4974,.T.) ;
#8096=EDGE_CURVE('',#6446,#6444,#3711,.T.) ;
#8097=EDGE_CURVE('',#6446,#6447,#4975,.T.) ;
#8098=EDGE_CURVE('',#6447,#6445,#3712,.T.) ;
#8099=EDGE_CURVE('',#6448,#6449,#3713,.T.) ;
#8100=EDGE_CURVE('',#6448,#6450,#4976,.T.) ;
#8101=EDGE_CURVE('',#6450,#6451,#3714,.T.) ;
#8102=EDGE_CURVE('',#6449,#6451,#4977,.T.) ;
#8103=EDGE_CURVE('',#6452,#6453,#3715,.T.) ;
#8104=EDGE_CURVE('',#6452,#6454,#4978,.T.) ;
#8105=EDGE_CURVE('',#6454,#6455,#3716,.T.) ;
#8106=EDGE_CURVE('',#6453,#6455,#4979,.T.) ;
#8107=EDGE_CURVE('',#6456,#6457,#3717,.T.) ;
#8108=EDGE_CURVE('',#6456,#6458,#4980,.T.) ;
#8109=EDGE_CURVE('',#6458,#6459,#3718,.T.) ;
#8110=EDGE_CURVE('',#6457,#6459,#4981,.T.) ;
#8111=EDGE_CURVE('',#6460,#6461,#4982,.T.) ;
#8112=EDGE_CURVE('',#6462,#6460,#3719,.T.) ;
#8113=EDGE_CURVE('',#6462,#6463,#4983,.T.) ;
#8114=EDGE_CURVE('',#6463,#6461,#3720,.T.) ;
#8115=EDGE_CURVE('',#6464,#6465,#4984,.T.) ;
#8116=EDGE_CURVE('',#6466,#6464,#3721,.T.) ;
#8117=EDGE_CURVE('',#6466,#6467,#4985,.T.) ;
#8118=EDGE_CURVE('',#6467,#6465,#3722,.T.) ;
#8119=EDGE_CURVE('',#6468,#6469,#4986,.T.) ;
#8120=EDGE_CURVE('',#6470,#6468,#3723,.T.) ;
#8121=EDGE_CURVE('',#6470,#6471,#4987,.T.) ;
#8122=EDGE_CURVE('',#6471,#6469,#3724,.T.) ;
#8123=EDGE_CURVE('',#6472,#6473,#3725,.T.) ;
#8124=EDGE_CURVE('',#6472,#6474,#4988,.T.) ;
#8125=EDGE_CURVE('',#6474,#6475,#3726,.T.) ;
#8126=EDGE_CURVE('',#6473,#6475,#4989,.T.) ;
#8127=EDGE_CURVE('',#6476,#6477,#3727,.T.) ;
#8128=EDGE_CURVE('',#6476,#6478,#4990,.T.) ;
#8129=EDGE_CURVE('',#6478,#6479,#3728,.T.) ;
#8130=EDGE_CURVE('',#6477,#6479,#4991,.T.) ;
#8131=EDGE_CURVE('',#6480,#6481,#3729,.T.) ;
#8132=EDGE_CURVE('',#6480,#6482,#4992,.T.) ;
#8133=EDGE_CURVE('',#6482,#6483,#3730,.T.) ;
#8134=EDGE_CURVE('',#6481,#6483,#4993,.T.) ;
#8135=EDGE_CURVE('',#6484,#6485,#3731,.T.) ;
#8136=EDGE_CURVE('',#6484,#6486,#4994,.T.) ;
#8137=EDGE_CURVE('',#6486,#6487,#3732,.T.) ;
#8138=EDGE_CURVE('',#6485,#6487,#4995,.T.) ;
#8139=EDGE_CURVE('',#6488,#6489,#3733,.T.) ;
#8140=EDGE_CURVE('',#6488,#6490,#4996,.T.) ;
#8141=EDGE_CURVE('',#6490,#6491,#3734,.T.) ;
#8142=EDGE_CURVE('',#6489,#6491,#4997,.T.) ;
#8143=EDGE_CURVE('',#6492,#6493,#3735,.T.) ;
#8144=EDGE_CURVE('',#6492,#6494,#4998,.T.) ;
#8145=EDGE_CURVE('',#6494,#6495,#3736,.T.) ;
#8146=EDGE_CURVE('',#6493,#6495,#4999,.T.) ;
#8147=EDGE_CURVE('',#6496,#6497,#3737,.T.) ;
#8148=EDGE_CURVE('',#6496,#6498,#5000,.T.) ;
#8149=EDGE_CURVE('',#6498,#6499,#3738,.T.) ;
#8150=EDGE_CURVE('',#6497,#6499,#5001,.T.) ;
#8151=EDGE_CURVE('',#6500,#6501,#3739,.T.) ;
#8152=EDGE_CURVE('',#6500,#6502,#5002,.T.) ;
#8153=EDGE_CURVE('',#6502,#6503,#3740,.T.) ;
#8154=EDGE_CURVE('',#6501,#6503,#5003,.T.) ;
#8155=EDGE_CURVE('',#6504,#6505,#3741,.T.) ;
#8156=EDGE_CURVE('',#6504,#6506,#5004,.T.) ;
#8157=EDGE_CURVE('',#6506,#6507,#3742,.T.) ;
#8158=EDGE_CURVE('',#6505,#6507,#5005,.T.) ;
#8159=EDGE_CURVE('',#6508,#6509,#3743,.T.) ;
#8160=EDGE_CURVE('',#6508,#6510,#5006,.T.) ;
#8161=EDGE_CURVE('',#6510,#6511,#3744,.T.) ;
#8162=EDGE_CURVE('',#6509,#6511,#5007,.T.) ;
#8163=EDGE_CURVE('',#6512,#6513,#3745,.T.) ;
#8164=EDGE_CURVE('',#6512,#6514,#5008,.T.) ;
#8165=EDGE_CURVE('',#6514,#6515,#3746,.T.) ;
#8166=EDGE_CURVE('',#6513,#6515,#5009,.T.) ;
#8167=EDGE_CURVE('',#6516,#6517,#3747,.T.) ;
#8168=EDGE_CURVE('',#6516,#6518,#5010,.T.) ;
#8169=EDGE_CURVE('',#6518,#6519,#3748,.T.) ;
#8170=EDGE_CURVE('',#6517,#6519,#5011,.T.) ;
#8171=EDGE_CURVE('',#6520,#6521,#3749,.T.) ;
#8172=EDGE_CURVE('',#6520,#6522,#5012,.T.) ;
#8173=EDGE_CURVE('',#6522,#6523,#3750,.T.) ;
#8174=EDGE_CURVE('',#6521,#6523,#5013,.T.) ;
#8175=EDGE_CURVE('',#6524,#6525,#5014,.T.) ;
#8176=EDGE_CURVE('',#6526,#6524,#3751,.T.) ;
#8177=EDGE_CURVE('',#6526,#6527,#5015,.T.) ;
#8178=EDGE_CURVE('',#6527,#6525,#3752,.T.) ;
#8179=EDGE_CURVE('',#6528,#6529,#3753,.T.) ;
#8180=EDGE_CURVE('',#6528,#6530,#5016,.T.) ;
#8181=EDGE_CURVE('',#6530,#6531,#3754,.T.) ;
#8182=EDGE_CURVE('',#6529,#6531,#5017,.T.) ;
#8183=EDGE_CURVE('',#6532,#6533,#3755,.T.) ;
#8184=EDGE_CURVE('',#6532,#6534,#5018,.T.) ;
#8185=EDGE_CURVE('',#6534,#6535,#3756,.T.) ;
#8186=EDGE_CURVE('',#6533,#6535,#5019,.T.) ;
#8187=EDGE_CURVE('',#6536,#6537,#3757,.T.) ;
#8188=EDGE_CURVE('',#6536,#6538,#5020,.T.) ;
#8189=EDGE_CURVE('',#6538,#6539,#3758,.T.) ;
#8190=EDGE_CURVE('',#6537,#6539,#5021,.T.) ;
#8191=EDGE_CURVE('',#6540,#6541,#3759,.T.) ;
#8192=EDGE_CURVE('',#6540,#6542,#5022,.T.) ;
#8193=EDGE_CURVE('',#6542,#6543,#3760,.T.) ;
#8194=EDGE_CURVE('',#6541,#6543,#5023,.T.) ;
#8195=EDGE_CURVE('',#6544,#6545,#3761,.T.) ;
#8196=EDGE_CURVE('',#6544,#6546,#5024,.T.) ;
#8197=EDGE_CURVE('',#6546,#6547,#3762,.T.) ;
#8198=EDGE_CURVE('',#6545,#6547,#5025,.T.) ;
#8199=EDGE_CURVE('',#6548,#6549,#3763,.T.) ;
#8200=EDGE_CURVE('',#6548,#6550,#5026,.T.) ;
#8201=EDGE_CURVE('',#6550,#6551,#3764,.T.) ;
#8202=EDGE_CURVE('',#6549,#6551,#5027,.T.) ;
#8203=EDGE_CURVE('',#6552,#6553,#3765,.T.) ;
#8204=EDGE_CURVE('',#6552,#6554,#5028,.T.) ;
#8205=EDGE_CURVE('',#6554,#6555,#3766,.T.) ;
#8206=EDGE_CURVE('',#6553,#6555,#5029,.T.) ;
#8207=EDGE_CURVE('',#6556,#6557,#3767,.T.) ;
#8208=EDGE_CURVE('',#6556,#6558,#5030,.T.) ;
#8209=EDGE_CURVE('',#6558,#6559,#3768,.T.) ;
#8210=EDGE_CURVE('',#6557,#6559,#5031,.T.) ;
#8211=EDGE_CURVE('',#6560,#6561,#3769,.T.) ;
#8212=EDGE_CURVE('',#6560,#6562,#5032,.T.) ;
#8213=EDGE_CURVE('',#6562,#6563,#3770,.T.) ;
#8214=EDGE_CURVE('',#6561,#6563,#5033,.T.) ;
#8215=EDGE_CURVE('',#6564,#6565,#3771,.T.) ;
#8216=EDGE_CURVE('',#6564,#6566,#5034,.T.) ;
#8217=EDGE_CURVE('',#6566,#6567,#3772,.T.) ;
#8218=EDGE_CURVE('',#6565,#6567,#5035,.T.) ;
#8219=EDGE_CURVE('',#6568,#6569,#3773,.T.) ;
#8220=EDGE_CURVE('',#6568,#6570,#5036,.T.) ;
#8221=EDGE_CURVE('',#6570,#6571,#3774,.T.) ;
#8222=EDGE_CURVE('',#6569,#6571,#5037,.T.) ;
#8223=EDGE_CURVE('',#6572,#6573,#5038,.T.) ;
#8224=EDGE_CURVE('',#6574,#6572,#3775,.T.) ;
#8225=EDGE_CURVE('',#6574,#6575,#5039,.T.) ;
#8226=EDGE_CURVE('',#6575,#6573,#3776,.T.) ;
#8227=EDGE_CURVE('',#6576,#6577,#5040,.T.) ;
#8228=EDGE_CURVE('',#6578,#6576,#3777,.T.) ;
#8229=EDGE_CURVE('',#6578,#6579,#5041,.T.) ;
#8230=EDGE_CURVE('',#6579,#6577,#3778,.T.) ;
#8231=EDGE_CURVE('',#6580,#6581,#5042,.T.) ;
#8232=EDGE_CURVE('',#6582,#6580,#3779,.T.) ;
#8233=EDGE_CURVE('',#6582,#6583,#5043,.T.) ;
#8234=EDGE_CURVE('',#6583,#6581,#3780,.T.) ;
#8235=EDGE_CURVE('',#6584,#6585,#5044,.T.) ;
#8236=EDGE_CURVE('',#6586,#6584,#3781,.T.) ;
#8237=EDGE_CURVE('',#6586,#6587,#5045,.T.) ;
#8238=EDGE_CURVE('',#6587,#6585,#3782,.T.) ;
#8239=EDGE_CURVE('',#6588,#6589,#5046,.T.) ;
#8240=EDGE_CURVE('',#6590,#6588,#3783,.T.) ;
#8241=EDGE_CURVE('',#6590,#6591,#5047,.T.) ;
#8242=EDGE_CURVE('',#6591,#6589,#3784,.T.) ;
#8243=EDGE_CURVE('',#6592,#6593,#5048,.T.) ;
#8244=EDGE_CURVE('',#6594,#6592,#3785,.T.) ;
#8245=EDGE_CURVE('',#6594,#6595,#5049,.T.) ;
#8246=EDGE_CURVE('',#6595,#6593,#3786,.T.) ;
#8247=EDGE_CURVE('',#6596,#6597,#5050,.T.) ;
#8248=EDGE_CURVE('',#6598,#6596,#3787,.T.) ;
#8249=EDGE_CURVE('',#6598,#6599,#5051,.T.) ;
#8250=EDGE_CURVE('',#6599,#6597,#3788,.T.) ;
#8251=EDGE_CURVE('',#6600,#6601,#3789,.T.) ;
#8252=EDGE_CURVE('',#6600,#6602,#5052,.T.) ;
#8253=EDGE_CURVE('',#6602,#6603,#3790,.T.) ;
#8254=EDGE_CURVE('',#6601,#6603,#5053,.T.) ;
#8255=EDGE_CURVE('',#6604,#6605,#3791,.T.) ;
#8256=EDGE_CURVE('',#6604,#6606,#5054,.T.) ;
#8257=EDGE_CURVE('',#6606,#6607,#3792,.T.) ;
#8258=EDGE_CURVE('',#6605,#6607,#5055,.T.) ;
#8259=EDGE_CURVE('',#6608,#6609,#3793,.T.) ;
#8260=EDGE_CURVE('',#6608,#6610,#5056,.T.) ;
#8261=EDGE_CURVE('',#6610,#6611,#3794,.T.) ;
#8262=EDGE_CURVE('',#6609,#6611,#5057,.T.) ;
#8263=EDGE_CURVE('',#6612,#6613,#3795,.T.) ;
#8264=EDGE_CURVE('',#6612,#6614,#5058,.T.) ;
#8265=EDGE_CURVE('',#6614,#6615,#3796,.T.) ;
#8266=EDGE_CURVE('',#6613,#6615,#5059,.T.) ;
#8267=EDGE_CURVE('',#6616,#6617,#3797,.T.) ;
#8268=EDGE_CURVE('',#6616,#6618,#5060,.T.) ;
#8269=EDGE_CURVE('',#6618,#6619,#3798,.T.) ;
#8270=EDGE_CURVE('',#6617,#6619,#5061,.T.) ;
#8271=EDGE_CURVE('',#6620,#6621,#3799,.T.) ;
#8272=EDGE_CURVE('',#6620,#6622,#5062,.T.) ;
#8273=EDGE_CURVE('',#6622,#6623,#3800,.T.) ;
#8274=EDGE_CURVE('',#6621,#6623,#5063,.T.) ;
#8275=EDGE_CURVE('',#6624,#6625,#3801,.T.) ;
#8276=EDGE_CURVE('',#6624,#6626,#5064,.T.) ;
#8277=EDGE_CURVE('',#6626,#6627,#3802,.T.) ;
#8278=EDGE_CURVE('',#6625,#6627,#5065,.T.) ;
#8279=EDGE_CURVE('',#6628,#6629,#3803,.T.) ;
#8280=EDGE_CURVE('',#6628,#6630,#5066,.T.) ;
#8281=EDGE_CURVE('',#6630,#6631,#3804,.T.) ;
#8282=EDGE_CURVE('',#6629,#6631,#5067,.T.) ;
#8283=EDGE_CURVE('',#6632,#6633,#3805,.T.) ;
#8284=EDGE_CURVE('',#6632,#6634,#5068,.T.) ;
#8285=EDGE_CURVE('',#6634,#6635,#3806,.T.) ;
#8286=EDGE_CURVE('',#6633,#6635,#5069,.T.) ;
#8287=EDGE_CURVE('',#6636,#6637,#3807,.T.) ;
#8288=EDGE_CURVE('',#6636,#6638,#5070,.T.) ;
#8289=EDGE_CURVE('',#6638,#6639,#3808,.T.) ;
#8290=EDGE_CURVE('',#6637,#6639,#5071,.T.) ;
#8291=EDGE_CURVE('',#6640,#6641,#3809,.T.) ;
#8292=EDGE_CURVE('',#6640,#6642,#5072,.T.) ;
#8293=EDGE_CURVE('',#6642,#6643,#3810,.T.) ;
#8294=EDGE_CURVE('',#6641,#6643,#5073,.T.) ;
#8295=EDGE_CURVE('',#6644,#6645,#5074,.T.) ;
#8296=EDGE_CURVE('',#6646,#6644,#3811,.T.) ;
#8297=EDGE_CURVE('',#6646,#6647,#5075,.T.) ;
#8298=EDGE_CURVE('',#6647,#6645,#3812,.T.) ;
#8299=EDGE_CURVE('',#6648,#6649,#3813,.T.) ;
#8300=EDGE_CURVE('',#6648,#6650,#5076,.T.) ;
#8301=EDGE_CURVE('',#6650,#6651,#3814,.T.) ;
#8302=EDGE_CURVE('',#6649,#6651,#5077,.T.) ;
#8303=EDGE_CURVE('',#6652,#6653,#3815,.T.) ;
#8304=EDGE_CURVE('',#6652,#6654,#5078,.T.) ;
#8305=EDGE_CURVE('',#6654,#6655,#3816,.T.) ;
#8306=EDGE_CURVE('',#6653,#6655,#5079,.T.) ;
#8307=EDGE_CURVE('',#6656,#6657,#3817,.T.) ;
#8308=EDGE_CURVE('',#6656,#6658,#5080,.T.) ;
#8309=EDGE_CURVE('',#6658,#6659,#3818,.T.) ;
#8310=EDGE_CURVE('',#6657,#6659,#5081,.T.) ;
#8311=EDGE_CURVE('',#6660,#6661,#3819,.T.) ;
#8312=EDGE_CURVE('',#6660,#6662,#5082,.T.) ;
#8313=EDGE_CURVE('',#6662,#6663,#3820,.T.) ;
#8314=EDGE_CURVE('',#6661,#6663,#5083,.T.) ;
#8315=EDGE_CURVE('',#6664,#6665,#3821,.T.) ;
#8316=EDGE_CURVE('',#6664,#6666,#5084,.T.) ;
#8317=EDGE_CURVE('',#6666,#6667,#3822,.T.) ;
#8318=EDGE_CURVE('',#6665,#6667,#5085,.T.) ;
#8319=EDGE_CURVE('',#6668,#6669,#3823,.T.) ;
#8320=EDGE_CURVE('',#6668,#6670,#5086,.T.) ;
#8321=EDGE_CURVE('',#6670,#6671,#3824,.T.) ;
#8322=EDGE_CURVE('',#6669,#6671,#5087,.T.) ;
#8323=EDGE_CURVE('',#6672,#6673,#3825,.T.) ;
#8324=EDGE_CURVE('',#6672,#6674,#5088,.T.) ;
#8325=EDGE_CURVE('',#6674,#6675,#3826,.T.) ;
#8326=EDGE_CURVE('',#6673,#6675,#5089,.T.) ;
#8327=EDGE_CURVE('',#6676,#6677,#5090,.T.) ;
#8328=EDGE_CURVE('',#6678,#6676,#3827,.T.) ;
#8329=EDGE_CURVE('',#6678,#6679,#5091,.T.) ;
#8330=EDGE_CURVE('',#6679,#6677,#3828,.T.) ;
#8331=EDGE_CURVE('',#6680,#6681,#3829,.T.) ;
#8332=EDGE_CURVE('',#6680,#6682,#5092,.T.) ;
#8333=EDGE_CURVE('',#6682,#6683,#3830,.T.) ;
#8334=EDGE_CURVE('',#6681,#6683,#5093,.T.) ;
#8335=EDGE_CURVE('',#6684,#6684,#3831,.T.) ;
#8336=EDGE_CURVE('',#6684,#6443,#5094,.T.) ;
#8337=EDGE_CURVE('',#6685,#6685,#3832,.T.) ;
#8338=EDGE_CURVE('',#6685,#6686,#5095,.T.) ;
#8339=EDGE_CURVE('',#6687,#6686,#3833,.T.) ;
#8340=EDGE_CURVE('',#6686,#6687,#3834,.T.) ;
#8341=EDGE_CURVE('',#6688,#6689,#3835,.T.) ;
#8342=EDGE_CURVE('',#6689,#6688,#3836,.T.) ;
#8343=EDGE_CURVE('',#6689,#6687,#5096,.T.) ;
#8344=EDGE_CURVE('',#6688,#6690,#5097,.T.) ;
#8345=EDGE_CURVE('',#6619,#6690,#3837,.T.) ;
#8346=EDGE_CURVE('',#6615,#6618,#3838,.T.) ;
#8347=EDGE_CURVE('',#6611,#6614,#3839,.T.) ;
#8348=EDGE_CURVE('',#6607,#6610,#3840,.T.) ;
#8349=EDGE_CURVE('',#6573,#6606,#3841,.T.) ;
#8350=EDGE_CURVE('',#6577,#6575,#3842,.T.) ;
#8351=EDGE_CURVE('',#6581,#6579,#3843,.T.) ;
#8352=EDGE_CURVE('',#6585,#6583,#3844,.T.) ;
#8353=EDGE_CURVE('',#6589,#6587,#3845,.T.) ;
#8354=EDGE_CURVE('',#6593,#6591,#3846,.T.) ;
#8355=EDGE_CURVE('',#6597,#6595,#3847,.T.) ;
#8356=EDGE_CURVE('',#6603,#6599,#3848,.T.) ;
#8357=EDGE_CURVE('',#6571,#6602,#3849,.T.) ;
#8358=EDGE_CURVE('',#6567,#6570,#3850,.T.) ;
#8359=EDGE_CURVE('',#6563,#6566,#3851,.T.) ;
#8360=EDGE_CURVE('',#6559,#6562,#3852,.T.) ;
#8361=EDGE_CURVE('',#6555,#6558,#3853,.T.) ;
#8362=EDGE_CURVE('',#6551,#6554,#3854,.T.) ;
#8363=EDGE_CURVE('',#6547,#6550,#3855,.T.) ;
#8364=EDGE_CURVE('',#6543,#6546,#3856,.T.) ;
#8365=EDGE_CURVE('',#6539,#6542,#3857,.T.) ;
#8366=EDGE_CURVE('',#6535,#6538,#3858,.T.) ;
#8367=EDGE_CURVE('',#6525,#6534,#3859,.T.) ;
#8368=EDGE_CURVE('',#6531,#6527,#3860,.T.) ;
#8369=EDGE_CURVE('',#6523,#6530,#3861,.T.) ;
#8370=EDGE_CURVE('',#6519,#6522,#3862,.T.) ;
#8371=EDGE_CURVE('',#6515,#6518,#3863,.T.) ;
#8372=EDGE_CURVE('',#6511,#6514,#3864,.T.) ;
#8373=EDGE_CURVE('',#6507,#6510,#3865,.T.) ;
#8374=EDGE_CURVE('',#6503,#6506,#3866,.T.) ;
#8375=EDGE_CURVE('',#6499,#6502,#3867,.T.) ;
#8376=EDGE_CURVE('',#6495,#6498,#3868,.T.) ;
#8377=EDGE_CURVE('',#6491,#6494,#3869,.T.) ;
#8378=EDGE_CURVE('',#6487,#6490,#3870,.T.) ;
#8379=EDGE_CURVE('',#6483,#6486,#3871,.T.) ;
#8380=EDGE_CURVE('',#6479,#6482,#3872,.T.) ;
#8381=EDGE_CURVE('',#6461,#6478,#3873,.T.) ;
#8382=EDGE_CURVE('',#6465,#6463,#3874,.T.) ;
#8383=EDGE_CURVE('',#6469,#6467,#3875,.T.) ;
#8384=EDGE_CURVE('',#6475,#6471,#3876,.T.) ;
#8385=EDGE_CURVE('',#6459,#6474,#3877,.T.) ;
#8386=EDGE_CURVE('',#6455,#6458,#3878,.T.) ;
#8387=EDGE_CURVE('',#6451,#6454,#3879,.T.) ;
#8388=EDGE_CURVE('',#6445,#6450,#3880,.T.) ;
#8389=EDGE_CURVE('',#6677,#6447,#3881,.T.) ;
#8390=EDGE_CURVE('',#6683,#6679,#3882,.T.) ;
#8391=EDGE_CURVE('',#6675,#6682,#3883,.T.) ;
#8392=EDGE_CURVE('',#6671,#6674,#3884,.T.) ;
#8393=EDGE_CURVE('',#6667,#6670,#3885,.T.) ;
#8394=EDGE_CURVE('',#6663,#6666,#3886,.T.) ;
#8395=EDGE_CURVE('',#6659,#6662,#3887,.T.) ;
#8396=EDGE_CURVE('',#6655,#6658,#3888,.T.) ;
#8397=EDGE_CURVE('',#6645,#6654,#3889,.T.) ;
#8398=EDGE_CURVE('',#6651,#6647,#3890,.T.) ;
#8399=EDGE_CURVE('',#6643,#6650,#3891,.T.) ;
#8400=EDGE_CURVE('',#6639,#6642,#3892,.T.) ;
#8401=EDGE_CURVE('',#6635,#6638,#3893,.T.) ;
#8402=EDGE_CURVE('',#6631,#6634,#3894,.T.) ;
#8403=EDGE_CURVE('',#6627,#6630,#3895,.T.) ;
#8404=EDGE_CURVE('',#6623,#6626,#3896,.T.) ;
#8405=EDGE_CURVE('',#6690,#6622,#3897,.T.) ;
#8406=EDGE_CURVE('',#6691,#6692,#3898,.T.) ;
#8407=EDGE_CURVE('',#6692,#6691,#3899,.T.) ;
#8408=EDGE_CURVE('',#6692,#6693,#5098,.T.) ;
#8409=EDGE_CURVE('',#6693,#6500,#3900,.T.) ;
#8410=EDGE_CURVE('',#6501,#6504,#3901,.T.) ;
#8411=EDGE_CURVE('',#6505,#6508,#3902,.T.) ;
#8412=EDGE_CURVE('',#6509,#6512,#3903,.T.) ;
#8413=EDGE_CURVE('',#6513,#6516,#3904,.T.) ;
#8414=EDGE_CURVE('',#6517,#6520,#3905,.T.) ;
#8415=EDGE_CURVE('',#6521,#6528,#3906,.T.) ;
#8416=EDGE_CURVE('',#6529,#6526,#3907,.T.) ;
#8417=EDGE_CURVE('',#6524,#6532,#3908,.T.) ;
#8418=EDGE_CURVE('',#6533,#6536,#3909,.T.) ;
#8419=EDGE_CURVE('',#6537,#6540,#3910,.T.) ;
#8420=EDGE_CURVE('',#6541,#6544,#3911,.T.) ;
#8421=EDGE_CURVE('',#6545,#6548,#3912,.T.) ;
#8422=EDGE_CURVE('',#6549,#6552,#3913,.T.) ;
#8423=EDGE_CURVE('',#6553,#6556,#3914,.T.) ;
#8424=EDGE_CURVE('',#6557,#6560,#3915,.T.) ;
#8425=EDGE_CURVE('',#6561,#6564,#3916,.T.) ;
#8426=EDGE_CURVE('',#6565,#6568,#3917,.T.) ;
#8427=EDGE_CURVE('',#6569,#6600,#3918,.T.) ;
#8428=EDGE_CURVE('',#6601,#6598,#3919,.T.) ;
#8429=EDGE_CURVE('',#6596,#6594,#3920,.T.) ;
#8430=EDGE_CURVE('',#6592,#6590,#3921,.T.) ;
#8431=EDGE_CURVE('',#6588,#6586,#3922,.T.) ;
#8432=EDGE_CURVE('',#6584,#6582,#3923,.T.) ;
#8433=EDGE_CURVE('',#6580,#6578,#3924,.T.) ;
#8434=EDGE_CURVE('',#6576,#6574,#3925,.T.) ;
#8435=EDGE_CURVE('',#6572,#6604,#3926,.T.) ;
#8436=EDGE_CURVE('',#6605,#6608,#3927,.T.) ;
#8437=EDGE_CURVE('',#6609,#6612,#3928,.T.) ;
#8438=EDGE_CURVE('',#6613,#6616,#3929,.T.) ;
#8439=EDGE_CURVE('',#6617,#6620,#3930,.T.) ;
#8440=EDGE_CURVE('',#6621,#6624,#3931,.T.) ;
#8441=EDGE_CURVE('',#6625,#6628,#3932,.T.) ;
#8442=EDGE_CURVE('',#6629,#6632,#3933,.T.) ;
#8443=EDGE_CURVE('',#6633,#6636,#3934,.T.) ;
#8444=EDGE_CURVE('',#6637,#6640,#3935,.T.) ;
#8445=EDGE_CURVE('',#6641,#6648,#3936,.T.) ;
#8446=EDGE_CURVE('',#6649,#6646,#3937,.T.) ;
#8447=EDGE_CURVE('',#6644,#6652,#3938,.T.) ;
#8448=EDGE_CURVE('',#6653,#6656,#3939,.T.) ;
#8449=EDGE_CURVE('',#6657,#6660,#3940,.T.) ;
#8450=EDGE_CURVE('',#6661,#6664,#3941,.T.) ;
#8451=EDGE_CURVE('',#6665,#6668,#3942,.T.) ;
#8452=EDGE_CURVE('',#6669,#6672,#3943,.T.) ;
#8453=EDGE_CURVE('',#6673,#6680,#3944,.T.) ;
#8454=EDGE_CURVE('',#6681,#6678,#3945,.T.) ;
#8455=EDGE_CURVE('',#6676,#6446,#3946,.T.) ;
#8456=EDGE_CURVE('',#6444,#6448,#3947,.T.) ;
#8457=EDGE_CURVE('',#6449,#6452,#3948,.T.) ;
#8458=EDGE_CURVE('',#6453,#6456,#3949,.T.) ;
#8459=EDGE_CURVE('',#6457,#6472,#3950,.T.) ;
#8460=EDGE_CURVE('',#6473,#6470,#3951,.T.) ;
#8461=EDGE_CURVE('',#6468,#6466,#3952,.T.) ;
#8462=EDGE_CURVE('',#6464,#6462,#3953,.T.) ;
#8463=EDGE_CURVE('',#6460,#6476,#3954,.T.) ;
#8464=EDGE_CURVE('',#6477,#6480,#3955,.T.) ;
#8465=EDGE_CURVE('',#6481,#6484,#3956,.T.) ;
#8466=EDGE_CURVE('',#6485,#6488,#3957,.T.) ;
#8467=EDGE_CURVE('',#6489,#6492,#3958,.T.) ;
#8468=EDGE_CURVE('',#6493,#6496,#3959,.T.) ;
#8469=EDGE_CURVE('',#6497,#6693,#3960,.T.) ;
#8470=EDGE_CURVE('',#6691,#6694,#5099,.T.) ;
#8471=EDGE_CURVE('',#6695,#6694,#3961,.T.) ;
#8472=EDGE_CURVE('',#6694,#6695,#3962,.T.) ;
#8473=EDGE_CURVE('',#6696,#6696,#3963,.T.) ;
#8474=EDGE_CURVE('',#6696,#6695,#5100,.T.) ;
#8475=EDGE_CURVE('',#6697,#6697,#3964,.T.) ;
#8476=EDGE_CURVE('',#6698,#6698,#3965,.T.) ;
#8477=EDGE_CURVE('',#6698,#6697,#5101,.T.) ;
#8478=EDGE_CURVE('',#6699,#6699,#3966,.T.) ;
#8479=EDGE_CURVE('',#6700,#6700,#3967,.T.) ;
#8480=EDGE_CURVE('',#6700,#6699,#5102,.T.) ;
#8481=EDGE_CURVE('',#6436,#6441,#3968,.T.) ;
#8482=EDGE_CURVE('',#6683,#6701,#3969,.T.) ;
#8483=EDGE_CURVE('',#6702,#6679,#3970,.T.) ;
#8484=EDGE_CURVE('',#6702,#6701,#3971,.T.) ;
#8485=EDGE_CURVE('',#6681,#6703,#3972,.T.) ;
#8486=EDGE_CURVE('',#6704,#6703,#3973,.T.) ;
#8487=EDGE_CURVE('',#6704,#6678,#3974,.T.) ;
#8488=EDGE_CURVE('',#6704,#6702,#5103,.T.) ;
#8489=EDGE_CURVE('',#6703,#6701,#5104,.T.) ;
#8490=EDGE_CURVE('',#6705,#6447,#3975,.T.) ;
#8491=EDGE_CURVE('',#6705,#6706,#3976,.T.) ;
#8492=EDGE_CURVE('',#6677,#6706,#3977,.T.) ;
#8493=EDGE_CURVE('',#6676,#6707,#3978,.T.) ;
#8494=EDGE_CURVE('',#6708,#6707,#3979,.T.) ;
#8495=EDGE_CURVE('',#6708,#6446,#3980,.T.) ;
#8496=EDGE_CURVE('',#6708,#6705,#5105,.T.) ;
#8497=EDGE_CURVE('',#6707,#6706,#5106,.T.) ;
#8498=EDGE_CURVE('',#6709,#6682,#3981,.T.) ;
#8499=EDGE_CURVE('',#6709,#6710,#3982,.T.) ;
#8500=EDGE_CURVE('',#6675,#6710,#3983,.T.) ;
#8501=EDGE_CURVE('',#6673,#6711,#3984,.T.) ;
#8502=EDGE_CURVE('',#6712,#6711,#3985,.T.) ;
#8503=EDGE_CURVE('',#6712,#6680,#3986,.T.) ;
#8504=EDGE_CURVE('',#6712,#6709,#5107,.T.) ;
#8505=EDGE_CURVE('',#6711,#6710,#5108,.T.) ;
#8506=EDGE_CURVE('',#6713,#6674,#3987,.T.) ;
#8507=EDGE_CURVE('',#6713,#6714,#3988,.T.) ;
#8508=EDGE_CURVE('',#6671,#6714,#3989,.T.) ;
#8509=EDGE_CURVE('',#6669,#6715,#3990,.T.) ;
#8510=EDGE_CURVE('',#6716,#6715,#3991,.T.) ;
#8511=EDGE_CURVE('',#6716,#6672,#3992,.T.) ;
#8512=EDGE_CURVE('',#6716,#6713,#5109,.T.) ;
#8513=EDGE_CURVE('',#6715,#6714,#5110,.T.) ;
#8514=EDGE_CURVE('',#6717,#6670,#3993,.T.) ;
#8515=EDGE_CURVE('',#6717,#6718,#3994,.T.) ;
#8516=EDGE_CURVE('',#6667,#6718,#3995,.T.) ;
#8517=EDGE_CURVE('',#6665,#6719,#3996,.T.) ;
#8518=EDGE_CURVE('',#6720,#6719,#3997,.T.) ;
#8519=EDGE_CURVE('',#6720,#6668,#3998,.T.) ;
#8520=EDGE_CURVE('',#6720,#6717,#5111,.T.) ;
#8521=EDGE_CURVE('',#6719,#6718,#5112,.T.) ;
#8522=EDGE_CURVE('',#6721,#6666,#3999,.T.) ;
#8523=EDGE_CURVE('',#6721,#6722,#4000,.T.) ;
#8524=EDGE_CURVE('',#6663,#6722,#4001,.T.) ;
#8525=EDGE_CURVE('',#6661,#6723,#4002,.T.) ;
#8526=EDGE_CURVE('',#6724,#6723,#4003,.T.) ;
#8527=EDGE_CURVE('',#6724,#6664,#4004,.T.) ;
#8528=EDGE_CURVE('',#6724,#6721,#5113,.T.) ;
#8529=EDGE_CURVE('',#6723,#6722,#5114,.T.) ;
#8530=EDGE_CURVE('',#6725,#6662,#4005,.T.) ;
#8531=EDGE_CURVE('',#6725,#6726,#4006,.T.) ;
#8532=EDGE_CURVE('',#6659,#6726,#4007,.T.) ;
#8533=EDGE_CURVE('',#6657,#6727,#4008,.T.) ;
#8534=EDGE_CURVE('',#6728,#6727,#4009,.T.) ;
#8535=EDGE_CURVE('',#6728,#6660,#4010,.T.) ;
#8536=EDGE_CURVE('',#6728,#6725,#5115,.T.) ;
#8537=EDGE_CURVE('',#6727,#6726,#5116,.T.) ;
#8538=EDGE_CURVE('',#6729,#6658,#4011,.T.) ;
#8539=EDGE_CURVE('',#6729,#6730,#4012,.T.) ;
#8540=EDGE_CURVE('',#6655,#6730,#4013,.T.) ;
#8541=EDGE_CURVE('',#6653,#6731,#4014,.T.) ;
#8542=EDGE_CURVE('',#6732,#6731,#4015,.T.) ;
#8543=EDGE_CURVE('',#6732,#6656,#4016,.T.) ;
#8544=EDGE_CURVE('',#6732,#6729,#5117,.T.) ;
#8545=EDGE_CURVE('',#6731,#6730,#5118,.T.) ;
#8546=EDGE_CURVE('',#6733,#6647,#4017,.T.) ;
#8547=EDGE_CURVE('',#6733,#6734,#4018,.T.) ;
#8548=EDGE_CURVE('',#6651,#6734,#4019,.T.) ;
#8549=EDGE_CURVE('',#6649,#6735,#4020,.T.) ;
#8550=EDGE_CURVE('',#6736,#6735,#4021,.T.) ;
#8551=EDGE_CURVE('',#6736,#6646,#4022,.T.) ;
#8552=EDGE_CURVE('',#6736,#6733,#5119,.T.) ;
#8553=EDGE_CURVE('',#6735,#6734,#5120,.T.) ;
#8554=EDGE_CURVE('',#6737,#6654,#4023,.T.) ;
#8555=EDGE_CURVE('',#6737,#6738,#4024,.T.) ;
#8556=EDGE_CURVE('',#6645,#6738,#4025,.T.) ;
#8557=EDGE_CURVE('',#6644,#6739,#4026,.T.) ;
#8558=EDGE_CURVE('',#6740,#6739,#4027,.T.) ;
#8559=EDGE_CURVE('',#6740,#6652,#4028,.T.) ;
#8560=EDGE_CURVE('',#6740,#6737,#5121,.T.) ;
#8561=EDGE_CURVE('',#6739,#6738,#5122,.T.) ;
#8562=EDGE_CURVE('',#6741,#6650,#4029,.T.) ;
#8563=EDGE_CURVE('',#6741,#6742,#4030,.T.) ;
#8564=EDGE_CURVE('',#6643,#6742,#4031,.T.) ;
#8565=EDGE_CURVE('',#6641,#6743,#4032,.T.) ;
#8566=EDGE_CURVE('',#6744,#6743,#4033,.T.) ;
#8567=EDGE_CURVE('',#6744,#6648,#4034,.T.) ;
#8568=EDGE_CURVE('',#6744,#6741,#5123,.T.) ;
#8569=EDGE_CURVE('',#6743,#6742,#5124,.T.) ;
#8570=EDGE_CURVE('',#6745,#6642,#4035,.T.) ;
#8571=EDGE_CURVE('',#6745,#6746,#4036,.T.) ;
#8572=EDGE_CURVE('',#6639,#6746,#4037,.T.) ;
#8573=EDGE_CURVE('',#6637,#6747,#4038,.T.) ;
#8574=EDGE_CURVE('',#6748,#6747,#4039,.T.) ;
#8575=EDGE_CURVE('',#6748,#6640,#4040,.T.) ;
#8576=EDGE_CURVE('',#6748,#6745,#5125,.T.) ;
#8577=EDGE_CURVE('',#6747,#6746,#5126,.T.) ;
#8578=EDGE_CURVE('',#6749,#6638,#4041,.T.) ;
#8579=EDGE_CURVE('',#6749,#6750,#4042,.T.) ;
#8580=EDGE_CURVE('',#6635,#6750,#4043,.T.) ;
#8581=EDGE_CURVE('',#6633,#6751,#4044,.T.) ;
#8582=EDGE_CURVE('',#6752,#6751,#4045,.T.) ;
#8583=EDGE_CURVE('',#6752,#6636,#4046,.T.) ;
#8584=EDGE_CURVE('',#6752,#6749,#5127,.T.) ;
#8585=EDGE_CURVE('',#6751,#6750,#5128,.T.) ;
#8586=EDGE_CURVE('',#6753,#6634,#4047,.T.) ;
#8587=EDGE_CURVE('',#6753,#6754,#4048,.T.) ;
#8588=EDGE_CURVE('',#6631,#6754,#4049,.T.) ;
#8589=EDGE_CURVE('',#6629,#6755,#4050,.T.) ;
#8590=EDGE_CURVE('',#6756,#6755,#4051,.T.) ;
#8591=EDGE_CURVE('',#6756,#6632,#4052,.T.) ;
#8592=EDGE_CURVE('',#6756,#6753,#5129,.T.) ;
#8593=EDGE_CURVE('',#6755,#6754,#5130,.T.) ;
#8594=EDGE_CURVE('',#6757,#6630,#4053,.T.) ;
#8595=EDGE_CURVE('',#6757,#6758,#4054,.T.) ;
#8596=EDGE_CURVE('',#6627,#6758,#4055,.T.) ;
#8597=EDGE_CURVE('',#6625,#6759,#4056,.T.) ;
#8598=EDGE_CURVE('',#6760,#6759,#4057,.T.) ;
#8599=EDGE_CURVE('',#6760,#6628,#4058,.T.) ;
#8600=EDGE_CURVE('',#6760,#6757,#5131,.T.) ;
#8601=EDGE_CURVE('',#6759,#6758,#5132,.T.) ;
#8602=EDGE_CURVE('',#6761,#6626,#4059,.T.) ;
#8603=EDGE_CURVE('',#6761,#6762,#4060,.T.) ;
#8604=EDGE_CURVE('',#6623,#6762,#4061,.T.) ;
#8605=EDGE_CURVE('',#6621,#6763,#4062,.T.) ;
#8606=EDGE_CURVE('',#6764,#6763,#4063,.T.) ;
#8607=EDGE_CURVE('',#6764,#6624,#4064,.T.) ;
#8608=EDGE_CURVE('',#6764,#6761,#5133,.T.) ;
#8609=EDGE_CURVE('',#6763,#6762,#5134,.T.) ;
#8610=EDGE_CURVE('',#6765,#6622,#4065,.T.) ;
#8611=EDGE_CURVE('',#6765,#6766,#4066,.T.) ;
#8612=EDGE_CURVE('',#6619,#6766,#4067,.T.) ;
#8613=EDGE_CURVE('',#6617,#6767,#4068,.T.) ;
#8614=EDGE_CURVE('',#6768,#6767,#4069,.T.) ;
#8615=EDGE_CURVE('',#6768,#6620,#4070,.T.) ;
#8616=EDGE_CURVE('',#6768,#6765,#5135,.T.) ;
#8617=EDGE_CURVE('',#6767,#6766,#5136,.T.) ;
#8618=EDGE_CURVE('',#6769,#6618,#4071,.T.) ;
#8619=EDGE_CURVE('',#6769,#6770,#4072,.T.) ;
#8620=EDGE_CURVE('',#6615,#6770,#4073,.T.) ;
#8621=EDGE_CURVE('',#6613,#6771,#4074,.T.) ;
#8622=EDGE_CURVE('',#6772,#6771,#4075,.T.) ;
#8623=EDGE_CURVE('',#6772,#6616,#4076,.T.) ;
#8624=EDGE_CURVE('',#6772,#6769,#5137,.T.) ;
#8625=EDGE_CURVE('',#6771,#6770,#5138,.T.) ;
#8626=EDGE_CURVE('',#6773,#6614,#4077,.T.) ;
#8627=EDGE_CURVE('',#6773,#6774,#4078,.T.) ;
#8628=EDGE_CURVE('',#6611,#6774,#4079,.T.) ;
#8629=EDGE_CURVE('',#6609,#6775,#4080,.T.) ;
#8630=EDGE_CURVE('',#6776,#6775,#4081,.T.) ;
#8631=EDGE_CURVE('',#6776,#6612,#4082,.T.) ;
#8632=EDGE_CURVE('',#6776,#6773,#5139,.T.) ;
#8633=EDGE_CURVE('',#6775,#6774,#5140,.T.) ;
#8634=EDGE_CURVE('',#6777,#6610,#4083,.T.) ;
#8635=EDGE_CURVE('',#6777,#6778,#4084,.T.) ;
#8636=EDGE_CURVE('',#6607,#6778,#4085,.T.) ;
#8637=EDGE_CURVE('',#6605,#6779,#4086,.T.) ;
#8638=EDGE_CURVE('',#6780,#6779,#4087,.T.) ;
#8639=EDGE_CURVE('',#6780,#6608,#4088,.T.) ;
#8640=EDGE_CURVE('',#6780,#6777,#5141,.T.) ;
#8641=EDGE_CURVE('',#6779,#6778,#5142,.T.) ;
#8642=EDGE_CURVE('',#6781,#6599,#4089,.T.) ;
#8643=EDGE_CURVE('',#6781,#6782,#4090,.T.) ;
#8644=EDGE_CURVE('',#6603,#6782,#4091,.T.) ;
#8645=EDGE_CURVE('',#6601,#6783,#4092,.T.) ;
#8646=EDGE_CURVE('',#6784,#6783,#4093,.T.) ;
#8647=EDGE_CURVE('',#6784,#6598,#4094,.T.) ;
#8648=EDGE_CURVE('',#6784,#6781,#5143,.T.) ;
#8649=EDGE_CURVE('',#6783,#6782,#5144,.T.) ;
#8650=EDGE_CURVE('',#6785,#6595,#4095,.T.) ;
#8651=EDGE_CURVE('',#6785,#6786,#4096,.T.) ;
#8652=EDGE_CURVE('',#6597,#6786,#4097,.T.) ;
#8653=EDGE_CURVE('',#6596,#6787,#4098,.T.) ;
#8654=EDGE_CURVE('',#6788,#6787,#4099,.T.) ;
#8655=EDGE_CURVE('',#6788,#6594,#4100,.T.) ;
#8656=EDGE_CURVE('',#6788,#6785,#5145,.T.) ;
#8657=EDGE_CURVE('',#6787,#6786,#5146,.T.) ;
#8658=EDGE_CURVE('',#6789,#6591,#4101,.T.) ;
#8659=EDGE_CURVE('',#6789,#6790,#4102,.T.) ;
#8660=EDGE_CURVE('',#6593,#6790,#4103,.T.) ;
#8661=EDGE_CURVE('',#6592,#6791,#4104,.T.) ;
#8662=EDGE_CURVE('',#6792,#6791,#4105,.T.) ;
#8663=EDGE_CURVE('',#6792,#6590,#4106,.T.) ;
#8664=EDGE_CURVE('',#6792,#6789,#5147,.T.) ;
#8665=EDGE_CURVE('',#6791,#6790,#5148,.T.) ;
#8666=EDGE_CURVE('',#6793,#6587,#4107,.T.) ;
#8667=EDGE_CURVE('',#6793,#6794,#4108,.T.) ;
#8668=EDGE_CURVE('',#6589,#6794,#4109,.T.) ;
#8669=EDGE_CURVE('',#6588,#6795,#4110,.T.) ;
#8670=EDGE_CURVE('',#6796,#6795,#4111,.T.) ;
#8671=EDGE_CURVE('',#6796,#6586,#4112,.T.) ;
#8672=EDGE_CURVE('',#6796,#6793,#5149,.T.) ;
#8673=EDGE_CURVE('',#6795,#6794,#5150,.T.) ;
#8674=EDGE_CURVE('',#6797,#6583,#4113,.T.) ;
#8675=EDGE_CURVE('',#6797,#6798,#4114,.T.) ;
#8676=EDGE_CURVE('',#6585,#6798,#4115,.T.) ;
#8677=EDGE_CURVE('',#6584,#6799,#4116,.T.) ;
#8678=EDGE_CURVE('',#6800,#6799,#4117,.T.) ;
#8679=EDGE_CURVE('',#6800,#6582,#4118,.T.) ;
#8680=EDGE_CURVE('',#6800,#6797,#5151,.T.) ;
#8681=EDGE_CURVE('',#6799,#6798,#5152,.T.) ;
#8682=EDGE_CURVE('',#6801,#6579,#4119,.T.) ;
#8683=EDGE_CURVE('',#6801,#6802,#4120,.T.) ;
#8684=EDGE_CURVE('',#6581,#6802,#4121,.T.) ;
#8685=EDGE_CURVE('',#6580,#6803,#4122,.T.) ;
#8686=EDGE_CURVE('',#6804,#6803,#4123,.T.) ;
#8687=EDGE_CURVE('',#6804,#6578,#4124,.T.) ;
#8688=EDGE_CURVE('',#6804,#6801,#5153,.T.) ;
#8689=EDGE_CURVE('',#6803,#6802,#5154,.T.) ;
#8690=EDGE_CURVE('',#6805,#6575,#4125,.T.) ;
#8691=EDGE_CURVE('',#6805,#6806,#4126,.T.) ;
#8692=EDGE_CURVE('',#6577,#6806,#4127,.T.) ;
#8693=EDGE_CURVE('',#6576,#6807,#4128,.T.) ;
#8694=EDGE_CURVE('',#6808,#6807,#4129,.T.) ;
#8695=EDGE_CURVE('',#6808,#6574,#4130,.T.) ;
#8696=EDGE_CURVE('',#6808,#6805,#5155,.T.) ;
#8697=EDGE_CURVE('',#6807,#6806,#5156,.T.) ;
#8698=EDGE_CURVE('',#6809,#6606,#4131,.T.) ;
#8699=EDGE_CURVE('',#6809,#6810,#4132,.T.) ;
#8700=EDGE_CURVE('',#6573,#6810,#4133,.T.) ;
#8701=EDGE_CURVE('',#6572,#6811,#4134,.T.) ;
#8702=EDGE_CURVE('',#6812,#6811,#4135,.T.) ;
#8703=EDGE_CURVE('',#6812,#6604,#4136,.T.) ;
#8704=EDGE_CURVE('',#6812,#6809,#5157,.T.) ;
#8705=EDGE_CURVE('',#6811,#6810,#5158,.T.) ;
#8706=EDGE_CURVE('',#6813,#6602,#4137,.T.) ;
#8707=EDGE_CURVE('',#6813,#6814,#4138,.T.) ;
#8708=EDGE_CURVE('',#6571,#6814,#4139,.T.) ;
#8709=EDGE_CURVE('',#6569,#6815,#4140,.T.) ;
#8710=EDGE_CURVE('',#6816,#6815,#4141,.T.) ;
#8711=EDGE_CURVE('',#6816,#6600,#4142,.T.) ;
#8712=EDGE_CURVE('',#6816,#6813,#5159,.T.) ;
#8713=EDGE_CURVE('',#6815,#6814,#5160,.T.) ;
#8714=EDGE_CURVE('',#6817,#6570,#4143,.T.) ;
#8715=EDGE_CURVE('',#6817,#6818,#4144,.T.) ;
#8716=EDGE_CURVE('',#6567,#6818,#4145,.T.) ;
#8717=EDGE_CURVE('',#6565,#6819,#4146,.T.) ;
#8718=EDGE_CURVE('',#6820,#6819,#4147,.T.) ;
#8719=EDGE_CURVE('',#6820,#6568,#4148,.T.) ;
#8720=EDGE_CURVE('',#6820,#6817,#5161,.T.) ;
#8721=EDGE_CURVE('',#6819,#6818,#5162,.T.) ;
#8722=EDGE_CURVE('',#6821,#6566,#4149,.T.) ;
#8723=EDGE_CURVE('',#6821,#6822,#4150,.T.) ;
#8724=EDGE_CURVE('',#6563,#6822,#4151,.T.) ;
#8725=EDGE_CURVE('',#6561,#6823,#4152,.T.) ;
#8726=EDGE_CURVE('',#6824,#6823,#4153,.T.) ;
#8727=EDGE_CURVE('',#6824,#6564,#4154,.T.) ;
#8728=EDGE_CURVE('',#6824,#6821,#5163,.T.) ;
#8729=EDGE_CURVE('',#6823,#6822,#5164,.T.) ;
#8730=EDGE_CURVE('',#6825,#6562,#4155,.T.) ;
#8731=EDGE_CURVE('',#6825,#6826,#4156,.T.) ;
#8732=EDGE_CURVE('',#6559,#6826,#4157,.T.) ;
#8733=EDGE_CURVE('',#6557,#6827,#4158,.T.) ;
#8734=EDGE_CURVE('',#6828,#6827,#4159,.T.) ;
#8735=EDGE_CURVE('',#6828,#6560,#4160,.T.) ;
#8736=EDGE_CURVE('',#6828,#6825,#5165,.T.) ;
#8737=EDGE_CURVE('',#6827,#6826,#5166,.T.) ;
#8738=EDGE_CURVE('',#6829,#6558,#4161,.T.) ;
#8739=EDGE_CURVE('',#6829,#6830,#4162,.T.) ;
#8740=EDGE_CURVE('',#6555,#6830,#4163,.T.) ;
#8741=EDGE_CURVE('',#6553,#6831,#4164,.T.) ;
#8742=EDGE_CURVE('',#6832,#6831,#4165,.T.) ;
#8743=EDGE_CURVE('',#6832,#6556,#4166,.T.) ;
#8744=EDGE_CURVE('',#6832,#6829,#5167,.T.) ;
#8745=EDGE_CURVE('',#6831,#6830,#5168,.T.) ;
#8746=EDGE_CURVE('',#6833,#6554,#4167,.T.) ;
#8747=EDGE_CURVE('',#6833,#6834,#4168,.T.) ;
#8748=EDGE_CURVE('',#6551,#6834,#4169,.T.) ;
#8749=EDGE_CURVE('',#6549,#6835,#4170,.T.) ;
#8750=EDGE_CURVE('',#6836,#6835,#4171,.T.) ;
#8751=EDGE_CURVE('',#6836,#6552,#4172,.T.) ;
#8752=EDGE_CURVE('',#6836,#6833,#5169,.T.) ;
#8753=EDGE_CURVE('',#6835,#6834,#5170,.T.) ;
#8754=EDGE_CURVE('',#6837,#6550,#4173,.T.) ;
#8755=EDGE_CURVE('',#6837,#6838,#4174,.T.) ;
#8756=EDGE_CURVE('',#6547,#6838,#4175,.T.) ;
#8757=EDGE_CURVE('',#6545,#6839,#4176,.T.) ;
#8758=EDGE_CURVE('',#6840,#6839,#4177,.T.) ;
#8759=EDGE_CURVE('',#6840,#6548,#4178,.T.) ;
#8760=EDGE_CURVE('',#6840,#6837,#5171,.T.) ;
#8761=EDGE_CURVE('',#6839,#6838,#5172,.T.) ;
#8762=EDGE_CURVE('',#6841,#6546,#4179,.T.) ;
#8763=EDGE_CURVE('',#6841,#6842,#4180,.T.) ;
#8764=EDGE_CURVE('',#6543,#6842,#4181,.T.) ;
#8765=EDGE_CURVE('',#6541,#6843,#4182,.T.) ;
#8766=EDGE_CURVE('',#6844,#6843,#4183,.T.) ;
#8767=EDGE_CURVE('',#6844,#6544,#4184,.T.) ;
#8768=EDGE_CURVE('',#6844,#6841,#5173,.T.) ;
#8769=EDGE_CURVE('',#6843,#6842,#5174,.T.) ;
#8770=EDGE_CURVE('',#6845,#6542,#4185,.T.) ;
#8771=EDGE_CURVE('',#6845,#6846,#4186,.T.) ;
#8772=EDGE_CURVE('',#6539,#6846,#4187,.T.) ;
#8773=EDGE_CURVE('',#6537,#6847,#4188,.T.) ;
#8774=EDGE_CURVE('',#6848,#6847,#4189,.T.) ;
#8775=EDGE_CURVE('',#6848,#6540,#4190,.T.) ;
#8776=EDGE_CURVE('',#6848,#6845,#5175,.T.) ;
#8777=EDGE_CURVE('',#6847,#6846,#5176,.T.) ;
#8778=EDGE_CURVE('',#6849,#6538,#4191,.T.) ;
#8779=EDGE_CURVE('',#6849,#6850,#4192,.T.) ;
#8780=EDGE_CURVE('',#6535,#6850,#4193,.T.) ;
#8781=EDGE_CURVE('',#6533,#6851,#4194,.T.) ;
#8782=EDGE_CURVE('',#6852,#6851,#4195,.T.) ;
#8783=EDGE_CURVE('',#6852,#6536,#4196,.T.) ;
#8784=EDGE_CURVE('',#6852,#6849,#5177,.T.) ;
#8785=EDGE_CURVE('',#6851,#6850,#5178,.T.) ;
#8786=EDGE_CURVE('',#6853,#6527,#4197,.T.) ;
#8787=EDGE_CURVE('',#6853,#6854,#4198,.T.) ;
#8788=EDGE_CURVE('',#6531,#6854,#4199,.T.) ;
#8789=EDGE_CURVE('',#6529,#6855,#4200,.T.) ;
#8790=EDGE_CURVE('',#6856,#6855,#4201,.T.) ;
#8791=EDGE_CURVE('',#6856,#6526,#4202,.T.) ;
#8792=EDGE_CURVE('',#6856,#6853,#5179,.T.) ;
#8793=EDGE_CURVE('',#6855,#6854,#5180,.T.) ;
#8794=EDGE_CURVE('',#6857,#6534,#4203,.T.) ;
#8795=EDGE_CURVE('',#6857,#6858,#4204,.T.) ;
#8796=EDGE_CURVE('',#6525,#6858,#4205,.T.) ;
#8797=EDGE_CURVE('',#6524,#6859,#4206,.T.) ;
#8798=EDGE_CURVE('',#6860,#6859,#4207,.T.) ;
#8799=EDGE_CURVE('',#6860,#6532,#4208,.T.) ;
#8800=EDGE_CURVE('',#6860,#6857,#5181,.T.) ;
#8801=EDGE_CURVE('',#6859,#6858,#5182,.T.) ;
#8802=EDGE_CURVE('',#6861,#6530,#4209,.T.) ;
#8803=EDGE_CURVE('',#6861,#6862,#4210,.T.) ;
#8804=EDGE_CURVE('',#6523,#6862,#4211,.T.) ;
#8805=EDGE_CURVE('',#6521,#6863,#4212,.T.) ;
#8806=EDGE_CURVE('',#6864,#6863,#4213,.T.) ;
#8807=EDGE_CURVE('',#6864,#6528,#4214,.T.) ;
#8808=EDGE_CURVE('',#6864,#6861,#5183,.T.) ;
#8809=EDGE_CURVE('',#6863,#6862,#5184,.T.) ;
#8810=EDGE_CURVE('',#6865,#6522,#4215,.T.) ;
#8811=EDGE_CURVE('',#6865,#6866,#4216,.T.) ;
#8812=EDGE_CURVE('',#6519,#6866,#4217,.T.) ;
#8813=EDGE_CURVE('',#6517,#6867,#4218,.T.) ;
#8814=EDGE_CURVE('',#6868,#6867,#4219,.T.) ;
#8815=EDGE_CURVE('',#6868,#6520,#4220,.T.) ;
#8816=EDGE_CURVE('',#6868,#6865,#5185,.T.) ;
#8817=EDGE_CURVE('',#6867,#6866,#5186,.T.) ;
#8818=EDGE_CURVE('',#6869,#6518,#4221,.T.) ;
#8819=EDGE_CURVE('',#6869,#6870,#4222,.T.) ;
#8820=EDGE_CURVE('',#6515,#6870,#4223,.T.) ;
#8821=EDGE_CURVE('',#6513,#6871,#4224,.T.) ;
#8822=EDGE_CURVE('',#6872,#6871,#4225,.T.) ;
#8823=EDGE_CURVE('',#6872,#6516,#4226,.T.) ;
#8824=EDGE_CURVE('',#6872,#6869,#5187,.T.) ;
#8825=EDGE_CURVE('',#6871,#6870,#5188,.T.) ;
#8826=EDGE_CURVE('',#6873,#6514,#4227,.T.) ;
#8827=EDGE_CURVE('',#6873,#6874,#4228,.T.) ;
#8828=EDGE_CURVE('',#6511,#6874,#4229,.T.) ;
#8829=EDGE_CURVE('',#6509,#6875,#4230,.T.) ;
#8830=EDGE_CURVE('',#6876,#6875,#4231,.T.) ;
#8831=EDGE_CURVE('',#6876,#6512,#4232,.T.) ;
#8832=EDGE_CURVE('',#6876,#6873,#5189,.T.) ;
#8833=EDGE_CURVE('',#6875,#6874,#5190,.T.) ;
#8834=EDGE_CURVE('',#6877,#6510,#4233,.T.) ;
#8835=EDGE_CURVE('',#6877,#6878,#4234,.T.) ;
#8836=EDGE_CURVE('',#6507,#6878,#4235,.T.) ;
#8837=EDGE_CURVE('',#6505,#6879,#4236,.T.) ;
#8838=EDGE_CURVE('',#6880,#6879,#4237,.T.) ;
#8839=EDGE_CURVE('',#6880,#6508,#4238,.T.) ;
#8840=EDGE_CURVE('',#6880,#6877,#5191,.T.) ;
#8841=EDGE_CURVE('',#6879,#6878,#5192,.T.) ;
#8842=EDGE_CURVE('',#6881,#6506,#4239,.T.) ;
#8843=EDGE_CURVE('',#6881,#6882,#4240,.T.) ;
#8844=EDGE_CURVE('',#6503,#6882,#4241,.T.) ;
#8845=EDGE_CURVE('',#6501,#6883,#4242,.T.) ;
#8846=EDGE_CURVE('',#6884,#6883,#4243,.T.) ;
#8847=EDGE_CURVE('',#6884,#6504,#4244,.T.) ;
#8848=EDGE_CURVE('',#6884,#6881,#5193,.T.) ;
#8849=EDGE_CURVE('',#6883,#6882,#5194,.T.) ;
#8850=EDGE_CURVE('',#6885,#6502,#4245,.T.) ;
#8851=EDGE_CURVE('',#6885,#6886,#4246,.T.) ;
#8852=EDGE_CURVE('',#6499,#6886,#4247,.T.) ;
#8853=EDGE_CURVE('',#6497,#6887,#4248,.T.) ;
#8854=EDGE_CURVE('',#6888,#6887,#4249,.T.) ;
#8855=EDGE_CURVE('',#6888,#6500,#4250,.T.) ;
#8856=EDGE_CURVE('',#6888,#6885,#5195,.T.) ;
#8857=EDGE_CURVE('',#6887,#6886,#5196,.T.) ;
#8858=EDGE_CURVE('',#6889,#6498,#4251,.T.) ;
#8859=EDGE_CURVE('',#6889,#6890,#4252,.T.) ;
#8860=EDGE_CURVE('',#6495,#6890,#4253,.T.) ;
#8861=EDGE_CURVE('',#6493,#6891,#4254,.T.) ;
#8862=EDGE_CURVE('',#6892,#6891,#4255,.T.) ;
#8863=EDGE_CURVE('',#6892,#6496,#4256,.T.) ;
#8864=EDGE_CURVE('',#6892,#6889,#5197,.T.) ;
#8865=EDGE_CURVE('',#6891,#6890,#5198,.T.) ;
#8866=EDGE_CURVE('',#6893,#6494,#4257,.T.) ;
#8867=EDGE_CURVE('',#6893,#6894,#4258,.T.) ;
#8868=EDGE_CURVE('',#6491,#6894,#4259,.T.) ;
#8869=EDGE_CURVE('',#6489,#6895,#4260,.T.) ;
#8870=EDGE_CURVE('',#6896,#6895,#4261,.T.) ;
#8871=EDGE_CURVE('',#6896,#6492,#4262,.T.) ;
#8872=EDGE_CURVE('',#6896,#6893,#5199,.T.) ;
#8873=EDGE_CURVE('',#6895,#6894,#5200,.T.) ;
#8874=EDGE_CURVE('',#6897,#6490,#4263,.T.) ;
#8875=EDGE_CURVE('',#6897,#6898,#4264,.T.) ;
#8876=EDGE_CURVE('',#6487,#6898,#4265,.T.) ;
#8877=EDGE_CURVE('',#6485,#6899,#4266,.T.) ;
#8878=EDGE_CURVE('',#6900,#6899,#4267,.T.) ;
#8879=EDGE_CURVE('',#6900,#6488,#4268,.T.) ;
#8880=EDGE_CURVE('',#6900,#6897,#5201,.T.) ;
#8881=EDGE_CURVE('',#6899,#6898,#5202,.T.) ;
#8882=EDGE_CURVE('',#6901,#6486,#4269,.T.) ;
#8883=EDGE_CURVE('',#6901,#6902,#4270,.T.) ;
#8884=EDGE_CURVE('',#6483,#6902,#4271,.T.) ;
#8885=EDGE_CURVE('',#6481,#6903,#4272,.T.) ;
#8886=EDGE_CURVE('',#6904,#6903,#4273,.T.) ;
#8887=EDGE_CURVE('',#6904,#6484,#4274,.T.) ;
#8888=EDGE_CURVE('',#6904,#6901,#5203,.T.) ;
#8889=EDGE_CURVE('',#6903,#6902,#5204,.T.) ;
#8890=EDGE_CURVE('',#6905,#6482,#4275,.T.) ;
#8891=EDGE_CURVE('',#6905,#6906,#4276,.T.) ;
#8892=EDGE_CURVE('',#6479,#6906,#4277,.T.) ;
#8893=EDGE_CURVE('',#6477,#6907,#4278,.T.) ;
#8894=EDGE_CURVE('',#6908,#6907,#4279,.T.) ;
#8895=EDGE_CURVE('',#6908,#6480,#4280,.T.) ;
#8896=EDGE_CURVE('',#6908,#6905,#5205,.T.) ;
#8897=EDGE_CURVE('',#6907,#6906,#5206,.T.) ;
#8898=EDGE_CURVE('',#6909,#6471,#4281,.T.) ;
#8899=EDGE_CURVE('',#6909,#6910,#4282,.T.) ;
#8900=EDGE_CURVE('',#6475,#6910,#4283,.T.) ;
#8901=EDGE_CURVE('',#6473,#6911,#4284,.T.) ;
#8902=EDGE_CURVE('',#6912,#6911,#4285,.T.) ;
#8903=EDGE_CURVE('',#6912,#6470,#4286,.T.) ;
#8904=EDGE_CURVE('',#6912,#6909,#5207,.T.) ;
#8905=EDGE_CURVE('',#6911,#6910,#5208,.T.) ;
#8906=EDGE_CURVE('',#6913,#6467,#4287,.T.) ;
#8907=EDGE_CURVE('',#6913,#6914,#4288,.T.) ;
#8908=EDGE_CURVE('',#6469,#6914,#4289,.T.) ;
#8909=EDGE_CURVE('',#6468,#6915,#4290,.T.) ;
#8910=EDGE_CURVE('',#6916,#6915,#4291,.T.) ;
#8911=EDGE_CURVE('',#6916,#6466,#4292,.T.) ;
#8912=EDGE_CURVE('',#6916,#6913,#5209,.T.) ;
#8913=EDGE_CURVE('',#6915,#6914,#5210,.T.) ;
#8914=EDGE_CURVE('',#6917,#6463,#4293,.T.) ;
#8915=EDGE_CURVE('',#6917,#6918,#4294,.T.) ;
#8916=EDGE_CURVE('',#6465,#6918,#4295,.T.) ;
#8917=EDGE_CURVE('',#6464,#6919,#4296,.T.) ;
#8918=EDGE_CURVE('',#6920,#6919,#4297,.T.) ;
#8919=EDGE_CURVE('',#6920,#6462,#4298,.T.) ;
#8920=EDGE_CURVE('',#6920,#6917,#5211,.T.) ;
#8921=EDGE_CURVE('',#6919,#6918,#5212,.T.) ;
#8922=EDGE_CURVE('',#6921,#6478,#4299,.T.) ;
#8923=EDGE_CURVE('',#6921,#6922,#4300,.T.) ;
#8924=EDGE_CURVE('',#6461,#6922,#4301,.T.) ;
#8925=EDGE_CURVE('',#6460,#6923,#4302,.T.) ;
#8926=EDGE_CURVE('',#6924,#6923,#4303,.T.) ;
#8927=EDGE_CURVE('',#6924,#6476,#4304,.T.) ;
#8928=EDGE_CURVE('',#6924,#6921,#5213,.T.) ;
#8929=EDGE_CURVE('',#6923,#6922,#5214,.T.) ;
#8930=EDGE_CURVE('',#6925,#6474,#4305,.T.) ;
#8931=EDGE_CURVE('',#6925,#6926,#4306,.T.) ;
#8932=EDGE_CURVE('',#6459,#6926,#4307,.T.) ;
#8933=EDGE_CURVE('',#6457,#6927,#4308,.T.) ;
#8934=EDGE_CURVE('',#6928,#6927,#4309,.T.) ;
#8935=EDGE_CURVE('',#6928,#6472,#4310,.T.) ;
#8936=EDGE_CURVE('',#6928,#6925,#5215,.T.) ;
#8937=EDGE_CURVE('',#6927,#6926,#5216,.T.) ;
#8938=EDGE_CURVE('',#6929,#6458,#4311,.T.) ;
#8939=EDGE_CURVE('',#6929,#6930,#4312,.T.) ;
#8940=EDGE_CURVE('',#6455,#6930,#4313,.T.) ;
#8941=EDGE_CURVE('',#6453,#6931,#4314,.T.) ;
#8942=EDGE_CURVE('',#6932,#6931,#4315,.T.) ;
#8943=EDGE_CURVE('',#6932,#6456,#4316,.T.) ;
#8944=EDGE_CURVE('',#6932,#6929,#5217,.T.) ;
#8945=EDGE_CURVE('',#6931,#6930,#5218,.T.) ;
#8946=EDGE_CURVE('',#6933,#6454,#4317,.T.) ;
#8947=EDGE_CURVE('',#6933,#6934,#4318,.T.) ;
#8948=EDGE_CURVE('',#6451,#6934,#4319,.T.) ;
#8949=EDGE_CURVE('',#6449,#6935,#4320,.T.) ;
#8950=EDGE_CURVE('',#6936,#6935,#4321,.T.) ;
#8951=EDGE_CURVE('',#6936,#6452,#4322,.T.) ;
#8952=EDGE_CURVE('',#6936,#6933,#5219,.T.) ;
#8953=EDGE_CURVE('',#6935,#6934,#5220,.T.) ;
#8954=EDGE_CURVE('',#6937,#6450,#4323,.T.) ;
#8955=EDGE_CURVE('',#6937,#6938,#4324,.T.) ;
#8956=EDGE_CURVE('',#6445,#6938,#4325,.T.) ;
#8957=EDGE_CURVE('',#6444,#6939,#4326,.T.) ;
#8958=EDGE_CURVE('',#6940,#6939,#4327,.T.) ;
#8959=EDGE_CURVE('',#6940,#6448,#4328,.T.) ;
#8960=EDGE_CURVE('',#6940,#6937,#5221,.T.) ;
#8961=EDGE_CURVE('',#6939,#6938,#5222,.T.) ;
#11058=ORIENTED_EDGE('',*,*,#8083,.F.) ;
#11059=ORIENTED_EDGE('',*,*,#8084,.F.) ;
#11060=ORIENTED_EDGE('',*,*,#8085,.T.) ;
#11061=ORIENTED_EDGE('',*,*,#8086,.F.) ;
#11062=ORIENTED_EDGE('',*,*,#8087,.F.) ;
#11063=ORIENTED_EDGE('',*,*,#8088,.T.) ;
#11064=ORIENTED_EDGE('',*,*,#8089,.F.) ;
#11065=ORIENTED_EDGE('',*,*,#8085,.F.) ;
#11066=ORIENTED_EDGE('',*,*,#8090,.F.) ;
#11067=ORIENTED_EDGE('',*,*,#8091,.F.) ;
#11068=ORIENTED_EDGE('',*,*,#8088,.F.) ;
#11069=ORIENTED_EDGE('',*,*,#8092,.F.) ;
#11070=ORIENTED_EDGE('',*,*,#8093,.F.) ;
#11071=ORIENTED_EDGE('',*,*,#8092,.T.) ;
#11072=ORIENTED_EDGE('',*,*,#8087,.T.) ;
#11073=ORIENTED_EDGE('',*,*,#8084,.T.) ;
#11074=ORIENTED_EDGE('',*,*,#8094,.T.) ;
#11075=ORIENTED_EDGE('',*,*,#8095,.F.) ;
#11076=ORIENTED_EDGE('',*,*,#8096,.F.) ;
#11077=ORIENTED_EDGE('',*,*,#8097,.T.) ;
#11078=ORIENTED_EDGE('',*,*,#8098,.T.) ;
#11079=ORIENTED_EDGE('',*,*,#8099,.F.) ;
#11080=ORIENTED_EDGE('',*,*,#8100,.T.) ;
#11081=ORIENTED_EDGE('',*,*,#8101,.T.) ;
#11082=ORIENTED_EDGE('',*,*,#8102,.F.) ;
#11083=ORIENTED_EDGE('',*,*,#8103,.F.) ;
#11084=ORIENTED_EDGE('',*,*,#8104,.T.) ;
#11085=ORIENTED_EDGE('',*,*,#8105,.T.) ;
#11086=ORIENTED_EDGE('',*,*,#8106,.F.) ;
#11087=ORIENTED_EDGE('',*,*,#8107,.F.) ;
#11088=ORIENTED_EDGE('',*,*,#8108,.T.) ;
#11089=ORIENTED_EDGE('',*,*,#8109,.T.) ;
#11090=ORIENTED_EDGE('',*,*,#8110,.F.) ;
#11091=ORIENTED_EDGE('',*,*,#8111,.F.) ;
#11092=ORIENTED_EDGE('',*,*,#8112,.F.) ;
#11093=ORIENTED_EDGE('',*,*,#8113,.T.) ;
#11094=ORIENTED_EDGE('',*,*,#8114,.T.) ;
#11095=ORIENTED_EDGE('',*,*,#8115,.F.) ;
#11096=ORIENTED_EDGE('',*,*,#8116,.F.) ;
#11097=ORIENTED_EDGE('',*,*,#8117,.T.) ;
#11098=ORIENTED_EDGE('',*,*,#8118,.T.) ;
#11099=ORIENTED_EDGE('',*,*,#8119,.F.) ;
#11100=ORIENTED_EDGE('',*,*,#8120,.F.) ;
#11101=ORIENTED_EDGE('',*,*,#8121,.T.) ;
#11102=ORIENTED_EDGE('',*,*,#8122,.T.) ;
#11103=ORIENTED_EDGE('',*,*,#8123,.F.) ;
#11104=ORIENTED_EDGE('',*,*,#8124,.T.) ;
#11105=ORIENTED_EDGE('',*,*,#8125,.T.) ;
#11106=ORIENTED_EDGE('',*,*,#8126,.F.) ;
#11107=ORIENTED_EDGE('',*,*,#8127,.F.) ;
#11108=ORIENTED_EDGE('',*,*,#8128,.T.) ;
#11109=ORIENTED_EDGE('',*,*,#8129,.T.) ;
#11110=ORIENTED_EDGE('',*,*,#8130,.F.) ;
#11111=ORIENTED_EDGE('',*,*,#8131,.F.) ;
#11112=ORIENTED_EDGE('',*,*,#8132,.T.) ;
#11113=ORIENTED_EDGE('',*,*,#8133,.T.) ;
#11114=ORIENTED_EDGE('',*,*,#8134,.F.) ;
#11115=ORIENTED_EDGE('',*,*,#8135,.F.) ;
#11116=ORIENTED_EDGE('',*,*,#8136,.T.) ;
#11117=ORIENTED_EDGE('',*,*,#8137,.T.) ;
#11118=ORIENTED_EDGE('',*,*,#8138,.F.) ;
#11119=ORIENTED_EDGE('',*,*,#8139,.F.) ;
#11120=ORIENTED_EDGE('',*,*,#8140,.T.) ;
#11121=ORIENTED_EDGE('',*,*,#8141,.T.) ;
#11122=ORIENTED_EDGE('',*,*,#8142,.F.) ;
#11123=ORIENTED_EDGE('',*,*,#8143,.F.) ;
#11124=ORIENTED_EDGE('',*,*,#8144,.T.) ;
#11125=ORIENTED_EDGE('',*,*,#8145,.T.) ;
#11126=ORIENTED_EDGE('',*,*,#8146,.F.) ;
#11127=ORIENTED_EDGE('',*,*,#8147,.F.) ;
#11128=ORIENTED_EDGE('',*,*,#8148,.T.) ;
#11129=ORIENTED_EDGE('',*,*,#8149,.T.) ;
#11130=ORIENTED_EDGE('',*,*,#8150,.F.) ;
#11131=ORIENTED_EDGE('',*,*,#8151,.F.) ;
#11132=ORIENTED_EDGE('',*,*,#8152,.T.) ;
#11133=ORIENTED_EDGE('',*,*,#8153,.T.) ;
#11134=ORIENTED_EDGE('',*,*,#8154,.F.) ;
#11135=ORIENTED_EDGE('',*,*,#8155,.F.) ;
#11136=ORIENTED_EDGE('',*,*,#8156,.T.) ;
#11137=ORIENTED_EDGE('',*,*,#8157,.T.) ;
#11138=ORIENTED_EDGE('',*,*,#8158,.F.) ;
#11139=ORIENTED_EDGE('',*,*,#8159,.F.) ;
#11140=ORIENTED_EDGE('',*,*,#8160,.T.) ;
#11141=ORIENTED_EDGE('',*,*,#8161,.T.) ;
#11142=ORIENTED_EDGE('',*,*,#8162,.F.) ;
#11143=ORIENTED_EDGE('',*,*,#8163,.F.) ;
#11144=ORIENTED_EDGE('',*,*,#8164,.T.) ;
#11145=ORIENTED_EDGE('',*,*,#8165,.T.) ;
#11146=ORIENTED_EDGE('',*,*,#8166,.F.) ;
#11147=ORIENTED_EDGE('',*,*,#8167,.F.) ;
#11148=ORIENTED_EDGE('',*,*,#8168,.T.) ;
#11149=ORIENTED_EDGE('',*,*,#8169,.T.) ;
#11150=ORIENTED_EDGE('',*,*,#8170,.F.) ;
#11151=ORIENTED_EDGE('',*,*,#8171,.F.) ;
#11152=ORIENTED_EDGE('',*,*,#8172,.T.) ;
#11153=ORIENTED_EDGE('',*,*,#8173,.T.) ;
#11154=ORIENTED_EDGE('',*,*,#8174,.F.) ;
#11155=ORIENTED_EDGE('',*,*,#8175,.F.) ;
#11156=ORIENTED_EDGE('',*,*,#8176,.F.) ;
#11157=ORIENTED_EDGE('',*,*,#8177,.T.) ;
#11158=ORIENTED_EDGE('',*,*,#8178,.T.) ;
#11159=ORIENTED_EDGE('',*,*,#8179,.F.) ;
#11160=ORIENTED_EDGE('',*,*,#8180,.T.) ;
#11161=ORIENTED_EDGE('',*,*,#8181,.T.) ;
#11162=ORIENTED_EDGE('',*,*,#8182,.F.) ;
#11163=ORIENTED_EDGE('',*,*,#8183,.F.) ;
#11164=ORIENTED_EDGE('',*,*,#8184,.T.) ;
#11165=ORIENTED_EDGE('',*,*,#8185,.T.) ;
#11166=ORIENTED_EDGE('',*,*,#8186,.F.) ;
#11167=ORIENTED_EDGE('',*,*,#8187,.F.) ;
#11168=ORIENTED_EDGE('',*,*,#8188,.T.) ;
#11169=ORIENTED_EDGE('',*,*,#8189,.T.) ;
#11170=ORIENTED_EDGE('',*,*,#8190,.F.) ;
#11171=ORIENTED_EDGE('',*,*,#8191,.F.) ;
#11172=ORIENTED_EDGE('',*,*,#8192,.T.) ;
#11173=ORIENTED_EDGE('',*,*,#8193,.T.) ;
#11174=ORIENTED_EDGE('',*,*,#8194,.F.) ;
#11175=ORIENTED_EDGE('',*,*,#8195,.F.) ;
#11176=ORIENTED_EDGE('',*,*,#8196,.T.) ;
#11177=ORIENTED_EDGE('',*,*,#8197,.T.) ;
#11178=ORIENTED_EDGE('',*,*,#8198,.F.) ;
#11179=ORIENTED_EDGE('',*,*,#8199,.F.) ;
#11180=ORIENTED_EDGE('',*,*,#8200,.T.) ;
#11181=ORIENTED_EDGE('',*,*,#8201,.T.) ;
#11182=ORIENTED_EDGE('',*,*,#8202,.F.) ;
#11183=ORIENTED_EDGE('',*,*,#8203,.F.) ;
#11184=ORIENTED_EDGE('',*,*,#8204,.T.) ;
#11185=ORIENTED_EDGE('',*,*,#8205,.T.) ;
#11186=ORIENTED_EDGE('',*,*,#8206,.F.) ;
#11187=ORIENTED_EDGE('',*,*,#8207,.F.) ;
#11188=ORIENTED_EDGE('',*,*,#8208,.T.) ;
#11189=ORIENTED_EDGE('',*,*,#8209,.T.) ;
#11190=ORIENTED_EDGE('',*,*,#8210,.F.) ;
#11191=ORIENTED_EDGE('',*,*,#8211,.F.) ;
#11192=ORIENTED_EDGE('',*,*,#8212,.T.) ;
#11193=ORIENTED_EDGE('',*,*,#8213,.T.) ;
#11194=ORIENTED_EDGE('',*,*,#8214,.F.) ;
#11195=ORIENTED_EDGE('',*,*,#8215,.F.) ;
#11196=ORIENTED_EDGE('',*,*,#8216,.T.) ;
#11197=ORIENTED_EDGE('',*,*,#8217,.T.) ;
#11198=ORIENTED_EDGE('',*,*,#8218,.F.) ;
#11199=ORIENTED_EDGE('',*,*,#8219,.F.) ;
#11200=ORIENTED_EDGE('',*,*,#8220,.T.) ;
#11201=ORIENTED_EDGE('',*,*,#8221,.T.) ;
#11202=ORIENTED_EDGE('',*,*,#8222,.F.) ;
#11203=ORIENTED_EDGE('',*,*,#8223,.F.) ;
#11204=ORIENTED_EDGE('',*,*,#8224,.F.) ;
#11205=ORIENTED_EDGE('',*,*,#8225,.T.) ;
#11206=ORIENTED_EDGE('',*,*,#8226,.T.) ;
#11207=ORIENTED_EDGE('',*,*,#8227,.F.) ;
#11208=ORIENTED_EDGE('',*,*,#8228,.F.) ;
#11209=ORIENTED_EDGE('',*,*,#8229,.T.) ;
#11210=ORIENTED_EDGE('',*,*,#8230,.T.) ;
#11211=ORIENTED_EDGE('',*,*,#8231,.F.) ;
#11212=ORIENTED_EDGE('',*,*,#8232,.F.) ;
#11213=ORIENTED_EDGE('',*,*,#8233,.T.) ;
#11214=ORIENTED_EDGE('',*,*,#8234,.T.) ;
#11215=ORIENTED_EDGE('',*,*,#8235,.F.) ;
#11216=ORIENTED_EDGE('',*,*,#8236,.F.) ;
#11217=ORIENTED_EDGE('',*,*,#8237,.T.) ;
#11218=ORIENTED_EDGE('',*,*,#8238,.T.) ;
#11219=ORIENTED_EDGE('',*,*,#8239,.F.) ;
#11220=ORIENTED_EDGE('',*,*,#8240,.F.) ;
#11221=ORIENTED_EDGE('',*,*,#8241,.T.) ;
#11222=ORIENTED_EDGE('',*,*,#8242,.T.) ;
#11223=ORIENTED_EDGE('',*,*,#8243,.F.) ;
#11224=ORIENTED_EDGE('',*,*,#8244,.F.) ;
#11225=ORIENTED_EDGE('',*,*,#8245,.T.) ;
#11226=ORIENTED_EDGE('',*,*,#8246,.T.) ;
#11227=ORIENTED_EDGE('',*,*,#8247,.F.) ;
#11228=ORIENTED_EDGE('',*,*,#8248,.F.) ;
#11229=ORIENTED_EDGE('',*,*,#8249,.T.) ;
#11230=ORIENTED_EDGE('',*,*,#8250,.T.) ;
#11231=ORIENTED_EDGE('',*,*,#8251,.F.) ;
#11232=ORIENTED_EDGE('',*,*,#8252,.T.) ;
#11233=ORIENTED_EDGE('',*,*,#8253,.T.) ;
#11234=ORIENTED_EDGE('',*,*,#8254,.F.) ;
#11235=ORIENTED_EDGE('',*,*,#8255,.F.) ;
#11236=ORIENTED_EDGE('',*,*,#8256,.T.) ;
#11237=ORIENTED_EDGE('',*,*,#8257,.T.) ;
#11238=ORIENTED_EDGE('',*,*,#8258,.F.) ;
#11239=ORIENTED_EDGE('',*,*,#8259,.F.) ;
#11240=ORIENTED_EDGE('',*,*,#8260,.T.) ;
#11241=ORIENTED_EDGE('',*,*,#8261,.T.) ;
#11242=ORIENTED_EDGE('',*,*,#8262,.F.) ;
#11243=ORIENTED_EDGE('',*,*,#8263,.F.) ;
#11244=ORIENTED_EDGE('',*,*,#8264,.T.) ;
#11245=ORIENTED_EDGE('',*,*,#8265,.T.) ;
#11246=ORIENTED_EDGE('',*,*,#8266,.F.) ;
#11247=ORIENTED_EDGE('',*,*,#8267,.F.) ;
#11248=ORIENTED_EDGE('',*,*,#8268,.T.) ;
#11249=ORIENTED_EDGE('',*,*,#8269,.T.) ;
#11250=ORIENTED_EDGE('',*,*,#8270,.F.) ;
#11251=ORIENTED_EDGE('',*,*,#8271,.F.) ;
#11252=ORIENTED_EDGE('',*,*,#8272,.T.) ;
#11253=ORIENTED_EDGE('',*,*,#8273,.T.) ;
#11254=ORIENTED_EDGE('',*,*,#8274,.F.) ;
#11255=ORIENTED_EDGE('',*,*,#8275,.F.) ;
#11256=ORIENTED_EDGE('',*,*,#8276,.T.) ;
#11257=ORIENTED_EDGE('',*,*,#8277,.T.) ;
#11258=ORIENTED_EDGE('',*,*,#8278,.F.) ;
#11259=ORIENTED_EDGE('',*,*,#8279,.F.) ;
#11260=ORIENTED_EDGE('',*,*,#8280,.T.) ;
#11261=ORIENTED_EDGE('',*,*,#8281,.T.) ;
#11262=ORIENTED_EDGE('',*,*,#8282,.F.) ;
#11263=ORIENTED_EDGE('',*,*,#8283,.F.) ;
#11264=ORIENTED_EDGE('',*,*,#8284,.T.) ;
#11265=ORIENTED_EDGE('',*,*,#8285,.T.) ;
#11266=ORIENTED_EDGE('',*,*,#8286,.F.) ;
#11267=ORIENTED_EDGE('',*,*,#8287,.F.) ;
#11268=ORIENTED_EDGE('',*,*,#8288,.T.) ;
#11269=ORIENTED_EDGE('',*,*,#8289,.T.) ;
#11270=ORIENTED_EDGE('',*,*,#8290,.F.) ;
#11271=ORIENTED_EDGE('',*,*,#8291,.F.) ;
#11272=ORIENTED_EDGE('',*,*,#8292,.T.) ;
#11273=ORIENTED_EDGE('',*,*,#8293,.T.) ;
#11274=ORIENTED_EDGE('',*,*,#8294,.F.) ;
#11275=ORIENTED_EDGE('',*,*,#8295,.F.) ;
#11276=ORIENTED_EDGE('',*,*,#8296,.F.) ;
#11277=ORIENTED_EDGE('',*,*,#8297,.T.) ;
#11278=ORIENTED_EDGE('',*,*,#8298,.T.) ;
#11279=ORIENTED_EDGE('',*,*,#8299,.F.) ;
#11280=ORIENTED_EDGE('',*,*,#8300,.T.) ;
#11281=ORIENTED_EDGE('',*,*,#8301,.T.) ;
#11282=ORIENTED_EDGE('',*,*,#8302,.F.) ;
#11283=ORIENTED_EDGE('',*,*,#8303,.F.) ;
#11284=ORIENTED_EDGE('',*,*,#8304,.T.) ;
#11285=ORIENTED_EDGE('',*,*,#8305,.T.) ;
#11286=ORIENTED_EDGE('',*,*,#8306,.F.) ;
#11287=ORIENTED_EDGE('',*,*,#8307,.F.) ;
#11288=ORIENTED_EDGE('',*,*,#8308,.T.) ;
#11289=ORIENTED_EDGE('',*,*,#8309,.T.) ;
#11290=ORIENTED_EDGE('',*,*,#8310,.F.) ;
#11291=ORIENTED_EDGE('',*,*,#8311,.F.) ;
#11292=ORIENTED_EDGE('',*,*,#8312,.T.) ;
#11293=ORIENTED_EDGE('',*,*,#8313,.T.) ;
#11294=ORIENTED_EDGE('',*,*,#8314,.F.) ;
#11295=ORIENTED_EDGE('',*,*,#8315,.F.) ;
#11296=ORIENTED_EDGE('',*,*,#8316,.T.) ;
#11297=ORIENTED_EDGE('',*,*,#8317,.T.) ;
#11298=ORIENTED_EDGE('',*,*,#8318,.F.) ;
#11299=ORIENTED_EDGE('',*,*,#8319,.F.) ;
#11300=ORIENTED_EDGE('',*,*,#8320,.T.) ;
#11301=ORIENTED_EDGE('',*,*,#8321,.T.) ;
#11302=ORIENTED_EDGE('',*,*,#8322,.F.) ;
#11303=ORIENTED_EDGE('',*,*,#8323,.F.) ;
#11304=ORIENTED_EDGE('',*,*,#8324,.T.) ;
#11305=ORIENTED_EDGE('',*,*,#8325,.T.) ;
#11306=ORIENTED_EDGE('',*,*,#8326,.F.) ;
#11307=ORIENTED_EDGE('',*,*,#8327,.F.) ;
#11308=ORIENTED_EDGE('',*,*,#8328,.F.) ;
#11309=ORIENTED_EDGE('',*,*,#8329,.T.) ;
#11310=ORIENTED_EDGE('',*,*,#8330,.T.) ;
#11311=ORIENTED_EDGE('',*,*,#8331,.F.) ;
#11312=ORIENTED_EDGE('',*,*,#8332,.T.) ;
#11313=ORIENTED_EDGE('',*,*,#8333,.T.) ;
#11314=ORIENTED_EDGE('',*,*,#8334,.F.) ;
#11315=ORIENTED_EDGE('',*,*,#8335,.F.) ;
#11316=ORIENTED_EDGE('',*,*,#8336,.T.) ;
#11317=ORIENTED_EDGE('',*,*,#8093,.T.) ;
#11318=ORIENTED_EDGE('',*,*,#8336,.F.) ;
#11319=ORIENTED_EDGE('',*,*,#8337,.F.) ;
#11320=ORIENTED_EDGE('',*,*,#8335,.T.) ;
#11321=ORIENTED_EDGE('',*,*,#8337,.T.) ;
#11322=ORIENTED_EDGE('',*,*,#8338,.T.) ;
#11323=ORIENTED_EDGE('',*,*,#8339,.F.) ;
#11324=ORIENTED_EDGE('',*,*,#8340,.F.) ;
#11325=ORIENTED_EDGE('',*,*,#8338,.F.) ;
#11326=ORIENTED_EDGE('',*,*,#8341,.F.) ;
#11327=ORIENTED_EDGE('',*,*,#8342,.F.) ;
#11328=ORIENTED_EDGE('',*,*,#8343,.T.) ;
#11329=ORIENTED_EDGE('',*,*,#8339,.T.) ;
#11330=ORIENTED_EDGE('',*,*,#8340,.T.) ;
#11331=ORIENTED_EDGE('',*,*,#8343,.F.) ;
#11332=ORIENTED_EDGE('',*,*,#8341,.T.) ;
#11333=ORIENTED_EDGE('',*,*,#8342,.T.) ;
#11334=ORIENTED_EDGE('',*,*,#8344,.T.) ;
#11335=ORIENTED_EDGE('',*,*,#8345,.F.) ;
#11336=ORIENTED_EDGE('',*,*,#8269,.F.) ;
#11337=ORIENTED_EDGE('',*,*,#8346,.F.) ;
#11338=ORIENTED_EDGE('',*,*,#8265,.F.) ;
#11339=ORIENTED_EDGE('',*,*,#8347,.F.) ;
#11340=ORIENTED_EDGE('',*,*,#8261,.F.) ;
#11341=ORIENTED_EDGE('',*,*,#8348,.F.) ;
#11342=ORIENTED_EDGE('',*,*,#8257,.F.) ;
#11343=ORIENTED_EDGE('',*,*,#8349,.F.) ;
#11344=ORIENTED_EDGE('',*,*,#8226,.F.) ;
#11345=ORIENTED_EDGE('',*,*,#8350,.F.) ;
#11346=ORIENTED_EDGE('',*,*,#8230,.F.) ;
#11347=ORIENTED_EDGE('',*,*,#8351,.F.) ;
#11348=ORIENTED_EDGE('',*,*,#8234,.F.) ;
#11349=ORIENTED_EDGE('',*,*,#8352,.F.) ;
#11350=ORIENTED_EDGE('',*,*,#8238,.F.) ;
#11351=ORIENTED_EDGE('',*,*,#8353,.F.) ;
#11352=ORIENTED_EDGE('',*,*,#8242,.F.) ;
#11353=ORIENTED_EDGE('',*,*,#8354,.F.) ;
#11354=ORIENTED_EDGE('',*,*,#8246,.F.) ;
#11355=ORIENTED_EDGE('',*,*,#8355,.F.) ;
#11356=ORIENTED_EDGE('',*,*,#8250,.F.) ;
#11357=ORIENTED_EDGE('',*,*,#8356,.F.) ;
#11358=ORIENTED_EDGE('',*,*,#8253,.F.) ;
#11359=ORIENTED_EDGE('',*,*,#8357,.F.) ;
#11360=ORIENTED_EDGE('',*,*,#8221,.F.) ;
#11361=ORIENTED_EDGE('',*,*,#8358,.F.) ;
#11362=ORIENTED_EDGE('',*,*,#8217,.F.) ;
#11363=ORIENTED_EDGE('',*,*,#8359,.F.) ;
#11364=ORIENTED_EDGE('',*,*,#8213,.F.) ;
#11365=ORIENTED_EDGE('',*,*,#8360,.F.) ;
#11366=ORIENTED_EDGE('',*,*,#8209,.F.) ;
#11367=ORIENTED_EDGE('',*,*,#8361,.F.) ;
#11368=ORIENTED_EDGE('',*,*,#8205,.F.) ;
#11369=ORIENTED_EDGE('',*,*,#8362,.F.) ;
#11370=ORIENTED_EDGE('',*,*,#8201,.F.) ;
#11371=ORIENTED_EDGE('',*,*,#8363,.F.) ;
#11372=ORIENTED_EDGE('',*,*,#8197,.F.) ;
#11373=ORIENTED_EDGE('',*,*,#8364,.F.) ;
#11374=ORIENTED_EDGE('',*,*,#8193,.F.) ;
#11375=ORIENTED_EDGE('',*,*,#8365,.F.) ;
#11376=ORIENTED_EDGE('',*,*,#8189,.F.) ;
#11377=ORIENTED_EDGE('',*,*,#8366,.F.) ;
#11378=ORIENTED_EDGE('',*,*,#8185,.F.) ;
#11379=ORIENTED_EDGE('',*,*,#8367,.F.) ;
#11380=ORIENTED_EDGE('',*,*,#8178,.F.) ;
#11381=ORIENTED_EDGE('',*,*,#8368,.F.) ;
#11382=ORIENTED_EDGE('',*,*,#8181,.F.) ;
#11383=ORIENTED_EDGE('',*,*,#8369,.F.) ;
#11384=ORIENTED_EDGE('',*,*,#8173,.F.) ;
#11385=ORIENTED_EDGE('',*,*,#8370,.F.) ;
#11386=ORIENTED_EDGE('',*,*,#8169,.F.) ;
#11387=ORIENTED_EDGE('',*,*,#8371,.F.) ;
#11388=ORIENTED_EDGE('',*,*,#8165,.F.) ;
#11389=ORIENTED_EDGE('',*,*,#8372,.F.) ;
#11390=ORIENTED_EDGE('',*,*,#8161,.F.) ;
#11391=ORIENTED_EDGE('',*,*,#8373,.F.) ;
#11392=ORIENTED_EDGE('',*,*,#8157,.F.) ;
#11393=ORIENTED_EDGE('',*,*,#8374,.F.) ;
#11394=ORIENTED_EDGE('',*,*,#8153,.F.) ;
#11395=ORIENTED_EDGE('',*,*,#8375,.F.) ;
#11396=ORIENTED_EDGE('',*,*,#8149,.F.) ;
#11397=ORIENTED_EDGE('',*,*,#8376,.F.) ;
#11398=ORIENTED_EDGE('',*,*,#8145,.F.) ;
#11399=ORIENTED_EDGE('',*,*,#8377,.F.) ;
#11400=ORIENTED_EDGE('',*,*,#8141,.F.) ;
#11401=ORIENTED_EDGE('',*,*,#8378,.F.) ;
#11402=ORIENTED_EDGE('',*,*,#8137,.F.) ;
#11403=ORIENTED_EDGE('',*,*,#8379,.F.) ;
#11404=ORIENTED_EDGE('',*,*,#8133,.F.) ;
#11405=ORIENTED_EDGE('',*,*,#8380,.F.) ;
#11406=ORIENTED_EDGE('',*,*,#8129,.F.) ;
#11407=ORIENTED_EDGE('',*,*,#8381,.F.) ;
#11408=ORIENTED_EDGE('',*,*,#8114,.F.) ;
#11409=ORIENTED_EDGE('',*,*,#8382,.F.) ;
#11410=ORIENTED_EDGE('',*,*,#8118,.F.) ;
#11411=ORIENTED_EDGE('',*,*,#8383,.F.) ;
#11412=ORIENTED_EDGE('',*,*,#8122,.F.) ;
#11413=ORIENTED_EDGE('',*,*,#8384,.F.) ;
#11414=ORIENTED_EDGE('',*,*,#8125,.F.) ;
#11415=ORIENTED_EDGE('',*,*,#8385,.F.) ;
#11416=ORIENTED_EDGE('',*,*,#8109,.F.) ;
#11417=ORIENTED_EDGE('',*,*,#8386,.F.) ;
#11418=ORIENTED_EDGE('',*,*,#8105,.F.) ;
#11419=ORIENTED_EDGE('',*,*,#8387,.F.) ;
#11420=ORIENTED_EDGE('',*,*,#8101,.F.) ;
#11421=ORIENTED_EDGE('',*,*,#8388,.F.) ;
#11422=ORIENTED_EDGE('',*,*,#8098,.F.) ;
#11423=ORIENTED_EDGE('',*,*,#8389,.F.) ;
#11424=ORIENTED_EDGE('',*,*,#8330,.F.) ;
#11425=ORIENTED_EDGE('',*,*,#8390,.F.) ;
#11426=ORIENTED_EDGE('',*,*,#8333,.F.) ;
#11427=ORIENTED_EDGE('',*,*,#8391,.F.) ;
#11428=ORIENTED_EDGE('',*,*,#8325,.F.) ;
#11429=ORIENTED_EDGE('',*,*,#8392,.F.) ;
#11430=ORIENTED_EDGE('',*,*,#8321,.F.) ;
#11431=ORIENTED_EDGE('',*,*,#8393,.F.) ;
#11432=ORIENTED_EDGE('',*,*,#8317,.F.) ;
#11433=ORIENTED_EDGE('',*,*,#8394,.F.) ;
#11434=ORIENTED_EDGE('',*,*,#8313,.F.) ;
#11435=ORIENTED_EDGE('',*,*,#8395,.F.) ;
#11436=ORIENTED_EDGE('',*,*,#8309,.F.) ;
#11437=ORIENTED_EDGE('',*,*,#8396,.F.) ;
#11438=ORIENTED_EDGE('',*,*,#8305,.F.) ;
#11439=ORIENTED_EDGE('',*,*,#8397,.F.) ;
#11440=ORIENTED_EDGE('',*,*,#8298,.F.) ;
#11441=ORIENTED_EDGE('',*,*,#8398,.F.) ;
#11442=ORIENTED_EDGE('',*,*,#8301,.F.) ;
#11443=ORIENTED_EDGE('',*,*,#8399,.F.) ;
#11444=ORIENTED_EDGE('',*,*,#8293,.F.) ;
#11445=ORIENTED_EDGE('',*,*,#8400,.F.) ;
#11446=ORIENTED_EDGE('',*,*,#8289,.F.) ;
#11447=ORIENTED_EDGE('',*,*,#8401,.F.) ;
#11448=ORIENTED_EDGE('',*,*,#8285,.F.) ;
#11449=ORIENTED_EDGE('',*,*,#8402,.F.) ;
#11450=ORIENTED_EDGE('',*,*,#8281,.F.) ;
#11451=ORIENTED_EDGE('',*,*,#8403,.F.) ;
#11452=ORIENTED_EDGE('',*,*,#8277,.F.) ;
#11453=ORIENTED_EDGE('',*,*,#8404,.F.) ;
#11454=ORIENTED_EDGE('',*,*,#8273,.F.) ;
#11455=ORIENTED_EDGE('',*,*,#8405,.F.) ;
#11456=ORIENTED_EDGE('',*,*,#8344,.F.) ;
#11457=ORIENTED_EDGE('',*,*,#8406,.F.) ;
#11458=ORIENTED_EDGE('',*,*,#8407,.F.) ;
#11459=ORIENTED_EDGE('',*,*,#8408,.T.) ;
#11460=ORIENTED_EDGE('',*,*,#8409,.T.) ;
#11461=ORIENTED_EDGE('',*,*,#8151,.T.) ;
#11462=ORIENTED_EDGE('',*,*,#8410,.T.) ;
#11463=ORIENTED_EDGE('',*,*,#8155,.T.) ;
#11464=ORIENTED_EDGE('',*,*,#8411,.T.) ;
#11465=ORIENTED_EDGE('',*,*,#8159,.T.) ;
#11466=ORIENTED_EDGE('',*,*,#8412,.T.) ;
#11467=ORIENTED_EDGE('',*,*,#8163,.T.) ;
#11468=ORIENTED_EDGE('',*,*,#8413,.T.) ;
#11469=ORIENTED_EDGE('',*,*,#8167,.T.) ;
#11470=ORIENTED_EDGE('',*,*,#8414,.T.) ;
#11471=ORIENTED_EDGE('',*,*,#8171,.T.) ;
#11472=ORIENTED_EDGE('',*,*,#8415,.T.) ;
#11473=ORIENTED_EDGE('',*,*,#8179,.T.) ;
#11474=ORIENTED_EDGE('',*,*,#8416,.T.) ;
#11475=ORIENTED_EDGE('',*,*,#8176,.T.) ;
#11476=ORIENTED_EDGE('',*,*,#8417,.T.) ;
#11477=ORIENTED_EDGE('',*,*,#8183,.T.) ;
#11478=ORIENTED_EDGE('',*,*,#8418,.T.) ;
#11479=ORIENTED_EDGE('',*,*,#8187,.T.) ;
#11480=ORIENTED_EDGE('',*,*,#8419,.T.) ;
#11481=ORIENTED_EDGE('',*,*,#8191,.T.) ;
#11482=ORIENTED_EDGE('',*,*,#8420,.T.) ;
#11483=ORIENTED_EDGE('',*,*,#8195,.T.) ;
#11484=ORIENTED_EDGE('',*,*,#8421,.T.) ;
#11485=ORIENTED_EDGE('',*,*,#8199,.T.) ;
#11486=ORIENTED_EDGE('',*,*,#8422,.T.) ;
#11487=ORIENTED_EDGE('',*,*,#8203,.T.) ;
#11488=ORIENTED_EDGE('',*,*,#8423,.T.) ;
#11489=ORIENTED_EDGE('',*,*,#8207,.T.) ;
#11490=ORIENTED_EDGE('',*,*,#8424,.T.) ;
#11491=ORIENTED_EDGE('',*,*,#8211,.T.) ;
#11492=ORIENTED_EDGE('',*,*,#8425,.T.) ;
#11493=ORIENTED_EDGE('',*,*,#8215,.T.) ;
#11494=ORIENTED_EDGE('',*,*,#8426,.T.) ;
#11495=ORIENTED_EDGE('',*,*,#8219,.T.) ;
#11496=ORIENTED_EDGE('',*,*,#8427,.T.) ;
#11497=ORIENTED_EDGE('',*,*,#8251,.T.) ;
#11498=ORIENTED_EDGE('',*,*,#8428,.T.) ;
#11499=ORIENTED_EDGE('',*,*,#8248,.T.) ;
#11500=ORIENTED_EDGE('',*,*,#8429,.T.) ;
#11501=ORIENTED_EDGE('',*,*,#8244,.T.) ;
#11502=ORIENTED_EDGE('',*,*,#8430,.T.) ;
#11503=ORIENTED_EDGE('',*,*,#8240,.T.) ;
#11504=ORIENTED_EDGE('',*,*,#8431,.T.) ;
#11505=ORIENTED_EDGE('',*,*,#8236,.T.) ;
#11506=ORIENTED_EDGE('',*,*,#8432,.T.) ;
#11507=ORIENTED_EDGE('',*,*,#8232,.T.) ;
#11508=ORIENTED_EDGE('',*,*,#8433,.T.) ;
#11509=ORIENTED_EDGE('',*,*,#8228,.T.) ;
#11510=ORIENTED_EDGE('',*,*,#8434,.T.) ;
#11511=ORIENTED_EDGE('',*,*,#8224,.T.) ;
#11512=ORIENTED_EDGE('',*,*,#8435,.T.) ;
#11513=ORIENTED_EDGE('',*,*,#8255,.T.) ;
#11514=ORIENTED_EDGE('',*,*,#8436,.T.) ;
#11515=ORIENTED_EDGE('',*,*,#8259,.T.) ;
#11516=ORIENTED_EDGE('',*,*,#8437,.T.) ;
#11517=ORIENTED_EDGE('',*,*,#8263,.T.) ;
#11518=ORIENTED_EDGE('',*,*,#8438,.T.) ;
#11519=ORIENTED_EDGE('',*,*,#8267,.T.) ;
#11520=ORIENTED_EDGE('',*,*,#8439,.T.) ;
#11521=ORIENTED_EDGE('',*,*,#8271,.T.) ;
#11522=ORIENTED_EDGE('',*,*,#8440,.T.) ;
#11523=ORIENTED_EDGE('',*,*,#8275,.T.) ;
#11524=ORIENTED_EDGE('',*,*,#8441,.T.) ;
#11525=ORIENTED_EDGE('',*,*,#8279,.T.) ;
#11526=ORIENTED_EDGE('',*,*,#8442,.T.) ;
#11527=ORIENTED_EDGE('',*,*,#8283,.T.) ;
#11528=ORIENTED_EDGE('',*,*,#8443,.T.) ;
#11529=ORIENTED_EDGE('',*,*,#8287,.T.) ;
#11530=ORIENTED_EDGE('',*,*,#8444,.T.) ;
#11531=ORIENTED_EDGE('',*,*,#8291,.T.) ;
#11532=ORIENTED_EDGE('',*,*,#8445,.T.) ;
#11533=ORIENTED_EDGE('',*,*,#8299,.T.) ;
#11534=ORIENTED_EDGE('',*,*,#8446,.T.) ;
#11535=ORIENTED_EDGE('',*,*,#8296,.T.) ;
#11536=ORIENTED_EDGE('',*,*,#8447,.T.) ;
#11537=ORIENTED_EDGE('',*,*,#8303,.T.) ;
#11538=ORIENTED_EDGE('',*,*,#8448,.T.) ;
#11539=ORIENTED_EDGE('',*,*,#8307,.T.) ;
#11540=ORIENTED_EDGE('',*,*,#8449,.T.) ;
#11541=ORIENTED_EDGE('',*,*,#8311,.T.) ;
#11542=ORIENTED_EDGE('',*,*,#8450,.T.) ;
#11543=ORIENTED_EDGE('',*,*,#8315,.T.) ;
#11544=ORIENTED_EDGE('',*,*,#8451,.T.) ;
#11545=ORIENTED_EDGE('',*,*,#8319,.T.) ;
#11546=ORIENTED_EDGE('',*,*,#8452,.T.) ;
#11547=ORIENTED_EDGE('',*,*,#8323,.T.) ;
#11548=ORIENTED_EDGE('',*,*,#8453,.T.) ;
#11549=ORIENTED_EDGE('',*,*,#8331,.T.) ;
#11550=ORIENTED_EDGE('',*,*,#8454,.T.) ;
#11551=ORIENTED_EDGE('',*,*,#8328,.T.) ;
#11552=ORIENTED_EDGE('',*,*,#8455,.T.) ;
#11553=ORIENTED_EDGE('',*,*,#8096,.T.) ;
#11554=ORIENTED_EDGE('',*,*,#8456,.T.) ;
#11555=ORIENTED_EDGE('',*,*,#8099,.T.) ;
#11556=ORIENTED_EDGE('',*,*,#8457,.T.) ;
#11557=ORIENTED_EDGE('',*,*,#8103,.T.) ;
#11558=ORIENTED_EDGE('',*,*,#8458,.T.) ;
#11559=ORIENTED_EDGE('',*,*,#8107,.T.) ;
#11560=ORIENTED_EDGE('',*,*,#8459,.T.) ;
#11561=ORIENTED_EDGE('',*,*,#8123,.T.) ;
#11562=ORIENTED_EDGE('',*,*,#8460,.T.) ;
#11563=ORIENTED_EDGE('',*,*,#8120,.T.) ;
#11564=ORIENTED_EDGE('',*,*,#8461,.T.) ;
#11565=ORIENTED_EDGE('',*,*,#8116,.T.) ;
#11566=ORIENTED_EDGE('',*,*,#8462,.T.) ;
#11567=ORIENTED_EDGE('',*,*,#8112,.T.) ;
#11568=ORIENTED_EDGE('',*,*,#8463,.T.) ;
#11569=ORIENTED_EDGE('',*,*,#8127,.T.) ;
#11570=ORIENTED_EDGE('',*,*,#8464,.T.) ;
#11571=ORIENTED_EDGE('',*,*,#8131,.T.) ;
#11572=ORIENTED_EDGE('',*,*,#8465,.T.) ;
#11573=ORIENTED_EDGE('',*,*,#8135,.T.) ;
#11574=ORIENTED_EDGE('',*,*,#8466,.T.) ;
#11575=ORIENTED_EDGE('',*,*,#8139,.T.) ;
#11576=ORIENTED_EDGE('',*,*,#8467,.T.) ;
#11577=ORIENTED_EDGE('',*,*,#8143,.T.) ;
#11578=ORIENTED_EDGE('',*,*,#8468,.T.) ;
#11579=ORIENTED_EDGE('',*,*,#8147,.T.) ;
#11580=ORIENTED_EDGE('',*,*,#8469,.T.) ;
#11581=ORIENTED_EDGE('',*,*,#8408,.F.) ;
#11582=ORIENTED_EDGE('',*,*,#8406,.T.) ;
#11583=ORIENTED_EDGE('',*,*,#8407,.T.) ;
#11584=ORIENTED_EDGE('',*,*,#8470,.T.) ;
#11585=ORIENTED_EDGE('',*,*,#8471,.F.) ;
#11586=ORIENTED_EDGE('',*,*,#8472,.F.) ;
#11587=ORIENTED_EDGE('',*,*,#8470,.F.) ;
#11588=ORIENTED_EDGE('',*,*,#8473,.F.) ;
#11589=ORIENTED_EDGE('',*,*,#8474,.T.) ;
#11590=ORIENTED_EDGE('',*,*,#8471,.T.) ;
#11591=ORIENTED_EDGE('',*,*,#8472,.T.) ;
#11592=ORIENTED_EDGE('',*,*,#8474,.F.) ;
#11593=ORIENTED_EDGE('',*,*,#8473,.T.) ;
#11594=ORIENTED_EDGE('',*,*,#8475,.F.) ;
#11595=ORIENTED_EDGE('',*,*,#8476,.F.) ;
#11596=ORIENTED_EDGE('',*,*,#8477,.T.) ;
#11597=ORIENTED_EDGE('',*,*,#8475,.T.) ;
#11598=ORIENTED_EDGE('',*,*,#8477,.F.) ;
#11599=ORIENTED_EDGE('',*,*,#8476,.T.) ;
#11600=ORIENTED_EDGE('',*,*,#8478,.F.) ;
#11601=ORIENTED_EDGE('',*,*,#8479,.F.) ;
#11602=ORIENTED_EDGE('',*,*,#8480,.T.) ;
#11603=ORIENTED_EDGE('',*,*,#8478,.T.) ;
#11604=ORIENTED_EDGE('',*,*,#8480,.F.) ;
#11605=ORIENTED_EDGE('',*,*,#8479,.T.) ;
#11606=ORIENTED_EDGE('',*,*,#8091,.T.) ;
#11607=ORIENTED_EDGE('',*,*,#8481,.F.) ;
#11608=ORIENTED_EDGE('',*,*,#8086,.T.) ;
#11609=ORIENTED_EDGE('',*,*,#8089,.T.) ;
#11610=ORIENTED_EDGE('',*,*,#8482,.F.) ;
#11611=ORIENTED_EDGE('',*,*,#8390,.T.) ;
#11612=ORIENTED_EDGE('',*,*,#8483,.F.) ;
#11613=ORIENTED_EDGE('',*,*,#8484,.T.) ;
#11614=ORIENTED_EDGE('',*,*,#8485,.T.) ;
#11615=ORIENTED_EDGE('',*,*,#8486,.F.) ;
#11616=ORIENTED_EDGE('',*,*,#8487,.T.) ;
#11617=ORIENTED_EDGE('',*,*,#8454,.F.) ;
#11618=ORIENTED_EDGE('',*,*,#8483,.T.) ;
#11619=ORIENTED_EDGE('',*,*,#8329,.F.) ;
#11620=ORIENTED_EDGE('',*,*,#8487,.F.) ;
#11621=ORIENTED_EDGE('',*,*,#8488,.T.) ;
#11622=ORIENTED_EDGE('',*,*,#8484,.F.) ;
#11623=ORIENTED_EDGE('',*,*,#8488,.F.) ;
#11624=ORIENTED_EDGE('',*,*,#8486,.T.) ;
#11625=ORIENTED_EDGE('',*,*,#8489,.T.) ;
#11626=ORIENTED_EDGE('',*,*,#8482,.T.) ;
#11627=ORIENTED_EDGE('',*,*,#8489,.F.) ;
#11628=ORIENTED_EDGE('',*,*,#8485,.F.) ;
#11629=ORIENTED_EDGE('',*,*,#8334,.T.) ;
#11630=ORIENTED_EDGE('',*,*,#8389,.T.) ;
#11631=ORIENTED_EDGE('',*,*,#8490,.F.) ;
#11632=ORIENTED_EDGE('',*,*,#8491,.T.) ;
#11633=ORIENTED_EDGE('',*,*,#8492,.F.) ;
#11634=ORIENTED_EDGE('',*,*,#8493,.T.) ;
#11635=ORIENTED_EDGE('',*,*,#8494,.F.) ;
#11636=ORIENTED_EDGE('',*,*,#8495,.T.) ;
#11637=ORIENTED_EDGE('',*,*,#8455,.F.) ;
#11638=ORIENTED_EDGE('',*,*,#8490,.T.) ;
#11639=ORIENTED_EDGE('',*,*,#8097,.F.) ;
#11640=ORIENTED_EDGE('',*,*,#8495,.F.) ;
#11641=ORIENTED_EDGE('',*,*,#8496,.T.) ;
#11642=ORIENTED_EDGE('',*,*,#8491,.F.) ;
#11643=ORIENTED_EDGE('',*,*,#8496,.F.) ;
#11644=ORIENTED_EDGE('',*,*,#8494,.T.) ;
#11645=ORIENTED_EDGE('',*,*,#8497,.T.) ;
#11646=ORIENTED_EDGE('',*,*,#8492,.T.) ;
#11647=ORIENTED_EDGE('',*,*,#8497,.F.) ;
#11648=ORIENTED_EDGE('',*,*,#8493,.F.) ;
#11649=ORIENTED_EDGE('',*,*,#8327,.T.) ;
#11650=ORIENTED_EDGE('',*,*,#8391,.T.) ;
#11651=ORIENTED_EDGE('',*,*,#8498,.F.) ;
#11652=ORIENTED_EDGE('',*,*,#8499,.T.) ;
#11653=ORIENTED_EDGE('',*,*,#8500,.F.) ;
#11654=ORIENTED_EDGE('',*,*,#8501,.T.) ;
#11655=ORIENTED_EDGE('',*,*,#8502,.F.) ;
#11656=ORIENTED_EDGE('',*,*,#8503,.T.) ;
#11657=ORIENTED_EDGE('',*,*,#8453,.F.) ;
#11658=ORIENTED_EDGE('',*,*,#8498,.T.) ;
#11659=ORIENTED_EDGE('',*,*,#8332,.F.) ;
#11660=ORIENTED_EDGE('',*,*,#8503,.F.) ;
#11661=ORIENTED_EDGE('',*,*,#8504,.T.) ;
#11662=ORIENTED_EDGE('',*,*,#8499,.F.) ;
#11663=ORIENTED_EDGE('',*,*,#8504,.F.) ;
#11664=ORIENTED_EDGE('',*,*,#8502,.T.) ;
#11665=ORIENTED_EDGE('',*,*,#8505,.T.) ;
#11666=ORIENTED_EDGE('',*,*,#8500,.T.) ;
#11667=ORIENTED_EDGE('',*,*,#8505,.F.) ;
#11668=ORIENTED_EDGE('',*,*,#8501,.F.) ;
#11669=ORIENTED_EDGE('',*,*,#8326,.T.) ;
#11670=ORIENTED_EDGE('',*,*,#8392,.T.) ;
#11671=ORIENTED_EDGE('',*,*,#8506,.F.) ;
#11672=ORIENTED_EDGE('',*,*,#8507,.T.) ;
#11673=ORIENTED_EDGE('',*,*,#8508,.F.) ;
#11674=ORIENTED_EDGE('',*,*,#8509,.T.) ;
#11675=ORIENTED_EDGE('',*,*,#8510,.F.) ;
#11676=ORIENTED_EDGE('',*,*,#8511,.T.) ;
#11677=ORIENTED_EDGE('',*,*,#8452,.F.) ;
#11678=ORIENTED_EDGE('',*,*,#8506,.T.) ;
#11679=ORIENTED_EDGE('',*,*,#8324,.F.) ;
#11680=ORIENTED_EDGE('',*,*,#8511,.F.) ;
#11681=ORIENTED_EDGE('',*,*,#8512,.T.) ;
#11682=ORIENTED_EDGE('',*,*,#8507,.F.) ;
#11683=ORIENTED_EDGE('',*,*,#8512,.F.) ;
#11684=ORIENTED_EDGE('',*,*,#8510,.T.) ;
#11685=ORIENTED_EDGE('',*,*,#8513,.T.) ;
#11686=ORIENTED_EDGE('',*,*,#8508,.T.) ;
#11687=ORIENTED_EDGE('',*,*,#8513,.F.) ;
#11688=ORIENTED_EDGE('',*,*,#8509,.F.) ;
#11689=ORIENTED_EDGE('',*,*,#8322,.T.) ;
#11690=ORIENTED_EDGE('',*,*,#8393,.T.) ;
#11691=ORIENTED_EDGE('',*,*,#8514,.F.) ;
#11692=ORIENTED_EDGE('',*,*,#8515,.T.) ;
#11693=ORIENTED_EDGE('',*,*,#8516,.F.) ;
#11694=ORIENTED_EDGE('',*,*,#8517,.T.) ;
#11695=ORIENTED_EDGE('',*,*,#8518,.F.) ;
#11696=ORIENTED_EDGE('',*,*,#8519,.T.) ;
#11697=ORIENTED_EDGE('',*,*,#8451,.F.) ;
#11698=ORIENTED_EDGE('',*,*,#8514,.T.) ;
#11699=ORIENTED_EDGE('',*,*,#8320,.F.) ;
#11700=ORIENTED_EDGE('',*,*,#8519,.F.) ;
#11701=ORIENTED_EDGE('',*,*,#8520,.T.) ;
#11702=ORIENTED_EDGE('',*,*,#8515,.F.) ;
#11703=ORIENTED_EDGE('',*,*,#8520,.F.) ;
#11704=ORIENTED_EDGE('',*,*,#8518,.T.) ;
#11705=ORIENTED_EDGE('',*,*,#8521,.T.) ;
#11706=ORIENTED_EDGE('',*,*,#8516,.T.) ;
#11707=ORIENTED_EDGE('',*,*,#8521,.F.) ;
#11708=ORIENTED_EDGE('',*,*,#8517,.F.) ;
#11709=ORIENTED_EDGE('',*,*,#8318,.T.) ;
#11710=ORIENTED_EDGE('',*,*,#8394,.T.) ;
#11711=ORIENTED_EDGE('',*,*,#8522,.F.) ;
#11712=ORIENTED_EDGE('',*,*,#8523,.T.) ;
#11713=ORIENTED_EDGE('',*,*,#8524,.F.) ;
#11714=ORIENTED_EDGE('',*,*,#8525,.T.) ;
#11715=ORIENTED_EDGE('',*,*,#8526,.F.) ;
#11716=ORIENTED_EDGE('',*,*,#8527,.T.) ;
#11717=ORIENTED_EDGE('',*,*,#8450,.F.) ;
#11718=ORIENTED_EDGE('',*,*,#8522,.T.) ;
#11719=ORIENTED_EDGE('',*,*,#8316,.F.) ;
#11720=ORIENTED_EDGE('',*,*,#8527,.F.) ;
#11721=ORIENTED_EDGE('',*,*,#8528,.T.) ;
#11722=ORIENTED_EDGE('',*,*,#8523,.F.) ;
#11723=ORIENTED_EDGE('',*,*,#8528,.F.) ;
#11724=ORIENTED_EDGE('',*,*,#8526,.T.) ;
#11725=ORIENTED_EDGE('',*,*,#8529,.T.) ;
#11726=ORIENTED_EDGE('',*,*,#8524,.T.) ;
#11727=ORIENTED_EDGE('',*,*,#8529,.F.) ;
#11728=ORIENTED_EDGE('',*,*,#8525,.F.) ;
#11729=ORIENTED_EDGE('',*,*,#8314,.T.) ;
#11730=ORIENTED_EDGE('',*,*,#8395,.T.) ;
#11731=ORIENTED_EDGE('',*,*,#8530,.F.) ;
#11732=ORIENTED_EDGE('',*,*,#8531,.T.) ;
#11733=ORIENTED_EDGE('',*,*,#8532,.F.) ;
#11734=ORIENTED_EDGE('',*,*,#8533,.T.) ;
#11735=ORIENTED_EDGE('',*,*,#8534,.F.) ;
#11736=ORIENTED_EDGE('',*,*,#8535,.T.) ;
#11737=ORIENTED_EDGE('',*,*,#8449,.F.) ;
#11738=ORIENTED_EDGE('',*,*,#8530,.T.) ;
#11739=ORIENTED_EDGE('',*,*,#8312,.F.) ;
#11740=ORIENTED_EDGE('',*,*,#8535,.F.) ;
#11741=ORIENTED_EDGE('',*,*,#8536,.T.) ;
#11742=ORIENTED_EDGE('',*,*,#8531,.F.) ;
#11743=ORIENTED_EDGE('',*,*,#8536,.F.) ;
#11744=ORIENTED_EDGE('',*,*,#8534,.T.) ;
#11745=ORIENTED_EDGE('',*,*,#8537,.T.) ;
#11746=ORIENTED_EDGE('',*,*,#8532,.T.) ;
#11747=ORIENTED_EDGE('',*,*,#8537,.F.) ;
#11748=ORIENTED_EDGE('',*,*,#8533,.F.) ;
#11749=ORIENTED_EDGE('',*,*,#8310,.T.) ;
#11750=ORIENTED_EDGE('',*,*,#8396,.T.) ;
#11751=ORIENTED_EDGE('',*,*,#8538,.F.) ;
#11752=ORIENTED_EDGE('',*,*,#8539,.T.) ;
#11753=ORIENTED_EDGE('',*,*,#8540,.F.) ;
#11754=ORIENTED_EDGE('',*,*,#8541,.T.) ;
#11755=ORIENTED_EDGE('',*,*,#8542,.F.) ;
#11756=ORIENTED_EDGE('',*,*,#8543,.T.) ;
#11757=ORIENTED_EDGE('',*,*,#8448,.F.) ;
#11758=ORIENTED_EDGE('',*,*,#8538,.T.) ;
#11759=ORIENTED_EDGE('',*,*,#8308,.F.) ;
#11760=ORIENTED_EDGE('',*,*,#8543,.F.) ;
#11761=ORIENTED_EDGE('',*,*,#8544,.T.) ;
#11762=ORIENTED_EDGE('',*,*,#8539,.F.) ;
#11763=ORIENTED_EDGE('',*,*,#8544,.F.) ;
#11764=ORIENTED_EDGE('',*,*,#8542,.T.) ;
#11765=ORIENTED_EDGE('',*,*,#8545,.T.) ;
#11766=ORIENTED_EDGE('',*,*,#8540,.T.) ;
#11767=ORIENTED_EDGE('',*,*,#8545,.F.) ;
#11768=ORIENTED_EDGE('',*,*,#8541,.F.) ;
#11769=ORIENTED_EDGE('',*,*,#8306,.T.) ;
#11770=ORIENTED_EDGE('',*,*,#8398,.T.) ;
#11771=ORIENTED_EDGE('',*,*,#8546,.F.) ;
#11772=ORIENTED_EDGE('',*,*,#8547,.T.) ;
#11773=ORIENTED_EDGE('',*,*,#8548,.F.) ;
#11774=ORIENTED_EDGE('',*,*,#8549,.T.) ;
#11775=ORIENTED_EDGE('',*,*,#8550,.F.) ;
#11776=ORIENTED_EDGE('',*,*,#8551,.T.) ;
#11777=ORIENTED_EDGE('',*,*,#8446,.F.) ;
#11778=ORIENTED_EDGE('',*,*,#8546,.T.) ;
#11779=ORIENTED_EDGE('',*,*,#8297,.F.) ;
#11780=ORIENTED_EDGE('',*,*,#8551,.F.) ;
#11781=ORIENTED_EDGE('',*,*,#8552,.T.) ;
#11782=ORIENTED_EDGE('',*,*,#8547,.F.) ;
#11783=ORIENTED_EDGE('',*,*,#8552,.F.) ;
#11784=ORIENTED_EDGE('',*,*,#8550,.T.) ;
#11785=ORIENTED_EDGE('',*,*,#8553,.T.) ;
#11786=ORIENTED_EDGE('',*,*,#8548,.T.) ;
#11787=ORIENTED_EDGE('',*,*,#8553,.F.) ;
#11788=ORIENTED_EDGE('',*,*,#8549,.F.) ;
#11789=ORIENTED_EDGE('',*,*,#8302,.T.) ;
#11790=ORIENTED_EDGE('',*,*,#8397,.T.) ;
#11791=ORIENTED_EDGE('',*,*,#8554,.F.) ;
#11792=ORIENTED_EDGE('',*,*,#8555,.T.) ;
#11793=ORIENTED_EDGE('',*,*,#8556,.F.) ;
#11794=ORIENTED_EDGE('',*,*,#8557,.T.) ;
#11795=ORIENTED_EDGE('',*,*,#8558,.F.) ;
#11796=ORIENTED_EDGE('',*,*,#8559,.T.) ;
#11797=ORIENTED_EDGE('',*,*,#8447,.F.) ;
#11798=ORIENTED_EDGE('',*,*,#8554,.T.) ;
#11799=ORIENTED_EDGE('',*,*,#8304,.F.) ;
#11800=ORIENTED_EDGE('',*,*,#8559,.F.) ;
#11801=ORIENTED_EDGE('',*,*,#8560,.T.) ;
#11802=ORIENTED_EDGE('',*,*,#8555,.F.) ;
#11803=ORIENTED_EDGE('',*,*,#8560,.F.) ;
#11804=ORIENTED_EDGE('',*,*,#8558,.T.) ;
#11805=ORIENTED_EDGE('',*,*,#8561,.T.) ;
#11806=ORIENTED_EDGE('',*,*,#8556,.T.) ;
#11807=ORIENTED_EDGE('',*,*,#8561,.F.) ;
#11808=ORIENTED_EDGE('',*,*,#8557,.F.) ;
#11809=ORIENTED_EDGE('',*,*,#8295,.T.) ;
#11810=ORIENTED_EDGE('',*,*,#8399,.T.) ;
#11811=ORIENTED_EDGE('',*,*,#8562,.F.) ;
#11812=ORIENTED_EDGE('',*,*,#8563,.T.) ;
#11813=ORIENTED_EDGE('',*,*,#8564,.F.) ;
#11814=ORIENTED_EDGE('',*,*,#8565,.T.) ;
#11815=ORIENTED_EDGE('',*,*,#8566,.F.) ;
#11816=ORIENTED_EDGE('',*,*,#8567,.T.) ;
#11817=ORIENTED_EDGE('',*,*,#8445,.F.) ;
#11818=ORIENTED_EDGE('',*,*,#8562,.T.) ;
#11819=ORIENTED_EDGE('',*,*,#8300,.F.) ;
#11820=ORIENTED_EDGE('',*,*,#8567,.F.) ;
#11821=ORIENTED_EDGE('',*,*,#8568,.T.) ;
#11822=ORIENTED_EDGE('',*,*,#8563,.F.) ;
#11823=ORIENTED_EDGE('',*,*,#8568,.F.) ;
#11824=ORIENTED_EDGE('',*,*,#8566,.T.) ;
#11825=ORIENTED_EDGE('',*,*,#8569,.T.) ;
#11826=ORIENTED_EDGE('',*,*,#8564,.T.) ;
#11827=ORIENTED_EDGE('',*,*,#8569,.F.) ;
#11828=ORIENTED_EDGE('',*,*,#8565,.F.) ;
#11829=ORIENTED_EDGE('',*,*,#8294,.T.) ;
#11830=ORIENTED_EDGE('',*,*,#8400,.T.) ;
#11831=ORIENTED_EDGE('',*,*,#8570,.F.) ;
#11832=ORIENTED_EDGE('',*,*,#8571,.T.) ;
#11833=ORIENTED_EDGE('',*,*,#8572,.F.) ;
#11834=ORIENTED_EDGE('',*,*,#8573,.T.) ;
#11835=ORIENTED_EDGE('',*,*,#8574,.F.) ;
#11836=ORIENTED_EDGE('',*,*,#8575,.T.) ;
#11837=ORIENTED_EDGE('',*,*,#8444,.F.) ;
#11838=ORIENTED_EDGE('',*,*,#8570,.T.) ;
#11839=ORIENTED_EDGE('',*,*,#8292,.F.) ;
#11840=ORIENTED_EDGE('',*,*,#8575,.F.) ;
#11841=ORIENTED_EDGE('',*,*,#8576,.T.) ;
#11842=ORIENTED_EDGE('',*,*,#8571,.F.) ;
#11843=ORIENTED_EDGE('',*,*,#8576,.F.) ;
#11844=ORIENTED_EDGE('',*,*,#8574,.T.) ;
#11845=ORIENTED_EDGE('',*,*,#8577,.T.) ;
#11846=ORIENTED_EDGE('',*,*,#8572,.T.) ;
#11847=ORIENTED_EDGE('',*,*,#8577,.F.) ;
#11848=ORIENTED_EDGE('',*,*,#8573,.F.) ;
#11849=ORIENTED_EDGE('',*,*,#8290,.T.) ;
#11850=ORIENTED_EDGE('',*,*,#8401,.T.) ;
#11851=ORIENTED_EDGE('',*,*,#8578,.F.) ;
#11852=ORIENTED_EDGE('',*,*,#8579,.T.) ;
#11853=ORIENTED_EDGE('',*,*,#8580,.F.) ;
#11854=ORIENTED_EDGE('',*,*,#8581,.T.) ;
#11855=ORIENTED_EDGE('',*,*,#8582,.F.) ;
#11856=ORIENTED_EDGE('',*,*,#8583,.T.) ;
#11857=ORIENTED_EDGE('',*,*,#8443,.F.) ;
#11858=ORIENTED_EDGE('',*,*,#8578,.T.) ;
#11859=ORIENTED_EDGE('',*,*,#8288,.F.) ;
#11860=ORIENTED_EDGE('',*,*,#8583,.F.) ;
#11861=ORIENTED_EDGE('',*,*,#8584,.T.) ;
#11862=ORIENTED_EDGE('',*,*,#8579,.F.) ;
#11863=ORIENTED_EDGE('',*,*,#8584,.F.) ;
#11864=ORIENTED_EDGE('',*,*,#8582,.T.) ;
#11865=ORIENTED_EDGE('',*,*,#8585,.T.) ;
#11866=ORIENTED_EDGE('',*,*,#8580,.T.) ;
#11867=ORIENTED_EDGE('',*,*,#8585,.F.) ;
#11868=ORIENTED_EDGE('',*,*,#8581,.F.) ;
#11869=ORIENTED_EDGE('',*,*,#8286,.T.) ;
#11870=ORIENTED_EDGE('',*,*,#8402,.T.) ;
#11871=ORIENTED_EDGE('',*,*,#8586,.F.) ;
#11872=ORIENTED_EDGE('',*,*,#8587,.T.) ;
#11873=ORIENTED_EDGE('',*,*,#8588,.F.) ;
#11874=ORIENTED_EDGE('',*,*,#8589,.T.) ;
#11875=ORIENTED_EDGE('',*,*,#8590,.F.) ;
#11876=ORIENTED_EDGE('',*,*,#8591,.T.) ;
#11877=ORIENTED_EDGE('',*,*,#8442,.F.) ;
#11878=ORIENTED_EDGE('',*,*,#8586,.T.) ;
#11879=ORIENTED_EDGE('',*,*,#8284,.F.) ;
#11880=ORIENTED_EDGE('',*,*,#8591,.F.) ;
#11881=ORIENTED_EDGE('',*,*,#8592,.T.) ;
#11882=ORIENTED_EDGE('',*,*,#8587,.F.) ;
#11883=ORIENTED_EDGE('',*,*,#8592,.F.) ;
#11884=ORIENTED_EDGE('',*,*,#8590,.T.) ;
#11885=ORIENTED_EDGE('',*,*,#8593,.T.) ;
#11886=ORIENTED_EDGE('',*,*,#8588,.T.) ;
#11887=ORIENTED_EDGE('',*,*,#8593,.F.) ;
#11888=ORIENTED_EDGE('',*,*,#8589,.F.) ;
#11889=ORIENTED_EDGE('',*,*,#8282,.T.) ;
#11890=ORIENTED_EDGE('',*,*,#8403,.T.) ;
#11891=ORIENTED_EDGE('',*,*,#8594,.F.) ;
#11892=ORIENTED_EDGE('',*,*,#8595,.T.) ;
#11893=ORIENTED_EDGE('',*,*,#8596,.F.) ;
#11894=ORIENTED_EDGE('',*,*,#8597,.T.) ;
#11895=ORIENTED_EDGE('',*,*,#8598,.F.) ;
#11896=ORIENTED_EDGE('',*,*,#8599,.T.) ;
#11897=ORIENTED_EDGE('',*,*,#8441,.F.) ;
#11898=ORIENTED_EDGE('',*,*,#8594,.T.) ;
#11899=ORIENTED_EDGE('',*,*,#8280,.F.) ;
#11900=ORIENTED_EDGE('',*,*,#8599,.F.) ;
#11901=ORIENTED_EDGE('',*,*,#8600,.T.) ;
#11902=ORIENTED_EDGE('',*,*,#8595,.F.) ;
#11903=ORIENTED_EDGE('',*,*,#8600,.F.) ;
#11904=ORIENTED_EDGE('',*,*,#8598,.T.) ;
#11905=ORIENTED_EDGE('',*,*,#8601,.T.) ;
#11906=ORIENTED_EDGE('',*,*,#8596,.T.) ;
#11907=ORIENTED_EDGE('',*,*,#8601,.F.) ;
#11908=ORIENTED_EDGE('',*,*,#8597,.F.) ;
#11909=ORIENTED_EDGE('',*,*,#8278,.T.) ;
#11910=ORIENTED_EDGE('',*,*,#8404,.T.) ;
#11911=ORIENTED_EDGE('',*,*,#8602,.F.) ;
#11912=ORIENTED_EDGE('',*,*,#8603,.T.) ;
#11913=ORIENTED_EDGE('',*,*,#8604,.F.) ;
#11914=ORIENTED_EDGE('',*,*,#8605,.T.) ;
#11915=ORIENTED_EDGE('',*,*,#8606,.F.) ;
#11916=ORIENTED_EDGE('',*,*,#8607,.T.) ;
#11917=ORIENTED_EDGE('',*,*,#8440,.F.) ;
#11918=ORIENTED_EDGE('',*,*,#8602,.T.) ;
#11919=ORIENTED_EDGE('',*,*,#8276,.F.) ;
#11920=ORIENTED_EDGE('',*,*,#8607,.F.) ;
#11921=ORIENTED_EDGE('',*,*,#8608,.T.) ;
#11922=ORIENTED_EDGE('',*,*,#8603,.F.) ;
#11923=ORIENTED_EDGE('',*,*,#8608,.F.) ;
#11924=ORIENTED_EDGE('',*,*,#8606,.T.) ;
#11925=ORIENTED_EDGE('',*,*,#8609,.T.) ;
#11926=ORIENTED_EDGE('',*,*,#8604,.T.) ;
#11927=ORIENTED_EDGE('',*,*,#8609,.F.) ;
#11928=ORIENTED_EDGE('',*,*,#8605,.F.) ;
#11929=ORIENTED_EDGE('',*,*,#8274,.T.) ;
#11930=ORIENTED_EDGE('',*,*,#8345,.T.) ;
#11931=ORIENTED_EDGE('',*,*,#8405,.T.) ;
#11932=ORIENTED_EDGE('',*,*,#8610,.F.) ;
#11933=ORIENTED_EDGE('',*,*,#8611,.T.) ;
#11934=ORIENTED_EDGE('',*,*,#8612,.F.) ;
#11935=ORIENTED_EDGE('',*,*,#8613,.T.) ;
#11936=ORIENTED_EDGE('',*,*,#8614,.F.) ;
#11937=ORIENTED_EDGE('',*,*,#8615,.T.) ;
#11938=ORIENTED_EDGE('',*,*,#8439,.F.) ;
#11939=ORIENTED_EDGE('',*,*,#8610,.T.) ;
#11940=ORIENTED_EDGE('',*,*,#8272,.F.) ;
#11941=ORIENTED_EDGE('',*,*,#8615,.F.) ;
#11942=ORIENTED_EDGE('',*,*,#8616,.T.) ;
#11943=ORIENTED_EDGE('',*,*,#8611,.F.) ;
#11944=ORIENTED_EDGE('',*,*,#8616,.F.) ;
#11945=ORIENTED_EDGE('',*,*,#8614,.T.) ;
#11946=ORIENTED_EDGE('',*,*,#8617,.T.) ;
#11947=ORIENTED_EDGE('',*,*,#8612,.T.) ;
#11948=ORIENTED_EDGE('',*,*,#8617,.F.) ;
#11949=ORIENTED_EDGE('',*,*,#8613,.F.) ;
#11950=ORIENTED_EDGE('',*,*,#8270,.T.) ;
#11951=ORIENTED_EDGE('',*,*,#8346,.T.) ;
#11952=ORIENTED_EDGE('',*,*,#8618,.F.) ;
#11953=ORIENTED_EDGE('',*,*,#8619,.T.) ;
#11954=ORIENTED_EDGE('',*,*,#8620,.F.) ;
#11955=ORIENTED_EDGE('',*,*,#8621,.T.) ;
#11956=ORIENTED_EDGE('',*,*,#8622,.F.) ;
#11957=ORIENTED_EDGE('',*,*,#8623,.T.) ;
#11958=ORIENTED_EDGE('',*,*,#8438,.F.) ;
#11959=ORIENTED_EDGE('',*,*,#8618,.T.) ;
#11960=ORIENTED_EDGE('',*,*,#8268,.F.) ;
#11961=ORIENTED_EDGE('',*,*,#8623,.F.) ;
#11962=ORIENTED_EDGE('',*,*,#8624,.T.) ;
#11963=ORIENTED_EDGE('',*,*,#8619,.F.) ;
#11964=ORIENTED_EDGE('',*,*,#8624,.F.) ;
#11965=ORIENTED_EDGE('',*,*,#8622,.T.) ;
#11966=ORIENTED_EDGE('',*,*,#8625,.T.) ;
#11967=ORIENTED_EDGE('',*,*,#8620,.T.) ;
#11968=ORIENTED_EDGE('',*,*,#8625,.F.) ;
#11969=ORIENTED_EDGE('',*,*,#8621,.F.) ;
#11970=ORIENTED_EDGE('',*,*,#8266,.T.) ;
#11971=ORIENTED_EDGE('',*,*,#8347,.T.) ;
#11972=ORIENTED_EDGE('',*,*,#8626,.F.) ;
#11973=ORIENTED_EDGE('',*,*,#8627,.T.) ;
#11974=ORIENTED_EDGE('',*,*,#8628,.F.) ;
#11975=ORIENTED_EDGE('',*,*,#8629,.T.) ;
#11976=ORIENTED_EDGE('',*,*,#8630,.F.) ;
#11977=ORIENTED_EDGE('',*,*,#8631,.T.) ;
#11978=ORIENTED_EDGE('',*,*,#8437,.F.) ;
#11979=ORIENTED_EDGE('',*,*,#8626,.T.) ;
#11980=ORIENTED_EDGE('',*,*,#8264,.F.) ;
#11981=ORIENTED_EDGE('',*,*,#8631,.F.) ;
#11982=ORIENTED_EDGE('',*,*,#8632,.T.) ;
#11983=ORIENTED_EDGE('',*,*,#8627,.F.) ;
#11984=ORIENTED_EDGE('',*,*,#8632,.F.) ;
#11985=ORIENTED_EDGE('',*,*,#8630,.T.) ;
#11986=ORIENTED_EDGE('',*,*,#8633,.T.) ;
#11987=ORIENTED_EDGE('',*,*,#8628,.T.) ;
#11988=ORIENTED_EDGE('',*,*,#8633,.F.) ;
#11989=ORIENTED_EDGE('',*,*,#8629,.F.) ;
#11990=ORIENTED_EDGE('',*,*,#8262,.T.) ;
#11991=ORIENTED_EDGE('',*,*,#8348,.T.) ;
#11992=ORIENTED_EDGE('',*,*,#8634,.F.) ;
#11993=ORIENTED_EDGE('',*,*,#8635,.T.) ;
#11994=ORIENTED_EDGE('',*,*,#8636,.F.) ;
#11995=ORIENTED_EDGE('',*,*,#8637,.T.) ;
#11996=ORIENTED_EDGE('',*,*,#8638,.F.) ;
#11997=ORIENTED_EDGE('',*,*,#8639,.T.) ;
#11998=ORIENTED_EDGE('',*,*,#8436,.F.) ;
#11999=ORIENTED_EDGE('',*,*,#8634,.T.) ;
#12000=ORIENTED_EDGE('',*,*,#8260,.F.) ;
#12001=ORIENTED_EDGE('',*,*,#8639,.F.) ;
#12002=ORIENTED_EDGE('',*,*,#8640,.T.) ;
#12003=ORIENTED_EDGE('',*,*,#8635,.F.) ;
#12004=ORIENTED_EDGE('',*,*,#8640,.F.) ;
#12005=ORIENTED_EDGE('',*,*,#8638,.T.) ;
#12006=ORIENTED_EDGE('',*,*,#8641,.T.) ;
#12007=ORIENTED_EDGE('',*,*,#8636,.T.) ;
#12008=ORIENTED_EDGE('',*,*,#8641,.F.) ;
#12009=ORIENTED_EDGE('',*,*,#8637,.F.) ;
#12010=ORIENTED_EDGE('',*,*,#8258,.T.) ;
#12011=ORIENTED_EDGE('',*,*,#8356,.T.) ;
#12012=ORIENTED_EDGE('',*,*,#8642,.F.) ;
#12013=ORIENTED_EDGE('',*,*,#8643,.T.) ;
#12014=ORIENTED_EDGE('',*,*,#8644,.F.) ;
#12015=ORIENTED_EDGE('',*,*,#8645,.T.) ;
#12016=ORIENTED_EDGE('',*,*,#8646,.F.) ;
#12017=ORIENTED_EDGE('',*,*,#8647,.T.) ;
#12018=ORIENTED_EDGE('',*,*,#8428,.F.) ;
#12019=ORIENTED_EDGE('',*,*,#8642,.T.) ;
#12020=ORIENTED_EDGE('',*,*,#8249,.F.) ;
#12021=ORIENTED_EDGE('',*,*,#8647,.F.) ;
#12022=ORIENTED_EDGE('',*,*,#8648,.T.) ;
#12023=ORIENTED_EDGE('',*,*,#8643,.F.) ;
#12024=ORIENTED_EDGE('',*,*,#8648,.F.) ;
#12025=ORIENTED_EDGE('',*,*,#8646,.T.) ;
#12026=ORIENTED_EDGE('',*,*,#8649,.T.) ;
#12027=ORIENTED_EDGE('',*,*,#8644,.T.) ;
#12028=ORIENTED_EDGE('',*,*,#8649,.F.) ;
#12029=ORIENTED_EDGE('',*,*,#8645,.F.) ;
#12030=ORIENTED_EDGE('',*,*,#8254,.T.) ;
#12031=ORIENTED_EDGE('',*,*,#8355,.T.) ;
#12032=ORIENTED_EDGE('',*,*,#8650,.F.) ;
#12033=ORIENTED_EDGE('',*,*,#8651,.T.) ;
#12034=ORIENTED_EDGE('',*,*,#8652,.F.) ;
#12035=ORIENTED_EDGE('',*,*,#8653,.T.) ;
#12036=ORIENTED_EDGE('',*,*,#8654,.F.) ;
#12037=ORIENTED_EDGE('',*,*,#8655,.T.) ;
#12038=ORIENTED_EDGE('',*,*,#8429,.F.) ;
#12039=ORIENTED_EDGE('',*,*,#8650,.T.) ;
#12040=ORIENTED_EDGE('',*,*,#8245,.F.) ;
#12041=ORIENTED_EDGE('',*,*,#8655,.F.) ;
#12042=ORIENTED_EDGE('',*,*,#8656,.T.) ;
#12043=ORIENTED_EDGE('',*,*,#8651,.F.) ;
#12044=ORIENTED_EDGE('',*,*,#8656,.F.) ;
#12045=ORIENTED_EDGE('',*,*,#8654,.T.) ;
#12046=ORIENTED_EDGE('',*,*,#8657,.T.) ;
#12047=ORIENTED_EDGE('',*,*,#8652,.T.) ;
#12048=ORIENTED_EDGE('',*,*,#8657,.F.) ;
#12049=ORIENTED_EDGE('',*,*,#8653,.F.) ;
#12050=ORIENTED_EDGE('',*,*,#8247,.T.) ;
#12051=ORIENTED_EDGE('',*,*,#8354,.T.) ;
#12052=ORIENTED_EDGE('',*,*,#8658,.F.) ;
#12053=ORIENTED_EDGE('',*,*,#8659,.T.) ;
#12054=ORIENTED_EDGE('',*,*,#8660,.F.) ;
#12055=ORIENTED_EDGE('',*,*,#8661,.T.) ;
#12056=ORIENTED_EDGE('',*,*,#8662,.F.) ;
#12057=ORIENTED_EDGE('',*,*,#8663,.T.) ;
#12058=ORIENTED_EDGE('',*,*,#8430,.F.) ;
#12059=ORIENTED_EDGE('',*,*,#8658,.T.) ;
#12060=ORIENTED_EDGE('',*,*,#8241,.F.) ;
#12061=ORIENTED_EDGE('',*,*,#8663,.F.) ;
#12062=ORIENTED_EDGE('',*,*,#8664,.T.) ;
#12063=ORIENTED_EDGE('',*,*,#8659,.F.) ;
#12064=ORIENTED_EDGE('',*,*,#8664,.F.) ;
#12065=ORIENTED_EDGE('',*,*,#8662,.T.) ;
#12066=ORIENTED_EDGE('',*,*,#8665,.T.) ;
#12067=ORIENTED_EDGE('',*,*,#8660,.T.) ;
#12068=ORIENTED_EDGE('',*,*,#8665,.F.) ;
#12069=ORIENTED_EDGE('',*,*,#8661,.F.) ;
#12070=ORIENTED_EDGE('',*,*,#8243,.T.) ;
#12071=ORIENTED_EDGE('',*,*,#8353,.T.) ;
#12072=ORIENTED_EDGE('',*,*,#8666,.F.) ;
#12073=ORIENTED_EDGE('',*,*,#8667,.T.) ;
#12074=ORIENTED_EDGE('',*,*,#8668,.F.) ;
#12075=ORIENTED_EDGE('',*,*,#8669,.T.) ;
#12076=ORIENTED_EDGE('',*,*,#8670,.F.) ;
#12077=ORIENTED_EDGE('',*,*,#8671,.T.) ;
#12078=ORIENTED_EDGE('',*,*,#8431,.F.) ;
#12079=ORIENTED_EDGE('',*,*,#8666,.T.) ;
#12080=ORIENTED_EDGE('',*,*,#8237,.F.) ;
#12081=ORIENTED_EDGE('',*,*,#8671,.F.) ;
#12082=ORIENTED_EDGE('',*,*,#8672,.T.) ;
#12083=ORIENTED_EDGE('',*,*,#8667,.F.) ;
#12084=ORIENTED_EDGE('',*,*,#8672,.F.) ;
#12085=ORIENTED_EDGE('',*,*,#8670,.T.) ;
#12086=ORIENTED_EDGE('',*,*,#8673,.T.) ;
#12087=ORIENTED_EDGE('',*,*,#8668,.T.) ;
#12088=ORIENTED_EDGE('',*,*,#8673,.F.) ;
#12089=ORIENTED_EDGE('',*,*,#8669,.F.) ;
#12090=ORIENTED_EDGE('',*,*,#8239,.T.) ;
#12091=ORIENTED_EDGE('',*,*,#8352,.T.) ;
#12092=ORIENTED_EDGE('',*,*,#8674,.F.) ;
#12093=ORIENTED_EDGE('',*,*,#8675,.T.) ;
#12094=ORIENTED_EDGE('',*,*,#8676,.F.) ;
#12095=ORIENTED_EDGE('',*,*,#8677,.T.) ;
#12096=ORIENTED_EDGE('',*,*,#8678,.F.) ;
#12097=ORIENTED_EDGE('',*,*,#8679,.T.) ;
#12098=ORIENTED_EDGE('',*,*,#8432,.F.) ;
#12099=ORIENTED_EDGE('',*,*,#8674,.T.) ;
#12100=ORIENTED_EDGE('',*,*,#8233,.F.) ;
#12101=ORIENTED_EDGE('',*,*,#8679,.F.) ;
#12102=ORIENTED_EDGE('',*,*,#8680,.T.) ;
#12103=ORIENTED_EDGE('',*,*,#8675,.F.) ;
#12104=ORIENTED_EDGE('',*,*,#8680,.F.) ;
#12105=ORIENTED_EDGE('',*,*,#8678,.T.) ;
#12106=ORIENTED_EDGE('',*,*,#8681,.T.) ;
#12107=ORIENTED_EDGE('',*,*,#8676,.T.) ;
#12108=ORIENTED_EDGE('',*,*,#8681,.F.) ;
#12109=ORIENTED_EDGE('',*,*,#8677,.F.) ;
#12110=ORIENTED_EDGE('',*,*,#8235,.T.) ;
#12111=ORIENTED_EDGE('',*,*,#8351,.T.) ;
#12112=ORIENTED_EDGE('',*,*,#8682,.F.) ;
#12113=ORIENTED_EDGE('',*,*,#8683,.T.) ;
#12114=ORIENTED_EDGE('',*,*,#8684,.F.) ;
#12115=ORIENTED_EDGE('',*,*,#8685,.T.) ;
#12116=ORIENTED_EDGE('',*,*,#8686,.F.) ;
#12117=ORIENTED_EDGE('',*,*,#8687,.T.) ;
#12118=ORIENTED_EDGE('',*,*,#8433,.F.) ;
#12119=ORIENTED_EDGE('',*,*,#8682,.T.) ;
#12120=ORIENTED_EDGE('',*,*,#8229,.F.) ;
#12121=ORIENTED_EDGE('',*,*,#8687,.F.) ;
#12122=ORIENTED_EDGE('',*,*,#8688,.T.) ;
#12123=ORIENTED_EDGE('',*,*,#8683,.F.) ;
#12124=ORIENTED_EDGE('',*,*,#8688,.F.) ;
#12125=ORIENTED_EDGE('',*,*,#8686,.T.) ;
#12126=ORIENTED_EDGE('',*,*,#8689,.T.) ;
#12127=ORIENTED_EDGE('',*,*,#8684,.T.) ;
#12128=ORIENTED_EDGE('',*,*,#8689,.F.) ;
#12129=ORIENTED_EDGE('',*,*,#8685,.F.) ;
#12130=ORIENTED_EDGE('',*,*,#8231,.T.) ;
#12131=ORIENTED_EDGE('',*,*,#8350,.T.) ;
#12132=ORIENTED_EDGE('',*,*,#8690,.F.) ;
#12133=ORIENTED_EDGE('',*,*,#8691,.T.) ;
#12134=ORIENTED_EDGE('',*,*,#8692,.F.) ;
#12135=ORIENTED_EDGE('',*,*,#8693,.T.) ;
#12136=ORIENTED_EDGE('',*,*,#8694,.F.) ;
#12137=ORIENTED_EDGE('',*,*,#8695,.T.) ;
#12138=ORIENTED_EDGE('',*,*,#8434,.F.) ;
#12139=ORIENTED_EDGE('',*,*,#8690,.T.) ;
#12140=ORIENTED_EDGE('',*,*,#8225,.F.) ;
#12141=ORIENTED_EDGE('',*,*,#8695,.F.) ;
#12142=ORIENTED_EDGE('',*,*,#8696,.T.) ;
#12143=ORIENTED_EDGE('',*,*,#8691,.F.) ;
#12144=ORIENTED_EDGE('',*,*,#8696,.F.) ;
#12145=ORIENTED_EDGE('',*,*,#8694,.T.) ;
#12146=ORIENTED_EDGE('',*,*,#8697,.T.) ;
#12147=ORIENTED_EDGE('',*,*,#8692,.T.) ;
#12148=ORIENTED_EDGE('',*,*,#8697,.F.) ;
#12149=ORIENTED_EDGE('',*,*,#8693,.F.) ;
#12150=ORIENTED_EDGE('',*,*,#8227,.T.) ;
#12151=ORIENTED_EDGE('',*,*,#8349,.T.) ;
#12152=ORIENTED_EDGE('',*,*,#8698,.F.) ;
#12153=ORIENTED_EDGE('',*,*,#8699,.T.) ;
#12154=ORIENTED_EDGE('',*,*,#8700,.F.) ;
#12155=ORIENTED_EDGE('',*,*,#8701,.T.) ;
#12156=ORIENTED_EDGE('',*,*,#8702,.F.) ;
#12157=ORIENTED_EDGE('',*,*,#8703,.T.) ;
#12158=ORIENTED_EDGE('',*,*,#8435,.F.) ;
#12159=ORIENTED_EDGE('',*,*,#8698,.T.) ;
#12160=ORIENTED_EDGE('',*,*,#8256,.F.) ;
#12161=ORIENTED_EDGE('',*,*,#8703,.F.) ;
#12162=ORIENTED_EDGE('',*,*,#8704,.T.) ;
#12163=ORIENTED_EDGE('',*,*,#8699,.F.) ;
#12164=ORIENTED_EDGE('',*,*,#8704,.F.) ;
#12165=ORIENTED_EDGE('',*,*,#8702,.T.) ;
#12166=ORIENTED_EDGE('',*,*,#8705,.T.) ;
#12167=ORIENTED_EDGE('',*,*,#8700,.T.) ;
#12168=ORIENTED_EDGE('',*,*,#8705,.F.) ;
#12169=ORIENTED_EDGE('',*,*,#8701,.F.) ;
#12170=ORIENTED_EDGE('',*,*,#8223,.T.) ;
#12171=ORIENTED_EDGE('',*,*,#8357,.T.) ;
#12172=ORIENTED_EDGE('',*,*,#8706,.F.) ;
#12173=ORIENTED_EDGE('',*,*,#8707,.T.) ;
#12174=ORIENTED_EDGE('',*,*,#8708,.F.) ;
#12175=ORIENTED_EDGE('',*,*,#8709,.T.) ;
#12176=ORIENTED_EDGE('',*,*,#8710,.F.) ;
#12177=ORIENTED_EDGE('',*,*,#8711,.T.) ;
#12178=ORIENTED_EDGE('',*,*,#8427,.F.) ;
#12179=ORIENTED_EDGE('',*,*,#8706,.T.) ;
#12180=ORIENTED_EDGE('',*,*,#8252,.F.) ;
#12181=ORIENTED_EDGE('',*,*,#8711,.F.) ;
#12182=ORIENTED_EDGE('',*,*,#8712,.T.) ;
#12183=ORIENTED_EDGE('',*,*,#8707,.F.) ;
#12184=ORIENTED_EDGE('',*,*,#8712,.F.) ;
#12185=ORIENTED_EDGE('',*,*,#8710,.T.) ;
#12186=ORIENTED_EDGE('',*,*,#8713,.T.) ;
#12187=ORIENTED_EDGE('',*,*,#8708,.T.) ;
#12188=ORIENTED_EDGE('',*,*,#8713,.F.) ;
#12189=ORIENTED_EDGE('',*,*,#8709,.F.) ;
#12190=ORIENTED_EDGE('',*,*,#8222,.T.) ;
#12191=ORIENTED_EDGE('',*,*,#8358,.T.) ;
#12192=ORIENTED_EDGE('',*,*,#8714,.F.) ;
#12193=ORIENTED_EDGE('',*,*,#8715,.T.) ;
#12194=ORIENTED_EDGE('',*,*,#8716,.F.) ;
#12195=ORIENTED_EDGE('',*,*,#8717,.T.) ;
#12196=ORIENTED_EDGE('',*,*,#8718,.F.) ;
#12197=ORIENTED_EDGE('',*,*,#8719,.T.) ;
#12198=ORIENTED_EDGE('',*,*,#8426,.F.) ;
#12199=ORIENTED_EDGE('',*,*,#8714,.T.) ;
#12200=ORIENTED_EDGE('',*,*,#8220,.F.) ;
#12201=ORIENTED_EDGE('',*,*,#8719,.F.) ;
#12202=ORIENTED_EDGE('',*,*,#8720,.T.) ;
#12203=ORIENTED_EDGE('',*,*,#8715,.F.) ;
#12204=ORIENTED_EDGE('',*,*,#8720,.F.) ;
#12205=ORIENTED_EDGE('',*,*,#8718,.T.) ;
#12206=ORIENTED_EDGE('',*,*,#8721,.T.) ;
#12207=ORIENTED_EDGE('',*,*,#8716,.T.) ;
#12208=ORIENTED_EDGE('',*,*,#8721,.F.) ;
#12209=ORIENTED_EDGE('',*,*,#8717,.F.) ;
#12210=ORIENTED_EDGE('',*,*,#8218,.T.) ;
#12211=ORIENTED_EDGE('',*,*,#8359,.T.) ;
#12212=ORIENTED_EDGE('',*,*,#8722,.F.) ;
#12213=ORIENTED_EDGE('',*,*,#8723,.T.) ;
#12214=ORIENTED_EDGE('',*,*,#8724,.F.) ;
#12215=ORIENTED_EDGE('',*,*,#8725,.T.) ;
#12216=ORIENTED_EDGE('',*,*,#8726,.F.) ;
#12217=ORIENTED_EDGE('',*,*,#8727,.T.) ;
#12218=ORIENTED_EDGE('',*,*,#8425,.F.) ;
#12219=ORIENTED_EDGE('',*,*,#8722,.T.) ;
#12220=ORIENTED_EDGE('',*,*,#8216,.F.) ;
#12221=ORIENTED_EDGE('',*,*,#8727,.F.) ;
#12222=ORIENTED_EDGE('',*,*,#8728,.T.) ;
#12223=ORIENTED_EDGE('',*,*,#8723,.F.) ;
#12224=ORIENTED_EDGE('',*,*,#8728,.F.) ;
#12225=ORIENTED_EDGE('',*,*,#8726,.T.) ;
#12226=ORIENTED_EDGE('',*,*,#8729,.T.) ;
#12227=ORIENTED_EDGE('',*,*,#8724,.T.) ;
#12228=ORIENTED_EDGE('',*,*,#8729,.F.) ;
#12229=ORIENTED_EDGE('',*,*,#8725,.F.) ;
#12230=ORIENTED_EDGE('',*,*,#8214,.T.) ;
#12231=ORIENTED_EDGE('',*,*,#8360,.T.) ;
#12232=ORIENTED_EDGE('',*,*,#8730,.F.) ;
#12233=ORIENTED_EDGE('',*,*,#8731,.T.) ;
#12234=ORIENTED_EDGE('',*,*,#8732,.F.) ;
#12235=ORIENTED_EDGE('',*,*,#8733,.T.) ;
#12236=ORIENTED_EDGE('',*,*,#8734,.F.) ;
#12237=ORIENTED_EDGE('',*,*,#8735,.T.) ;
#12238=ORIENTED_EDGE('',*,*,#8424,.F.) ;
#12239=ORIENTED_EDGE('',*,*,#8730,.T.) ;
#12240=ORIENTED_EDGE('',*,*,#8212,.F.) ;
#12241=ORIENTED_EDGE('',*,*,#8735,.F.) ;
#12242=ORIENTED_EDGE('',*,*,#8736,.T.) ;
#12243=ORIENTED_EDGE('',*,*,#8731,.F.) ;
#12244=ORIENTED_EDGE('',*,*,#8736,.F.) ;
#12245=ORIENTED_EDGE('',*,*,#8734,.T.) ;
#12246=ORIENTED_EDGE('',*,*,#8737,.T.) ;
#12247=ORIENTED_EDGE('',*,*,#8732,.T.) ;
#12248=ORIENTED_EDGE('',*,*,#8737,.F.) ;
#12249=ORIENTED_EDGE('',*,*,#8733,.F.) ;
#12250=ORIENTED_EDGE('',*,*,#8210,.T.) ;
#12251=ORIENTED_EDGE('',*,*,#8361,.T.) ;
#12252=ORIENTED_EDGE('',*,*,#8738,.F.) ;
#12253=ORIENTED_EDGE('',*,*,#8739,.T.) ;
#12254=ORIENTED_EDGE('',*,*,#8740,.F.) ;
#12255=ORIENTED_EDGE('',*,*,#8741,.T.) ;
#12256=ORIENTED_EDGE('',*,*,#8742,.F.) ;
#12257=ORIENTED_EDGE('',*,*,#8743,.T.) ;
#12258=ORIENTED_EDGE('',*,*,#8423,.F.) ;
#12259=ORIENTED_EDGE('',*,*,#8738,.T.) ;
#12260=ORIENTED_EDGE('',*,*,#8208,.F.) ;
#12261=ORIENTED_EDGE('',*,*,#8743,.F.) ;
#12262=ORIENTED_EDGE('',*,*,#8744,.T.) ;
#12263=ORIENTED_EDGE('',*,*,#8739,.F.) ;
#12264=ORIENTED_EDGE('',*,*,#8744,.F.) ;
#12265=ORIENTED_EDGE('',*,*,#8742,.T.) ;
#12266=ORIENTED_EDGE('',*,*,#8745,.T.) ;
#12267=ORIENTED_EDGE('',*,*,#8740,.T.) ;
#12268=ORIENTED_EDGE('',*,*,#8745,.F.) ;
#12269=ORIENTED_EDGE('',*,*,#8741,.F.) ;
#12270=ORIENTED_EDGE('',*,*,#8206,.T.) ;
#12271=ORIENTED_EDGE('',*,*,#8362,.T.) ;
#12272=ORIENTED_EDGE('',*,*,#8746,.F.) ;
#12273=ORIENTED_EDGE('',*,*,#8747,.T.) ;
#12274=ORIENTED_EDGE('',*,*,#8748,.F.) ;
#12275=ORIENTED_EDGE('',*,*,#8749,.T.) ;
#12276=ORIENTED_EDGE('',*,*,#8750,.F.) ;
#12277=ORIENTED_EDGE('',*,*,#8751,.T.) ;
#12278=ORIENTED_EDGE('',*,*,#8422,.F.) ;
#12279=ORIENTED_EDGE('',*,*,#8746,.T.) ;
#12280=ORIENTED_EDGE('',*,*,#8204,.F.) ;
#12281=ORIENTED_EDGE('',*,*,#8751,.F.) ;
#12282=ORIENTED_EDGE('',*,*,#8752,.T.) ;
#12283=ORIENTED_EDGE('',*,*,#8747,.F.) ;
#12284=ORIENTED_EDGE('',*,*,#8752,.F.) ;
#12285=ORIENTED_EDGE('',*,*,#8750,.T.) ;
#12286=ORIENTED_EDGE('',*,*,#8753,.T.) ;
#12287=ORIENTED_EDGE('',*,*,#8748,.T.) ;
#12288=ORIENTED_EDGE('',*,*,#8753,.F.) ;
#12289=ORIENTED_EDGE('',*,*,#8749,.F.) ;
#12290=ORIENTED_EDGE('',*,*,#8202,.T.) ;
#12291=ORIENTED_EDGE('',*,*,#8363,.T.) ;
#12292=ORIENTED_EDGE('',*,*,#8754,.F.) ;
#12293=ORIENTED_EDGE('',*,*,#8755,.T.) ;
#12294=ORIENTED_EDGE('',*,*,#8756,.F.) ;
#12295=ORIENTED_EDGE('',*,*,#8757,.T.) ;
#12296=ORIENTED_EDGE('',*,*,#8758,.F.) ;
#12297=ORIENTED_EDGE('',*,*,#8759,.T.) ;
#12298=ORIENTED_EDGE('',*,*,#8421,.F.) ;
#12299=ORIENTED_EDGE('',*,*,#8754,.T.) ;
#12300=ORIENTED_EDGE('',*,*,#8200,.F.) ;
#12301=ORIENTED_EDGE('',*,*,#8759,.F.) ;
#12302=ORIENTED_EDGE('',*,*,#8760,.T.) ;
#12303=ORIENTED_EDGE('',*,*,#8755,.F.) ;
#12304=ORIENTED_EDGE('',*,*,#8760,.F.) ;
#12305=ORIENTED_EDGE('',*,*,#8758,.T.) ;
#12306=ORIENTED_EDGE('',*,*,#8761,.T.) ;
#12307=ORIENTED_EDGE('',*,*,#8756,.T.) ;
#12308=ORIENTED_EDGE('',*,*,#8761,.F.) ;
#12309=ORIENTED_EDGE('',*,*,#8757,.F.) ;
#12310=ORIENTED_EDGE('',*,*,#8198,.T.) ;
#12311=ORIENTED_EDGE('',*,*,#8364,.T.) ;
#12312=ORIENTED_EDGE('',*,*,#8762,.F.) ;
#12313=ORIENTED_EDGE('',*,*,#8763,.T.) ;
#12314=ORIENTED_EDGE('',*,*,#8764,.F.) ;
#12315=ORIENTED_EDGE('',*,*,#8765,.T.) ;
#12316=ORIENTED_EDGE('',*,*,#8766,.F.) ;
#12317=ORIENTED_EDGE('',*,*,#8767,.T.) ;
#12318=ORIENTED_EDGE('',*,*,#8420,.F.) ;
#12319=ORIENTED_EDGE('',*,*,#8762,.T.) ;
#12320=ORIENTED_EDGE('',*,*,#8196,.F.) ;
#12321=ORIENTED_EDGE('',*,*,#8767,.F.) ;
#12322=ORIENTED_EDGE('',*,*,#8768,.T.) ;
#12323=ORIENTED_EDGE('',*,*,#8763,.F.) ;
#12324=ORIENTED_EDGE('',*,*,#8768,.F.) ;
#12325=ORIENTED_EDGE('',*,*,#8766,.T.) ;
#12326=ORIENTED_EDGE('',*,*,#8769,.T.) ;
#12327=ORIENTED_EDGE('',*,*,#8764,.T.) ;
#12328=ORIENTED_EDGE('',*,*,#8769,.F.) ;
#12329=ORIENTED_EDGE('',*,*,#8765,.F.) ;
#12330=ORIENTED_EDGE('',*,*,#8194,.T.) ;
#12331=ORIENTED_EDGE('',*,*,#8365,.T.) ;
#12332=ORIENTED_EDGE('',*,*,#8770,.F.) ;
#12333=ORIENTED_EDGE('',*,*,#8771,.T.) ;
#12334=ORIENTED_EDGE('',*,*,#8772,.F.) ;
#12335=ORIENTED_EDGE('',*,*,#8773,.T.) ;
#12336=ORIENTED_EDGE('',*,*,#8774,.F.) ;
#12337=ORIENTED_EDGE('',*,*,#8775,.T.) ;
#12338=ORIENTED_EDGE('',*,*,#8419,.F.) ;
#12339=ORIENTED_EDGE('',*,*,#8770,.T.) ;
#12340=ORIENTED_EDGE('',*,*,#8192,.F.) ;
#12341=ORIENTED_EDGE('',*,*,#8775,.F.) ;
#12342=ORIENTED_EDGE('',*,*,#8776,.T.) ;
#12343=ORIENTED_EDGE('',*,*,#8771,.F.) ;
#12344=ORIENTED_EDGE('',*,*,#8776,.F.) ;
#12345=ORIENTED_EDGE('',*,*,#8774,.T.) ;
#12346=ORIENTED_EDGE('',*,*,#8777,.T.) ;
#12347=ORIENTED_EDGE('',*,*,#8772,.T.) ;
#12348=ORIENTED_EDGE('',*,*,#8777,.F.) ;
#12349=ORIENTED_EDGE('',*,*,#8773,.F.) ;
#12350=ORIENTED_EDGE('',*,*,#8190,.T.) ;
#12351=ORIENTED_EDGE('',*,*,#8366,.T.) ;
#12352=ORIENTED_EDGE('',*,*,#8778,.F.) ;
#12353=ORIENTED_EDGE('',*,*,#8779,.T.) ;
#12354=ORIENTED_EDGE('',*,*,#8780,.F.) ;
#12355=ORIENTED_EDGE('',*,*,#8781,.T.) ;
#12356=ORIENTED_EDGE('',*,*,#8782,.F.) ;
#12357=ORIENTED_EDGE('',*,*,#8783,.T.) ;
#12358=ORIENTED_EDGE('',*,*,#8418,.F.) ;
#12359=ORIENTED_EDGE('',*,*,#8778,.T.) ;
#12360=ORIENTED_EDGE('',*,*,#8188,.F.) ;
#12361=ORIENTED_EDGE('',*,*,#8783,.F.) ;
#12362=ORIENTED_EDGE('',*,*,#8784,.T.) ;
#12363=ORIENTED_EDGE('',*,*,#8779,.F.) ;
#12364=ORIENTED_EDGE('',*,*,#8784,.F.) ;
#12365=ORIENTED_EDGE('',*,*,#8782,.T.) ;
#12366=ORIENTED_EDGE('',*,*,#8785,.T.) ;
#12367=ORIENTED_EDGE('',*,*,#8780,.T.) ;
#12368=ORIENTED_EDGE('',*,*,#8785,.F.) ;
#12369=ORIENTED_EDGE('',*,*,#8781,.F.) ;
#12370=ORIENTED_EDGE('',*,*,#8186,.T.) ;
#12371=ORIENTED_EDGE('',*,*,#8368,.T.) ;
#12372=ORIENTED_EDGE('',*,*,#8786,.F.) ;
#12373=ORIENTED_EDGE('',*,*,#8787,.T.) ;
#12374=ORIENTED_EDGE('',*,*,#8788,.F.) ;
#12375=ORIENTED_EDGE('',*,*,#8789,.T.) ;
#12376=ORIENTED_EDGE('',*,*,#8790,.F.) ;
#12377=ORIENTED_EDGE('',*,*,#8791,.T.) ;
#12378=ORIENTED_EDGE('',*,*,#8416,.F.) ;
#12379=ORIENTED_EDGE('',*,*,#8786,.T.) ;
#12380=ORIENTED_EDGE('',*,*,#8177,.F.) ;
#12381=ORIENTED_EDGE('',*,*,#8791,.F.) ;
#12382=ORIENTED_EDGE('',*,*,#8792,.T.) ;
#12383=ORIENTED_EDGE('',*,*,#8787,.F.) ;
#12384=ORIENTED_EDGE('',*,*,#8792,.F.) ;
#12385=ORIENTED_EDGE('',*,*,#8790,.T.) ;
#12386=ORIENTED_EDGE('',*,*,#8793,.T.) ;
#12387=ORIENTED_EDGE('',*,*,#8788,.T.) ;
#12388=ORIENTED_EDGE('',*,*,#8793,.F.) ;
#12389=ORIENTED_EDGE('',*,*,#8789,.F.) ;
#12390=ORIENTED_EDGE('',*,*,#8182,.T.) ;
#12391=ORIENTED_EDGE('',*,*,#8367,.T.) ;
#12392=ORIENTED_EDGE('',*,*,#8794,.F.) ;
#12393=ORIENTED_EDGE('',*,*,#8795,.T.) ;
#12394=ORIENTED_EDGE('',*,*,#8796,.F.) ;
#12395=ORIENTED_EDGE('',*,*,#8797,.T.) ;
#12396=ORIENTED_EDGE('',*,*,#8798,.F.) ;
#12397=ORIENTED_EDGE('',*,*,#8799,.T.) ;
#12398=ORIENTED_EDGE('',*,*,#8417,.F.) ;
#12399=ORIENTED_EDGE('',*,*,#8794,.T.) ;
#12400=ORIENTED_EDGE('',*,*,#8184,.F.) ;
#12401=ORIENTED_EDGE('',*,*,#8799,.F.) ;
#12402=ORIENTED_EDGE('',*,*,#8800,.T.) ;
#12403=ORIENTED_EDGE('',*,*,#8795,.F.) ;
#12404=ORIENTED_EDGE('',*,*,#8800,.F.) ;
#12405=ORIENTED_EDGE('',*,*,#8798,.T.) ;
#12406=ORIENTED_EDGE('',*,*,#8801,.T.) ;
#12407=ORIENTED_EDGE('',*,*,#8796,.T.) ;
#12408=ORIENTED_EDGE('',*,*,#8801,.F.) ;
#12409=ORIENTED_EDGE('',*,*,#8797,.F.) ;
#12410=ORIENTED_EDGE('',*,*,#8175,.T.) ;
#12411=ORIENTED_EDGE('',*,*,#8369,.T.) ;
#12412=ORIENTED_EDGE('',*,*,#8802,.F.) ;
#12413=ORIENTED_EDGE('',*,*,#8803,.T.) ;
#12414=ORIENTED_EDGE('',*,*,#8804,.F.) ;
#12415=ORIENTED_EDGE('',*,*,#8805,.T.) ;
#12416=ORIENTED_EDGE('',*,*,#8806,.F.) ;
#12417=ORIENTED_EDGE('',*,*,#8807,.T.) ;
#12418=ORIENTED_EDGE('',*,*,#8415,.F.) ;
#12419=ORIENTED_EDGE('',*,*,#8802,.T.) ;
#12420=ORIENTED_EDGE('',*,*,#8180,.F.) ;
#12421=ORIENTED_EDGE('',*,*,#8807,.F.) ;
#12422=ORIENTED_EDGE('',*,*,#8808,.T.) ;
#12423=ORIENTED_EDGE('',*,*,#8803,.F.) ;
#12424=ORIENTED_EDGE('',*,*,#8808,.F.) ;
#12425=ORIENTED_EDGE('',*,*,#8806,.T.) ;
#12426=ORIENTED_EDGE('',*,*,#8809,.T.) ;
#12427=ORIENTED_EDGE('',*,*,#8804,.T.) ;
#12428=ORIENTED_EDGE('',*,*,#8809,.F.) ;
#12429=ORIENTED_EDGE('',*,*,#8805,.F.) ;
#12430=ORIENTED_EDGE('',*,*,#8174,.T.) ;
#12431=ORIENTED_EDGE('',*,*,#8370,.T.) ;
#12432=ORIENTED_EDGE('',*,*,#8810,.F.) ;
#12433=ORIENTED_EDGE('',*,*,#8811,.T.) ;
#12434=ORIENTED_EDGE('',*,*,#8812,.F.) ;
#12435=ORIENTED_EDGE('',*,*,#8813,.T.) ;
#12436=ORIENTED_EDGE('',*,*,#8814,.F.) ;
#12437=ORIENTED_EDGE('',*,*,#8815,.T.) ;
#12438=ORIENTED_EDGE('',*,*,#8414,.F.) ;
#12439=ORIENTED_EDGE('',*,*,#8810,.T.) ;
#12440=ORIENTED_EDGE('',*,*,#8172,.F.) ;
#12441=ORIENTED_EDGE('',*,*,#8815,.F.) ;
#12442=ORIENTED_EDGE('',*,*,#8816,.T.) ;
#12443=ORIENTED_EDGE('',*,*,#8811,.F.) ;
#12444=ORIENTED_EDGE('',*,*,#8816,.F.) ;
#12445=ORIENTED_EDGE('',*,*,#8814,.T.) ;
#12446=ORIENTED_EDGE('',*,*,#8817,.T.) ;
#12447=ORIENTED_EDGE('',*,*,#8812,.T.) ;
#12448=ORIENTED_EDGE('',*,*,#8817,.F.) ;
#12449=ORIENTED_EDGE('',*,*,#8813,.F.) ;
#12450=ORIENTED_EDGE('',*,*,#8170,.T.) ;
#12451=ORIENTED_EDGE('',*,*,#8371,.T.) ;
#12452=ORIENTED_EDGE('',*,*,#8818,.F.) ;
#12453=ORIENTED_EDGE('',*,*,#8819,.T.) ;
#12454=ORIENTED_EDGE('',*,*,#8820,.F.) ;
#12455=ORIENTED_EDGE('',*,*,#8821,.T.) ;
#12456=ORIENTED_EDGE('',*,*,#8822,.F.) ;
#12457=ORIENTED_EDGE('',*,*,#8823,.T.) ;
#12458=ORIENTED_EDGE('',*,*,#8413,.F.) ;
#12459=ORIENTED_EDGE('',*,*,#8818,.T.) ;
#12460=ORIENTED_EDGE('',*,*,#8168,.F.) ;
#12461=ORIENTED_EDGE('',*,*,#8823,.F.) ;
#12462=ORIENTED_EDGE('',*,*,#8824,.T.) ;
#12463=ORIENTED_EDGE('',*,*,#8819,.F.) ;
#12464=ORIENTED_EDGE('',*,*,#8824,.F.) ;
#12465=ORIENTED_EDGE('',*,*,#8822,.T.) ;
#12466=ORIENTED_EDGE('',*,*,#8825,.T.) ;
#12467=ORIENTED_EDGE('',*,*,#8820,.T.) ;
#12468=ORIENTED_EDGE('',*,*,#8825,.F.) ;
#12469=ORIENTED_EDGE('',*,*,#8821,.F.) ;
#12470=ORIENTED_EDGE('',*,*,#8166,.T.) ;
#12471=ORIENTED_EDGE('',*,*,#8372,.T.) ;
#12472=ORIENTED_EDGE('',*,*,#8826,.F.) ;
#12473=ORIENTED_EDGE('',*,*,#8827,.T.) ;
#12474=ORIENTED_EDGE('',*,*,#8828,.F.) ;
#12475=ORIENTED_EDGE('',*,*,#8829,.T.) ;
#12476=ORIENTED_EDGE('',*,*,#8830,.F.) ;
#12477=ORIENTED_EDGE('',*,*,#8831,.T.) ;
#12478=ORIENTED_EDGE('',*,*,#8412,.F.) ;
#12479=ORIENTED_EDGE('',*,*,#8826,.T.) ;
#12480=ORIENTED_EDGE('',*,*,#8164,.F.) ;
#12481=ORIENTED_EDGE('',*,*,#8831,.F.) ;
#12482=ORIENTED_EDGE('',*,*,#8832,.T.) ;
#12483=ORIENTED_EDGE('',*,*,#8827,.F.) ;
#12484=ORIENTED_EDGE('',*,*,#8832,.F.) ;
#12485=ORIENTED_EDGE('',*,*,#8830,.T.) ;
#12486=ORIENTED_EDGE('',*,*,#8833,.T.) ;
#12487=ORIENTED_EDGE('',*,*,#8828,.T.) ;
#12488=ORIENTED_EDGE('',*,*,#8833,.F.) ;
#12489=ORIENTED_EDGE('',*,*,#8829,.F.) ;
#12490=ORIENTED_EDGE('',*,*,#8162,.T.) ;
#12491=ORIENTED_EDGE('',*,*,#8373,.T.) ;
#12492=ORIENTED_EDGE('',*,*,#8834,.F.) ;
#12493=ORIENTED_EDGE('',*,*,#8835,.T.) ;
#12494=ORIENTED_EDGE('',*,*,#8836,.F.) ;
#12495=ORIENTED_EDGE('',*,*,#8837,.T.) ;
#12496=ORIENTED_EDGE('',*,*,#8838,.F.) ;
#12497=ORIENTED_EDGE('',*,*,#8839,.T.) ;
#12498=ORIENTED_EDGE('',*,*,#8411,.F.) ;
#12499=ORIENTED_EDGE('',*,*,#8834,.T.) ;
#12500=ORIENTED_EDGE('',*,*,#8160,.F.) ;
#12501=ORIENTED_EDGE('',*,*,#8839,.F.) ;
#12502=ORIENTED_EDGE('',*,*,#8840,.T.) ;
#12503=ORIENTED_EDGE('',*,*,#8835,.F.) ;
#12504=ORIENTED_EDGE('',*,*,#8840,.F.) ;
#12505=ORIENTED_EDGE('',*,*,#8838,.T.) ;
#12506=ORIENTED_EDGE('',*,*,#8841,.T.) ;
#12507=ORIENTED_EDGE('',*,*,#8836,.T.) ;
#12508=ORIENTED_EDGE('',*,*,#8841,.F.) ;
#12509=ORIENTED_EDGE('',*,*,#8837,.F.) ;
#12510=ORIENTED_EDGE('',*,*,#8158,.T.) ;
#12511=ORIENTED_EDGE('',*,*,#8374,.T.) ;
#12512=ORIENTED_EDGE('',*,*,#8842,.F.) ;
#12513=ORIENTED_EDGE('',*,*,#8843,.T.) ;
#12514=ORIENTED_EDGE('',*,*,#8844,.F.) ;
#12515=ORIENTED_EDGE('',*,*,#8845,.T.) ;
#12516=ORIENTED_EDGE('',*,*,#8846,.F.) ;
#12517=ORIENTED_EDGE('',*,*,#8847,.T.) ;
#12518=ORIENTED_EDGE('',*,*,#8410,.F.) ;
#12519=ORIENTED_EDGE('',*,*,#8842,.T.) ;
#12520=ORIENTED_EDGE('',*,*,#8156,.F.) ;
#12521=ORIENTED_EDGE('',*,*,#8847,.F.) ;
#12522=ORIENTED_EDGE('',*,*,#8848,.T.) ;
#12523=ORIENTED_EDGE('',*,*,#8843,.F.) ;
#12524=ORIENTED_EDGE('',*,*,#8848,.F.) ;
#12525=ORIENTED_EDGE('',*,*,#8846,.T.) ;
#12526=ORIENTED_EDGE('',*,*,#8849,.T.) ;
#12527=ORIENTED_EDGE('',*,*,#8844,.T.) ;
#12528=ORIENTED_EDGE('',*,*,#8849,.F.) ;
#12529=ORIENTED_EDGE('',*,*,#8845,.F.) ;
#12530=ORIENTED_EDGE('',*,*,#8154,.T.) ;
#12531=ORIENTED_EDGE('',*,*,#8375,.T.) ;
#12532=ORIENTED_EDGE('',*,*,#8850,.F.) ;
#12533=ORIENTED_EDGE('',*,*,#8851,.T.) ;
#12534=ORIENTED_EDGE('',*,*,#8852,.F.) ;
#12535=ORIENTED_EDGE('',*,*,#8853,.T.) ;
#12536=ORIENTED_EDGE('',*,*,#8854,.F.) ;
#12537=ORIENTED_EDGE('',*,*,#8855,.T.) ;
#12538=ORIENTED_EDGE('',*,*,#8409,.F.) ;
#12539=ORIENTED_EDGE('',*,*,#8469,.F.) ;
#12540=ORIENTED_EDGE('',*,*,#8850,.T.) ;
#12541=ORIENTED_EDGE('',*,*,#8152,.F.) ;
#12542=ORIENTED_EDGE('',*,*,#8855,.F.) ;
#12543=ORIENTED_EDGE('',*,*,#8856,.T.) ;
#12544=ORIENTED_EDGE('',*,*,#8851,.F.) ;
#12545=ORIENTED_EDGE('',*,*,#8856,.F.) ;
#12546=ORIENTED_EDGE('',*,*,#8854,.T.) ;
#12547=ORIENTED_EDGE('',*,*,#8857,.T.) ;
#12548=ORIENTED_EDGE('',*,*,#8852,.T.) ;
#12549=ORIENTED_EDGE('',*,*,#8857,.F.) ;
#12550=ORIENTED_EDGE('',*,*,#8853,.F.) ;
#12551=ORIENTED_EDGE('',*,*,#8150,.T.) ;
#12552=ORIENTED_EDGE('',*,*,#8376,.T.) ;
#12553=ORIENTED_EDGE('',*,*,#8858,.F.) ;
#12554=ORIENTED_EDGE('',*,*,#8859,.T.) ;
#12555=ORIENTED_EDGE('',*,*,#8860,.F.) ;
#12556=ORIENTED_EDGE('',*,*,#8861,.T.) ;
#12557=ORIENTED_EDGE('',*,*,#8862,.F.) ;
#12558=ORIENTED_EDGE('',*,*,#8863,.T.) ;
#12559=ORIENTED_EDGE('',*,*,#8468,.F.) ;
#12560=ORIENTED_EDGE('',*,*,#8858,.T.) ;
#12561=ORIENTED_EDGE('',*,*,#8148,.F.) ;
#12562=ORIENTED_EDGE('',*,*,#8863,.F.) ;
#12563=ORIENTED_EDGE('',*,*,#8864,.T.) ;
#12564=ORIENTED_EDGE('',*,*,#8859,.F.) ;
#12565=ORIENTED_EDGE('',*,*,#8864,.F.) ;
#12566=ORIENTED_EDGE('',*,*,#8862,.T.) ;
#12567=ORIENTED_EDGE('',*,*,#8865,.T.) ;
#12568=ORIENTED_EDGE('',*,*,#8860,.T.) ;
#12569=ORIENTED_EDGE('',*,*,#8865,.F.) ;
#12570=ORIENTED_EDGE('',*,*,#8861,.F.) ;
#12571=ORIENTED_EDGE('',*,*,#8146,.T.) ;
#12572=ORIENTED_EDGE('',*,*,#8377,.T.) ;
#12573=ORIENTED_EDGE('',*,*,#8866,.F.) ;
#12574=ORIENTED_EDGE('',*,*,#8867,.T.) ;
#12575=ORIENTED_EDGE('',*,*,#8868,.F.) ;
#12576=ORIENTED_EDGE('',*,*,#8869,.T.) ;
#12577=ORIENTED_EDGE('',*,*,#8870,.F.) ;
#12578=ORIENTED_EDGE('',*,*,#8871,.T.) ;
#12579=ORIENTED_EDGE('',*,*,#8467,.F.) ;
#12580=ORIENTED_EDGE('',*,*,#8866,.T.) ;
#12581=ORIENTED_EDGE('',*,*,#8144,.F.) ;
#12582=ORIENTED_EDGE('',*,*,#8871,.F.) ;
#12583=ORIENTED_EDGE('',*,*,#8872,.T.) ;
#12584=ORIENTED_EDGE('',*,*,#8867,.F.) ;
#12585=ORIENTED_EDGE('',*,*,#8872,.F.) ;
#12586=ORIENTED_EDGE('',*,*,#8870,.T.) ;
#12587=ORIENTED_EDGE('',*,*,#8873,.T.) ;
#12588=ORIENTED_EDGE('',*,*,#8868,.T.) ;
#12589=ORIENTED_EDGE('',*,*,#8873,.F.) ;
#12590=ORIENTED_EDGE('',*,*,#8869,.F.) ;
#12591=ORIENTED_EDGE('',*,*,#8142,.T.) ;
#12592=ORIENTED_EDGE('',*,*,#8378,.T.) ;
#12593=ORIENTED_EDGE('',*,*,#8874,.F.) ;
#12594=ORIENTED_EDGE('',*,*,#8875,.T.) ;
#12595=ORIENTED_EDGE('',*,*,#8876,.F.) ;
#12596=ORIENTED_EDGE('',*,*,#8877,.T.) ;
#12597=ORIENTED_EDGE('',*,*,#8878,.F.) ;
#12598=ORIENTED_EDGE('',*,*,#8879,.T.) ;
#12599=ORIENTED_EDGE('',*,*,#8466,.F.) ;
#12600=ORIENTED_EDGE('',*,*,#8874,.T.) ;
#12601=ORIENTED_EDGE('',*,*,#8140,.F.) ;
#12602=ORIENTED_EDGE('',*,*,#8879,.F.) ;
#12603=ORIENTED_EDGE('',*,*,#8880,.T.) ;
#12604=ORIENTED_EDGE('',*,*,#8875,.F.) ;
#12605=ORIENTED_EDGE('',*,*,#8880,.F.) ;
#12606=ORIENTED_EDGE('',*,*,#8878,.T.) ;
#12607=ORIENTED_EDGE('',*,*,#8881,.T.) ;
#12608=ORIENTED_EDGE('',*,*,#8876,.T.) ;
#12609=ORIENTED_EDGE('',*,*,#8881,.F.) ;
#12610=ORIENTED_EDGE('',*,*,#8877,.F.) ;
#12611=ORIENTED_EDGE('',*,*,#8138,.T.) ;
#12612=ORIENTED_EDGE('',*,*,#8379,.T.) ;
#12613=ORIENTED_EDGE('',*,*,#8882,.F.) ;
#12614=ORIENTED_EDGE('',*,*,#8883,.T.) ;
#12615=ORIENTED_EDGE('',*,*,#8884,.F.) ;
#12616=ORIENTED_EDGE('',*,*,#8885,.T.) ;
#12617=ORIENTED_EDGE('',*,*,#8886,.F.) ;
#12618=ORIENTED_EDGE('',*,*,#8887,.T.) ;
#12619=ORIENTED_EDGE('',*,*,#8465,.F.) ;
#12620=ORIENTED_EDGE('',*,*,#8882,.T.) ;
#12621=ORIENTED_EDGE('',*,*,#8136,.F.) ;
#12622=ORIENTED_EDGE('',*,*,#8887,.F.) ;
#12623=ORIENTED_EDGE('',*,*,#8888,.T.) ;
#12624=ORIENTED_EDGE('',*,*,#8883,.F.) ;
#12625=ORIENTED_EDGE('',*,*,#8888,.F.) ;
#12626=ORIENTED_EDGE('',*,*,#8886,.T.) ;
#12627=ORIENTED_EDGE('',*,*,#8889,.T.) ;
#12628=ORIENTED_EDGE('',*,*,#8884,.T.) ;
#12629=ORIENTED_EDGE('',*,*,#8889,.F.) ;
#12630=ORIENTED_EDGE('',*,*,#8885,.F.) ;
#12631=ORIENTED_EDGE('',*,*,#8134,.T.) ;
#12632=ORIENTED_EDGE('',*,*,#8380,.T.) ;
#12633=ORIENTED_EDGE('',*,*,#8890,.F.) ;
#12634=ORIENTED_EDGE('',*,*,#8891,.T.) ;
#12635=ORIENTED_EDGE('',*,*,#8892,.F.) ;
#12636=ORIENTED_EDGE('',*,*,#8893,.T.) ;
#12637=ORIENTED_EDGE('',*,*,#8894,.F.) ;
#12638=ORIENTED_EDGE('',*,*,#8895,.T.) ;
#12639=ORIENTED_EDGE('',*,*,#8464,.F.) ;
#12640=ORIENTED_EDGE('',*,*,#8890,.T.) ;
#12641=ORIENTED_EDGE('',*,*,#8132,.F.) ;
#12642=ORIENTED_EDGE('',*,*,#8895,.F.) ;
#12643=ORIENTED_EDGE('',*,*,#8896,.T.) ;
#12644=ORIENTED_EDGE('',*,*,#8891,.F.) ;
#12645=ORIENTED_EDGE('',*,*,#8896,.F.) ;
#12646=ORIENTED_EDGE('',*,*,#8894,.T.) ;
#12647=ORIENTED_EDGE('',*,*,#8897,.T.) ;
#12648=ORIENTED_EDGE('',*,*,#8892,.T.) ;
#12649=ORIENTED_EDGE('',*,*,#8897,.F.) ;
#12650=ORIENTED_EDGE('',*,*,#8893,.F.) ;
#12651=ORIENTED_EDGE('',*,*,#8130,.T.) ;
#12652=ORIENTED_EDGE('',*,*,#8384,.T.) ;
#12653=ORIENTED_EDGE('',*,*,#8898,.F.) ;
#12654=ORIENTED_EDGE('',*,*,#8899,.T.) ;
#12655=ORIENTED_EDGE('',*,*,#8900,.F.) ;
#12656=ORIENTED_EDGE('',*,*,#8901,.T.) ;
#12657=ORIENTED_EDGE('',*,*,#8902,.F.) ;
#12658=ORIENTED_EDGE('',*,*,#8903,.T.) ;
#12659=ORIENTED_EDGE('',*,*,#8460,.F.) ;
#12660=ORIENTED_EDGE('',*,*,#8898,.T.) ;
#12661=ORIENTED_EDGE('',*,*,#8121,.F.) ;
#12662=ORIENTED_EDGE('',*,*,#8903,.F.) ;
#12663=ORIENTED_EDGE('',*,*,#8904,.T.) ;
#12664=ORIENTED_EDGE('',*,*,#8899,.F.) ;
#12665=ORIENTED_EDGE('',*,*,#8904,.F.) ;
#12666=ORIENTED_EDGE('',*,*,#8902,.T.) ;
#12667=ORIENTED_EDGE('',*,*,#8905,.T.) ;
#12668=ORIENTED_EDGE('',*,*,#8900,.T.) ;
#12669=ORIENTED_EDGE('',*,*,#8905,.F.) ;
#12670=ORIENTED_EDGE('',*,*,#8901,.F.) ;
#12671=ORIENTED_EDGE('',*,*,#8126,.T.) ;
#12672=ORIENTED_EDGE('',*,*,#8383,.T.) ;
#12673=ORIENTED_EDGE('',*,*,#8906,.F.) ;
#12674=ORIENTED_EDGE('',*,*,#8907,.T.) ;
#12675=ORIENTED_EDGE('',*,*,#8908,.F.) ;
#12676=ORIENTED_EDGE('',*,*,#8909,.T.) ;
#12677=ORIENTED_EDGE('',*,*,#8910,.F.) ;
#12678=ORIENTED_EDGE('',*,*,#8911,.T.) ;
#12679=ORIENTED_EDGE('',*,*,#8461,.F.) ;
#12680=ORIENTED_EDGE('',*,*,#8906,.T.) ;
#12681=ORIENTED_EDGE('',*,*,#8117,.F.) ;
#12682=ORIENTED_EDGE('',*,*,#8911,.F.) ;
#12683=ORIENTED_EDGE('',*,*,#8912,.T.) ;
#12684=ORIENTED_EDGE('',*,*,#8907,.F.) ;
#12685=ORIENTED_EDGE('',*,*,#8912,.F.) ;
#12686=ORIENTED_EDGE('',*,*,#8910,.T.) ;
#12687=ORIENTED_EDGE('',*,*,#8913,.T.) ;
#12688=ORIENTED_EDGE('',*,*,#8908,.T.) ;
#12689=ORIENTED_EDGE('',*,*,#8913,.F.) ;
#12690=ORIENTED_EDGE('',*,*,#8909,.F.) ;
#12691=ORIENTED_EDGE('',*,*,#8119,.T.) ;
#12692=ORIENTED_EDGE('',*,*,#8382,.T.) ;
#12693=ORIENTED_EDGE('',*,*,#8914,.F.) ;
#12694=ORIENTED_EDGE('',*,*,#8915,.T.) ;
#12695=ORIENTED_EDGE('',*,*,#8916,.F.) ;
#12696=ORIENTED_EDGE('',*,*,#8917,.T.) ;
#12697=ORIENTED_EDGE('',*,*,#8918,.F.) ;
#12698=ORIENTED_EDGE('',*,*,#8919,.T.) ;
#12699=ORIENTED_EDGE('',*,*,#8462,.F.) ;
#12700=ORIENTED_EDGE('',*,*,#8914,.T.) ;
#12701=ORIENTED_EDGE('',*,*,#8113,.F.) ;
#12702=ORIENTED_EDGE('',*,*,#8919,.F.) ;
#12703=ORIENTED_EDGE('',*,*,#8920,.T.) ;
#12704=ORIENTED_EDGE('',*,*,#8915,.F.) ;
#12705=ORIENTED_EDGE('',*,*,#8920,.F.) ;
#12706=ORIENTED_EDGE('',*,*,#8918,.T.) ;
#12707=ORIENTED_EDGE('',*,*,#8921,.T.) ;
#12708=ORIENTED_EDGE('',*,*,#8916,.T.) ;
#12709=ORIENTED_EDGE('',*,*,#8921,.F.) ;
#12710=ORIENTED_EDGE('',*,*,#8917,.F.) ;
#12711=ORIENTED_EDGE('',*,*,#8115,.T.) ;
#12712=ORIENTED_EDGE('',*,*,#8381,.T.) ;
#12713=ORIENTED_EDGE('',*,*,#8922,.F.) ;
#12714=ORIENTED_EDGE('',*,*,#8923,.T.) ;
#12715=ORIENTED_EDGE('',*,*,#8924,.F.) ;
#12716=ORIENTED_EDGE('',*,*,#8925,.T.) ;
#12717=ORIENTED_EDGE('',*,*,#8926,.F.) ;
#12718=ORIENTED_EDGE('',*,*,#8927,.T.) ;
#12719=ORIENTED_EDGE('',*,*,#8463,.F.) ;
#12720=ORIENTED_EDGE('',*,*,#8922,.T.) ;
#12721=ORIENTED_EDGE('',*,*,#8128,.F.) ;
#12722=ORIENTED_EDGE('',*,*,#8927,.F.) ;
#12723=ORIENTED_EDGE('',*,*,#8928,.T.) ;
#12724=ORIENTED_EDGE('',*,*,#8923,.F.) ;
#12725=ORIENTED_EDGE('',*,*,#8928,.F.) ;
#12726=ORIENTED_EDGE('',*,*,#8926,.T.) ;
#12727=ORIENTED_EDGE('',*,*,#8929,.T.) ;
#12728=ORIENTED_EDGE('',*,*,#8924,.T.) ;
#12729=ORIENTED_EDGE('',*,*,#8929,.F.) ;
#12730=ORIENTED_EDGE('',*,*,#8925,.F.) ;
#12731=ORIENTED_EDGE('',*,*,#8111,.T.) ;
#12732=ORIENTED_EDGE('',*,*,#8385,.T.) ;
#12733=ORIENTED_EDGE('',*,*,#8930,.F.) ;
#12734=ORIENTED_EDGE('',*,*,#8931,.T.) ;
#12735=ORIENTED_EDGE('',*,*,#8932,.F.) ;
#12736=ORIENTED_EDGE('',*,*,#8933,.T.) ;
#12737=ORIENTED_EDGE('',*,*,#8934,.F.) ;
#12738=ORIENTED_EDGE('',*,*,#8935,.T.) ;
#12739=ORIENTED_EDGE('',*,*,#8459,.F.) ;
#12740=ORIENTED_EDGE('',*,*,#8930,.T.) ;
#12741=ORIENTED_EDGE('',*,*,#8124,.F.) ;
#12742=ORIENTED_EDGE('',*,*,#8935,.F.) ;
#12743=ORIENTED_EDGE('',*,*,#8936,.T.) ;
#12744=ORIENTED_EDGE('',*,*,#8931,.F.) ;
#12745=ORIENTED_EDGE('',*,*,#8936,.F.) ;
#12746=ORIENTED_EDGE('',*,*,#8934,.T.) ;
#12747=ORIENTED_EDGE('',*,*,#8937,.T.) ;
#12748=ORIENTED_EDGE('',*,*,#8932,.T.) ;
#12749=ORIENTED_EDGE('',*,*,#8937,.F.) ;
#12750=ORIENTED_EDGE('',*,*,#8933,.F.) ;
#12751=ORIENTED_EDGE('',*,*,#8110,.T.) ;
#12752=ORIENTED_EDGE('',*,*,#8386,.T.) ;
#12753=ORIENTED_EDGE('',*,*,#8938,.F.) ;
#12754=ORIENTED_EDGE('',*,*,#8939,.T.) ;
#12755=ORIENTED_EDGE('',*,*,#8940,.F.) ;
#12756=ORIENTED_EDGE('',*,*,#8941,.T.) ;
#12757=ORIENTED_EDGE('',*,*,#8942,.F.) ;
#12758=ORIENTED_EDGE('',*,*,#8943,.T.) ;
#12759=ORIENTED_EDGE('',*,*,#8458,.F.) ;
#12760=ORIENTED_EDGE('',*,*,#8938,.T.) ;
#12761=ORIENTED_EDGE('',*,*,#8108,.F.) ;
#12762=ORIENTED_EDGE('',*,*,#8943,.F.) ;
#12763=ORIENTED_EDGE('',*,*,#8944,.T.) ;
#12764=ORIENTED_EDGE('',*,*,#8939,.F.) ;
#12765=ORIENTED_EDGE('',*,*,#8944,.F.) ;
#12766=ORIENTED_EDGE('',*,*,#8942,.T.) ;
#12767=ORIENTED_EDGE('',*,*,#8945,.T.) ;
#12768=ORIENTED_EDGE('',*,*,#8940,.T.) ;
#12769=ORIENTED_EDGE('',*,*,#8945,.F.) ;
#12770=ORIENTED_EDGE('',*,*,#8941,.F.) ;
#12771=ORIENTED_EDGE('',*,*,#8106,.T.) ;
#12772=ORIENTED_EDGE('',*,*,#8387,.T.) ;
#12773=ORIENTED_EDGE('',*,*,#8946,.F.) ;
#12774=ORIENTED_EDGE('',*,*,#8947,.T.) ;
#12775=ORIENTED_EDGE('',*,*,#8948,.F.) ;
#12776=ORIENTED_EDGE('',*,*,#8949,.T.) ;
#12777=ORIENTED_EDGE('',*,*,#8950,.F.) ;
#12778=ORIENTED_EDGE('',*,*,#8951,.T.) ;
#12779=ORIENTED_EDGE('',*,*,#8457,.F.) ;
#12780=ORIENTED_EDGE('',*,*,#8946,.T.) ;
#12781=ORIENTED_EDGE('',*,*,#8104,.F.) ;
#12782=ORIENTED_EDGE('',*,*,#8951,.F.) ;
#12783=ORIENTED_EDGE('',*,*,#8952,.T.) ;
#12784=ORIENTED_EDGE('',*,*,#8947,.F.) ;
#12785=ORIENTED_EDGE('',*,*,#8952,.F.) ;
#12786=ORIENTED_EDGE('',*,*,#8950,.T.) ;
#12787=ORIENTED_EDGE('',*,*,#8953,.T.) ;
#12788=ORIENTED_EDGE('',*,*,#8948,.T.) ;
#12789=ORIENTED_EDGE('',*,*,#8953,.F.) ;
#12790=ORIENTED_EDGE('',*,*,#8949,.F.) ;
#12791=ORIENTED_EDGE('',*,*,#8102,.T.) ;
#12792=ORIENTED_EDGE('',*,*,#8388,.T.) ;
#12793=ORIENTED_EDGE('',*,*,#8954,.F.) ;
#12794=ORIENTED_EDGE('',*,*,#8955,.T.) ;
#12795=ORIENTED_EDGE('',*,*,#8956,.F.) ;
#12796=ORIENTED_EDGE('',*,*,#8957,.T.) ;
#12797=ORIENTED_EDGE('',*,*,#8958,.F.) ;
#12798=ORIENTED_EDGE('',*,*,#8959,.T.) ;
#12799=ORIENTED_EDGE('',*,*,#8456,.F.) ;
#12800=ORIENTED_EDGE('',*,*,#8954,.T.) ;
#12801=ORIENTED_EDGE('',*,*,#8100,.F.) ;
#12802=ORIENTED_EDGE('',*,*,#8959,.F.) ;
#12803=ORIENTED_EDGE('',*,*,#8960,.T.) ;
#12804=ORIENTED_EDGE('',*,*,#8955,.F.) ;
#12805=ORIENTED_EDGE('',*,*,#8960,.F.) ;
#12806=ORIENTED_EDGE('',*,*,#8958,.T.) ;
#12807=ORIENTED_EDGE('',*,*,#8961,.T.) ;
#12808=ORIENTED_EDGE('',*,*,#8956,.T.) ;
#12809=ORIENTED_EDGE('',*,*,#8961,.F.) ;
#12810=ORIENTED_EDGE('',*,*,#8957,.F.) ;
#12811=ORIENTED_EDGE('',*,*,#8095,.T.) ;
#12812=ORIENTED_EDGE('',*,*,#8090,.T.) ;
#12813=ORIENTED_EDGE('',*,*,#8094,.F.) ;
#12814=ORIENTED_EDGE('',*,*,#8083,.T.) ;
#12815=ORIENTED_EDGE('',*,*,#8481,.T.) ;
#14553=CONICAL_SURFACE('',#16399,47.0433475024125,1.30899693899575) ;
#14554=CONICAL_SURFACE('',#16402,49.2411809548974,0.261799387799187) ;
#14555=CONICAL_SURFACE('',#16405,49.5,1.30899693899575) ;
#14556=CONICAL_SURFACE('',#16467,47.175,1.30899693899575) ;
#14557=CONICAL_SURFACE('',#16531,49.5,0.261799387799147) ;
#14558=CONICAL_SURFACE('',#16534,49.2411809548975,1.30899693899575) ;
#14921=ADVANCED_FACE('',(#1833),#908,.F.) ;
#14922=ADVANCED_FACE('',(#1834),#909,.F.) ;
#14923=ADVANCED_FACE('',(#1835),#910,.F.) ;
#14924=ADVANCED_FACE('',(#1836,#750),#911,.F.) ;
#14925=ADVANCED_FACE('',(#1837),#1264,.T.) ;
#14926=ADVANCED_FACE('',(#1838),#1265,.T.) ;
#14927=ADVANCED_FACE('',(#1839),#1266,.T.) ;
#14928=ADVANCED_FACE('',(#1840),#1267,.T.) ;
#14929=ADVANCED_FACE('',(#1841),#1268,.T.) ;
#14930=ADVANCED_FACE('',(#1842),#1269,.T.) ;
#14931=ADVANCED_FACE('',(#1843),#1270,.T.) ;
#14932=ADVANCED_FACE('',(#1844),#1271,.T.) ;
#14933=ADVANCED_FACE('',(#1845),#1272,.T.) ;
#14934=ADVANCED_FACE('',(#1846),#1273,.T.) ;
#14935=ADVANCED_FACE('',(#1847),#1274,.T.) ;
#14936=ADVANCED_FACE('',(#1848),#1275,.T.) ;
#14937=ADVANCED_FACE('',(#1849),#1276,.T.) ;
#14938=ADVANCED_FACE('',(#1850),#1277,.T.) ;
#14939=ADVANCED_FACE('',(#1851),#1278,.T.) ;
#14940=ADVANCED_FACE('',(#1852),#1279,.T.) ;
#14941=ADVANCED_FACE('',(#1853),#1280,.T.) ;
#14942=ADVANCED_FACE('',(#1854),#1281,.T.) ;
#14943=ADVANCED_FACE('',(#1855),#1282,.T.) ;
#14944=ADVANCED_FACE('',(#1856),#1283,.T.) ;
#14945=ADVANCED_FACE('',(#1857),#1284,.T.) ;
#14946=ADVANCED_FACE('',(#1858),#1285,.T.) ;
#14947=ADVANCED_FACE('',(#1859),#1286,.T.) ;
#14948=ADVANCED_FACE('',(#1860),#1287,.T.) ;
#14949=ADVANCED_FACE('',(#1861),#1288,.T.) ;
#14950=ADVANCED_FACE('',(#1862),#1289,.T.) ;
#14951=ADVANCED_FACE('',(#1863),#1290,.T.) ;
#14952=ADVANCED_FACE('',(#1864),#1291,.T.) ;
#14953=ADVANCED_FACE('',(#1865),#1292,.T.) ;
#14954=ADVANCED_FACE('',(#1866),#1293,.T.) ;
#14955=ADVANCED_FACE('',(#1867),#1294,.T.) ;
#14956=ADVANCED_FACE('',(#1868),#1295,.T.) ;
#14957=ADVANCED_FACE('',(#1869),#1296,.T.) ;
#14958=ADVANCED_FACE('',(#1870),#1297,.T.) ;
#14959=ADVANCED_FACE('',(#1871),#1298,.T.) ;
#14960=ADVANCED_FACE('',(#1872),#1299,.T.) ;
#14961=ADVANCED_FACE('',(#1873),#1300,.T.) ;
#14962=ADVANCED_FACE('',(#1874),#1301,.T.) ;
#14963=ADVANCED_FACE('',(#1875),#1302,.T.) ;
#14964=ADVANCED_FACE('',(#1876),#1303,.T.) ;
#14965=ADVANCED_FACE('',(#1877),#1304,.T.) ;
#14966=ADVANCED_FACE('',(#1878),#1305,.T.) ;
#14967=ADVANCED_FACE('',(#1879),#1306,.T.) ;
#14968=ADVANCED_FACE('',(#1880),#1307,.T.) ;
#14969=ADVANCED_FACE('',(#1881),#1308,.T.) ;
#14970=ADVANCED_FACE('',(#1882),#1309,.T.) ;
#14971=ADVANCED_FACE('',(#1883),#1310,.T.) ;
#14972=ADVANCED_FACE('',(#1884),#1311,.T.) ;
#14973=ADVANCED_FACE('',(#1885),#1312,.T.) ;
#14974=ADVANCED_FACE('',(#1886),#1313,.T.) ;
#14975=ADVANCED_FACE('',(#1887),#1314,.T.) ;
#14976=ADVANCED_FACE('',(#1888),#1315,.T.) ;
#14977=ADVANCED_FACE('',(#1889),#1316,.T.) ;
#14978=ADVANCED_FACE('',(#1890),#1317,.T.) ;
#14979=ADVANCED_FACE('',(#1891),#1318,.T.) ;
#14980=ADVANCED_FACE('',(#1892),#1319,.T.) ;
#14981=ADVANCED_FACE('',(#1893),#1320,.T.) ;
#14982=ADVANCED_FACE('',(#1894),#1321,.T.) ;
#14983=ADVANCED_FACE('',(#1895),#1322,.T.) ;
#14984=ADVANCED_FACE('',(#1896),#1323,.T.) ;
#14985=ADVANCED_FACE('',(#1897),#1324,.T.) ;
#14986=ADVANCED_FACE('',(#1898,#751),#912,.F.) ;
#14987=ADVANCED_FACE('',(#1899),#14553,.F.) ;
#14988=ADVANCED_FACE('',(#1900),#14554,.T.) ;
#14989=ADVANCED_FACE('',(#1901),#14555,.T.) ;
#14990=ADVANCED_FACE('',(#1902),#14556,.T.) ;
#14991=ADVANCED_FACE('',(#1903),#14557,.T.) ;
#14992=ADVANCED_FACE('',(#1904),#14558,.F.) ;
#14993=ADVANCED_FACE('',(#1905,#752),#913,.F.) ;
#14994=ADVANCED_FACE('',(#1906),#1325,.T.) ;
#14995=ADVANCED_FACE('',(#1907,#753),#914,.F.) ;
#14996=ADVANCED_FACE('',(#1908),#1326,.T.) ;
#14997=ADVANCED_FACE('',(#1909,#754),#915,.F.) ;
#14998=ADVANCED_FACE('',(#1910),#916,.T.) ;
#14999=ADVANCED_FACE('',(#1911),#917,.F.) ;
#15000=ADVANCED_FACE('',(#1912),#1327,.T.) ;
#15001=ADVANCED_FACE('',(#1913),#1328,.F.) ;
#15002=ADVANCED_FACE('',(#1914),#1329,.T.) ;
#15003=ADVANCED_FACE('',(#1915),#918,.T.) ;
#15004=ADVANCED_FACE('',(#1916),#919,.F.) ;
#15005=ADVANCED_FACE('',(#1917),#1330,.T.) ;
#15006=ADVANCED_FACE('',(#1918),#1331,.F.) ;
#15007=ADVANCED_FACE('',(#1919),#1332,.T.) ;
#15008=ADVANCED_FACE('',(#1920),#920,.T.) ;
#15009=ADVANCED_FACE('',(#1921),#921,.F.) ;
#15010=ADVANCED_FACE('',(#1922),#1333,.T.) ;
#15011=ADVANCED_FACE('',(#1923),#1334,.F.) ;
#15012=ADVANCED_FACE('',(#1924),#1335,.T.) ;
#15013=ADVANCED_FACE('',(#1925),#922,.T.) ;
#15014=ADVANCED_FACE('',(#1926),#923,.F.) ;
#15015=ADVANCED_FACE('',(#1927),#1336,.T.) ;
#15016=ADVANCED_FACE('',(#1928),#1337,.F.) ;
#15017=ADVANCED_FACE('',(#1929),#1338,.T.) ;
#15018=ADVANCED_FACE('',(#1930),#924,.T.) ;
#15019=ADVANCED_FACE('',(#1931),#925,.F.) ;
#15020=ADVANCED_FACE('',(#1932),#1339,.T.) ;
#15021=ADVANCED_FACE('',(#1933),#1340,.F.) ;
#15022=ADVANCED_FACE('',(#1934),#1341,.T.) ;
#15023=ADVANCED_FACE('',(#1935),#926,.T.) ;
#15024=ADVANCED_FACE('',(#1936),#927,.F.) ;
#15025=ADVANCED_FACE('',(#1937),#1342,.T.) ;
#15026=ADVANCED_FACE('',(#1938),#1343,.F.) ;
#15027=ADVANCED_FACE('',(#1939),#1344,.T.) ;
#15028=ADVANCED_FACE('',(#1940),#928,.T.) ;
#15029=ADVANCED_FACE('',(#1941),#929,.F.) ;
#15030=ADVANCED_FACE('',(#1942),#1345,.T.) ;
#15031=ADVANCED_FACE('',(#1943),#1346,.F.) ;
#15032=ADVANCED_FACE('',(#1944),#1347,.T.) ;
#15033=ADVANCED_FACE('',(#1945),#930,.T.) ;
#15034=ADVANCED_FACE('',(#1946),#931,.F.) ;
#15035=ADVANCED_FACE('',(#1947),#1348,.T.) ;
#15036=ADVANCED_FACE('',(#1948),#1349,.F.) ;
#15037=ADVANCED_FACE('',(#1949),#1350,.T.) ;
#15038=ADVANCED_FACE('',(#1950),#932,.T.) ;
#15039=ADVANCED_FACE('',(#1951),#933,.F.) ;
#15040=ADVANCED_FACE('',(#1952),#1351,.T.) ;
#15041=ADVANCED_FACE('',(#1953),#1352,.F.) ;
#15042=ADVANCED_FACE('',(#1954),#1353,.T.) ;
#15043=ADVANCED_FACE('',(#1955),#934,.T.) ;
#15044=ADVANCED_FACE('',(#1956),#935,.F.) ;
#15045=ADVANCED_FACE('',(#1957),#1354,.T.) ;
#15046=ADVANCED_FACE('',(#1958),#1355,.F.) ;
#15047=ADVANCED_FACE('',(#1959),#1356,.T.) ;
#15048=ADVANCED_FACE('',(#1960),#936,.T.) ;
#15049=ADVANCED_FACE('',(#1961),#937,.F.) ;
#15050=ADVANCED_FACE('',(#1962),#1357,.T.) ;
#15051=ADVANCED_FACE('',(#1963),#1358,.F.) ;
#15052=ADVANCED_FACE('',(#1964),#1359,.T.) ;
#15053=ADVANCED_FACE('',(#1965),#938,.T.) ;
#15054=ADVANCED_FACE('',(#1966),#939,.F.) ;
#15055=ADVANCED_FACE('',(#1967),#1360,.T.) ;
#15056=ADVANCED_FACE('',(#1968),#1361,.F.) ;
#15057=ADVANCED_FACE('',(#1969),#1362,.T.) ;
#15058=ADVANCED_FACE('',(#1970),#940,.T.) ;
#15059=ADVANCED_FACE('',(#1971),#941,.F.) ;
#15060=ADVANCED_FACE('',(#1972),#1363,.T.) ;
#15061=ADVANCED_FACE('',(#1973),#1364,.F.) ;
#15062=ADVANCED_FACE('',(#1974),#1365,.T.) ;
#15063=ADVANCED_FACE('',(#1975),#942,.T.) ;
#15064=ADVANCED_FACE('',(#1976),#943,.F.) ;
#15065=ADVANCED_FACE('',(#1977),#1366,.T.) ;
#15066=ADVANCED_FACE('',(#1978),#1367,.F.) ;
#15067=ADVANCED_FACE('',(#1979),#1368,.T.) ;
#15068=ADVANCED_FACE('',(#1980),#944,.T.) ;
#15069=ADVANCED_FACE('',(#1981),#945,.F.) ;
#15070=ADVANCED_FACE('',(#1982),#1369,.T.) ;
#15071=ADVANCED_FACE('',(#1983),#1370,.F.) ;
#15072=ADVANCED_FACE('',(#1984),#1371,.T.) ;
#15073=ADVANCED_FACE('',(#1985),#946,.T.) ;
#15074=ADVANCED_FACE('',(#1986),#947,.F.) ;
#15075=ADVANCED_FACE('',(#1987),#1372,.T.) ;
#15076=ADVANCED_FACE('',(#1988),#1373,.F.) ;
#15077=ADVANCED_FACE('',(#1989),#1374,.T.) ;
#15078=ADVANCED_FACE('',(#1990),#948,.T.) ;
#15079=ADVANCED_FACE('',(#1991),#949,.F.) ;
#15080=ADVANCED_FACE('',(#1992),#1375,.T.) ;
#15081=ADVANCED_FACE('',(#1993),#1376,.F.) ;
#15082=ADVANCED_FACE('',(#1994),#1377,.T.) ;
#15083=ADVANCED_FACE('',(#1995),#950,.T.) ;
#15084=ADVANCED_FACE('',(#1996),#951,.F.) ;
#15085=ADVANCED_FACE('',(#1997),#1378,.T.) ;
#15086=ADVANCED_FACE('',(#1998),#1379,.F.) ;
#15087=ADVANCED_FACE('',(#1999),#1380,.T.) ;
#15088=ADVANCED_FACE('',(#2000),#952,.T.) ;
#15089=ADVANCED_FACE('',(#2001),#953,.F.) ;
#15090=ADVANCED_FACE('',(#2002),#1381,.T.) ;
#15091=ADVANCED_FACE('',(#2003),#1382,.F.) ;
#15092=ADVANCED_FACE('',(#2004),#1383,.T.) ;
#15093=ADVANCED_FACE('',(#2005),#954,.T.) ;
#15094=ADVANCED_FACE('',(#2006),#955,.F.) ;
#15095=ADVANCED_FACE('',(#2007),#1384,.T.) ;
#15096=ADVANCED_FACE('',(#2008),#1385,.F.) ;
#15097=ADVANCED_FACE('',(#2009),#1386,.T.) ;
#15098=ADVANCED_FACE('',(#2010),#956,.T.) ;
#15099=ADVANCED_FACE('',(#2011),#957,.F.) ;
#15100=ADVANCED_FACE('',(#2012),#1387,.T.) ;
#15101=ADVANCED_FACE('',(#2013),#1388,.F.) ;
#15102=ADVANCED_FACE('',(#2014),#1389,.T.) ;
#15103=ADVANCED_FACE('',(#2015),#958,.T.) ;
#15104=ADVANCED_FACE('',(#2016),#959,.F.) ;
#15105=ADVANCED_FACE('',(#2017),#1390,.T.) ;
#15106=ADVANCED_FACE('',(#2018),#1391,.F.) ;
#15107=ADVANCED_FACE('',(#2019),#1392,.T.) ;
#15108=ADVANCED_FACE('',(#2020),#960,.T.) ;
#15109=ADVANCED_FACE('',(#2021),#961,.F.) ;
#15110=ADVANCED_FACE('',(#2022),#1393,.T.) ;
#15111=ADVANCED_FACE('',(#2023),#1394,.F.) ;
#15112=ADVANCED_FACE('',(#2024),#1395,.T.) ;
#15113=ADVANCED_FACE('',(#2025),#962,.T.) ;
#15114=ADVANCED_FACE('',(#2026),#963,.F.) ;
#15115=ADVANCED_FACE('',(#2027),#1396,.T.) ;
#15116=ADVANCED_FACE('',(#2028),#1397,.F.) ;
#15117=ADVANCED_FACE('',(#2029),#1398,.T.) ;
#15118=ADVANCED_FACE('',(#2030),#964,.T.) ;
#15119=ADVANCED_FACE('',(#2031),#965,.F.) ;
#15120=ADVANCED_FACE('',(#2032),#1399,.T.) ;
#15121=ADVANCED_FACE('',(#2033),#1400,.F.) ;
#15122=ADVANCED_FACE('',(#2034),#1401,.T.) ;
#15123=ADVANCED_FACE('',(#2035),#966,.T.) ;
#15124=ADVANCED_FACE('',(#2036),#967,.F.) ;
#15125=ADVANCED_FACE('',(#2037),#1402,.T.) ;
#15126=ADVANCED_FACE('',(#2038),#1403,.F.) ;
#15127=ADVANCED_FACE('',(#2039),#1404,.T.) ;
#15128=ADVANCED_FACE('',(#2040),#968,.T.) ;
#15129=ADVANCED_FACE('',(#2041),#969,.F.) ;
#15130=ADVANCED_FACE('',(#2042),#1405,.T.) ;
#15131=ADVANCED_FACE('',(#2043),#1406,.F.) ;
#15132=ADVANCED_FACE('',(#2044),#1407,.T.) ;
#15133=ADVANCED_FACE('',(#2045),#970,.T.) ;
#15134=ADVANCED_FACE('',(#2046),#971,.F.) ;
#15135=ADVANCED_FACE('',(#2047),#1408,.T.) ;
#15136=ADVANCED_FACE('',(#2048),#1409,.F.) ;
#15137=ADVANCED_FACE('',(#2049),#1410,.T.) ;
#15138=ADVANCED_FACE('',(#2050),#972,.T.) ;
#15139=ADVANCED_FACE('',(#2051),#973,.F.) ;
#15140=ADVANCED_FACE('',(#2052),#1411,.T.) ;
#15141=ADVANCED_FACE('',(#2053),#1412,.F.) ;
#15142=ADVANCED_FACE('',(#2054),#1413,.T.) ;
#15143=ADVANCED_FACE('',(#2055),#974,.T.) ;
#15144=ADVANCED_FACE('',(#2056),#975,.F.) ;
#15145=ADVANCED_FACE('',(#2057),#1414,.T.) ;
#15146=ADVANCED_FACE('',(#2058),#1415,.F.) ;
#15147=ADVANCED_FACE('',(#2059),#1416,.T.) ;
#15148=ADVANCED_FACE('',(#2060),#976,.T.) ;
#15149=ADVANCED_FACE('',(#2061),#977,.F.) ;
#15150=ADVANCED_FACE('',(#2062),#1417,.T.) ;
#15151=ADVANCED_FACE('',(#2063),#1418,.F.) ;
#15152=ADVANCED_FACE('',(#2064),#1419,.T.) ;
#15153=ADVANCED_FACE('',(#2065),#978,.T.) ;
#15154=ADVANCED_FACE('',(#2066),#979,.F.) ;
#15155=ADVANCED_FACE('',(#2067),#1420,.T.) ;
#15156=ADVANCED_FACE('',(#2068),#1421,.F.) ;
#15157=ADVANCED_FACE('',(#2069),#1422,.T.) ;
#15158=ADVANCED_FACE('',(#2070),#980,.T.) ;
#15159=ADVANCED_FACE('',(#2071),#981,.F.) ;
#15160=ADVANCED_FACE('',(#2072),#1423,.T.) ;
#15161=ADVANCED_FACE('',(#2073),#1424,.F.) ;
#15162=ADVANCED_FACE('',(#2074),#1425,.T.) ;
#15163=ADVANCED_FACE('',(#2075),#982,.T.) ;
#15164=ADVANCED_FACE('',(#2076),#983,.F.) ;
#15165=ADVANCED_FACE('',(#2077),#1426,.T.) ;
#15166=ADVANCED_FACE('',(#2078),#1427,.F.) ;
#15167=ADVANCED_FACE('',(#2079),#1428,.T.) ;
#15168=ADVANCED_FACE('',(#2080),#984,.T.) ;
#15169=ADVANCED_FACE('',(#2081),#985,.F.) ;
#15170=ADVANCED_FACE('',(#2082),#1429,.T.) ;
#15171=ADVANCED_FACE('',(#2083),#1430,.F.) ;
#15172=ADVANCED_FACE('',(#2084),#1431,.T.) ;
#15173=ADVANCED_FACE('',(#2085),#986,.T.) ;
#15174=ADVANCED_FACE('',(#2086),#987,.F.) ;
#15175=ADVANCED_FACE('',(#2087),#1432,.T.) ;
#15176=ADVANCED_FACE('',(#2088),#1433,.F.) ;
#15177=ADVANCED_FACE('',(#2089),#1434,.T.) ;
#15178=ADVANCED_FACE('',(#2090),#988,.T.) ;
#15179=ADVANCED_FACE('',(#2091),#989,.F.) ;
#15180=ADVANCED_FACE('',(#2092),#1435,.T.) ;
#15181=ADVANCED_FACE('',(#2093),#1436,.F.) ;
#15182=ADVANCED_FACE('',(#2094),#1437,.T.) ;
#15183=ADVANCED_FACE('',(#2095),#990,.T.) ;
#15184=ADVANCED_FACE('',(#2096),#991,.F.) ;
#15185=ADVANCED_FACE('',(#2097),#1438,.T.) ;
#15186=ADVANCED_FACE('',(#2098),#1439,.F.) ;
#15187=ADVANCED_FACE('',(#2099),#1440,.T.) ;
#15188=ADVANCED_FACE('',(#2100),#992,.T.) ;
#15189=ADVANCED_FACE('',(#2101),#993,.F.) ;
#15190=ADVANCED_FACE('',(#2102),#1441,.T.) ;
#15191=ADVANCED_FACE('',(#2103),#1442,.F.) ;
#15192=ADVANCED_FACE('',(#2104),#1443,.T.) ;
#15193=ADVANCED_FACE('',(#2105),#994,.T.) ;
#15194=ADVANCED_FACE('',(#2106),#995,.F.) ;
#15195=ADVANCED_FACE('',(#2107),#1444,.T.) ;
#15196=ADVANCED_FACE('',(#2108),#1445,.F.) ;
#15197=ADVANCED_FACE('',(#2109),#1446,.T.) ;
#15198=ADVANCED_FACE('',(#2110),#996,.T.) ;
#15199=ADVANCED_FACE('',(#2111),#997,.F.) ;
#15200=ADVANCED_FACE('',(#2112),#1447,.T.) ;
#15201=ADVANCED_FACE('',(#2113),#1448,.F.) ;
#15202=ADVANCED_FACE('',(#2114),#1449,.T.) ;
#15203=ADVANCED_FACE('',(#2115),#998,.T.) ;
#15204=ADVANCED_FACE('',(#2116),#999,.F.) ;
#15205=ADVANCED_FACE('',(#2117),#1450,.T.) ;
#15206=ADVANCED_FACE('',(#2118),#1451,.F.) ;
#15207=ADVANCED_FACE('',(#2119),#1452,.T.) ;
#15208=ADVANCED_FACE('',(#2120),#1000,.T.) ;
#15209=ADVANCED_FACE('',(#2121),#1001,.F.) ;
#15210=ADVANCED_FACE('',(#2122),#1453,.T.) ;
#15211=ADVANCED_FACE('',(#2123),#1454,.F.) ;
#15212=ADVANCED_FACE('',(#2124),#1455,.T.) ;
#15213=ADVANCED_FACE('',(#2125),#1002,.T.) ;
#15214=ADVANCED_FACE('',(#2126),#1003,.F.) ;
#15215=ADVANCED_FACE('',(#2127),#1456,.T.) ;
#15216=ADVANCED_FACE('',(#2128),#1457,.F.) ;
#15217=ADVANCED_FACE('',(#2129),#1458,.T.) ;
#15218=ADVANCED_FACE('',(#2130),#1004,.T.) ;
#15219=ADVANCED_FACE('',(#2131),#1005,.F.) ;
#15220=ADVANCED_FACE('',(#2132),#1459,.T.) ;
#15221=ADVANCED_FACE('',(#2133),#1460,.F.) ;
#15222=ADVANCED_FACE('',(#2134),#1461,.T.) ;
#15223=ADVANCED_FACE('',(#2135),#1006,.T.) ;
#15224=ADVANCED_FACE('',(#2136),#1007,.F.) ;
#15225=ADVANCED_FACE('',(#2137),#1462,.T.) ;
#15226=ADVANCED_FACE('',(#2138),#1463,.F.) ;
#15227=ADVANCED_FACE('',(#2139),#1464,.T.) ;
#15228=ADVANCED_FACE('',(#2140),#1008,.T.) ;
#15229=ADVANCED_FACE('',(#2141),#1009,.F.) ;
#15230=ADVANCED_FACE('',(#2142),#1465,.T.) ;
#15231=ADVANCED_FACE('',(#2143),#1466,.F.) ;
#15232=ADVANCED_FACE('',(#2144),#1467,.T.) ;
#15233=ADVANCED_FACE('',(#2145),#1010,.T.) ;
#15234=ADVANCED_FACE('',(#2146),#1011,.F.) ;
#15235=ADVANCED_FACE('',(#2147),#1468,.T.) ;
#15236=ADVANCED_FACE('',(#2148),#1469,.F.) ;
#15237=ADVANCED_FACE('',(#2149),#1470,.T.) ;
#15238=ADVANCED_FACE('',(#2150),#1012,.T.) ;
#15239=ADVANCED_FACE('',(#2151),#1013,.F.) ;
#15240=ADVANCED_FACE('',(#2152),#1471,.T.) ;
#15241=ADVANCED_FACE('',(#2153),#1472,.F.) ;
#15242=ADVANCED_FACE('',(#2154),#1473,.T.) ;
#15243=ADVANCED_FACE('',(#2155),#1014,.T.) ;
#15244=ADVANCED_FACE('',(#2156),#1015,.F.) ;
#15245=ADVANCED_FACE('',(#2157),#1474,.T.) ;
#15246=ADVANCED_FACE('',(#2158),#1475,.F.) ;
#15247=ADVANCED_FACE('',(#2159),#1476,.T.) ;
#15248=ADVANCED_FACE('',(#2160),#1016,.T.) ;
#15249=ADVANCED_FACE('',(#2161),#1017,.F.) ;
#15250=ADVANCED_FACE('',(#2162),#1477,.T.) ;
#15251=ADVANCED_FACE('',(#2163),#1478,.F.) ;
#15252=ADVANCED_FACE('',(#2164),#1479,.T.) ;
#15253=ADVANCED_FACE('',(#2165),#1018,.T.) ;
#15254=ADVANCED_FACE('',(#2166),#1019,.F.) ;
#15255=ADVANCED_FACE('',(#2167),#1480,.T.) ;
#15256=ADVANCED_FACE('',(#2168),#1481,.F.) ;
#15257=ADVANCED_FACE('',(#2169),#1482,.T.) ;
#15258=ADVANCED_FACE('',(#2170),#1020,.T.) ;
#15259=ADVANCED_FACE('',(#2171),#1021,.F.) ;
#15260=ADVANCED_FACE('',(#2172),#1483,.T.) ;
#15261=ADVANCED_FACE('',(#2173),#1484,.F.) ;
#15262=ADVANCED_FACE('',(#2174),#1485,.T.) ;
#15263=ADVANCED_FACE('',(#2175),#1022,.T.) ;
#15264=ADVANCED_FACE('',(#2176),#1023,.F.) ;
#15265=ADVANCED_FACE('',(#2177),#1486,.T.) ;
#15266=ADVANCED_FACE('',(#2178),#1487,.F.) ;
#15267=ADVANCED_FACE('',(#2179),#1488,.T.) ;
#15268=ADVANCED_FACE('',(#2180),#1024,.T.) ;
#15269=ADVANCED_FACE('',(#2181),#1025,.F.) ;
#15270=ADVANCED_FACE('',(#2182),#1489,.T.) ;
#15271=ADVANCED_FACE('',(#2183),#1490,.F.) ;
#15272=ADVANCED_FACE('',(#2184),#1491,.T.) ;
#15273=ADVANCED_FACE('',(#2185),#1026,.T.) ;
#15274=ADVANCED_FACE('',(#2186),#1027,.F.) ;
#15275=ADVANCED_FACE('',(#2187),#1492,.T.) ;
#15276=ADVANCED_FACE('',(#2188),#1493,.F.) ;
#15277=ADVANCED_FACE('',(#2189),#1494,.T.) ;
#15278=ADVANCED_FACE('',(#2190),#1028,.T.) ;
#15279=ADVANCED_FACE('',(#2191),#1029,.F.) ;
#15280=ADVANCED_FACE('',(#2192),#1495,.T.) ;
#15281=ADVANCED_FACE('',(#2193),#1496,.F.) ;
#15282=ADVANCED_FACE('',(#2194),#1497,.T.) ;
#15283=ADVANCED_FACE('',(#2195),#1030,.T.) ;
#15284=ADVANCED_FACE('',(#2196),#1031,.F.) ;
#15285=ADVANCED_FACE('',(#2197),#1498,.T.) ;
#15286=ADVANCED_FACE('',(#2198),#1499,.F.) ;
#15287=ADVANCED_FACE('',(#2199),#1500,.T.) ;
#15288=ADVANCED_FACE('',(#2200),#1032,.T.) ;
#15289=ADVANCED_FACE('',(#2201),#1033,.F.) ;
#15290=ADVANCED_FACE('',(#2202),#1501,.T.) ;
#15291=ADVANCED_FACE('',(#2203),#1502,.F.) ;
#15292=ADVANCED_FACE('',(#2204),#1503,.T.) ;
#15293=ADVANCED_FACE('',(#2205),#1034,.T.) ;
#15294=ADVANCED_FACE('',(#2206),#1035,.F.) ;
#15295=ADVANCED_FACE('',(#2207),#1504,.T.) ;
#15296=ADVANCED_FACE('',(#2208),#1505,.F.) ;
#15297=ADVANCED_FACE('',(#2209),#1506,.T.) ;
#15298=ADVANCED_FACE('',(#2210),#1507,.F.) ;
#15502=CLOSED_SHELL('',(#14921,#14922,#14923,#14924,#14925,#14926,#14927,
#14928,#14929,#14930,#14931,#14932,#14933,#14934,#14935,#14936,#14937,#14938,
#14939,#14940,#14941,#14942,#14943,#14944,#14945,#14946,#14947,#14948,#14949,
#14950,#14951,#14952,#14953,#14954,#14955,#14956,#14957,#14958,#14959,#14960,
#14961,#14962,#14963,#14964,#14965,#14966,#14967,#14968,#14969,#14970,#14971,
#14972,#14973,#14974,#14975,#14976,#14977,#14978,#14979,#14980,#14981,#14982,
#14983,#14984,#14985,#14986,#14987,#14988,#14989,#14990,#14991,#14992,#14993,
#14994,#14995,#14996,#14997,#14998,#14999,#15000,#15001,#15002,#15003,#15004,
#15005,#15006,#15007,#15008,#15009,#15010,#15011,#15012,#15013,#15014,#15015,
#15016,#15017,#15018,#15019,#15020,#15021,#15022,#15023,#15024,#15025,#15026,
#15027,#15028,#15029,#15030,#15031,#15032,#15033,#15034,#15035,#15036,#15037,
#15038,#15039,#15040,#15041,#15042,#15043,#15044,#15045,#15046,#15047,#15048,
#15049,#15050,#15051,#15052,#15053,#15054,#15055,#15056,#15057,#15058,#15059,
#15060,#15061,#15062,#15063,#15064,#15065,#15066,#15067,#15068,#15069,#15070,
#15071,#15072,#15073,#15074,#15075,#15076,#15077,#15078,#15079,#15080,#15081,
#15082,#15083,#15084,#15085,#15086,#15087,#15088,#15089,#15090,#15091,#15092,
#15093,#15094,#15095,#15096,#15097,#15098,#15099,#15100,#15101,#15102,#15103,
#15104,#15105,#15106,#15107,#15108,#15109,#15110,#15111,#15112,#15113,#15114,
#15115,#15116,#15117,#15118,#15119,#15120,#15121,#15122,#15123,#15124,#15125,
#15126,#15127,#15128,#15129,#15130,#15131,#15132,#15133,#15134,#15135,#15136,
#15137,#15138,#15139,#15140,#15141,#15142,#15143,#15144,#15145,#15146,#15147,
#15148,#15149,#15150,#15151,#15152,#15153,#15154,#15155,#15156,#15157,#15158,
#15159,#15160,#15161,#15162,#15163,#15164,#15165,#15166,#15167,#15168,#15169,
#15170,#15171,#15172,#15173,#15174,#15175,#15176,#15177,#15178,#15179,#15180,
#15181,#15182,#15183,#15184,#15185,#15186,#15187,#15188,#15189,#15190,#15191,
#15192,#15193,#15194,#15195,#15196,#15197,#15198,#15199,#15200,#15201,#15202,
#15203,#15204,#15205,#15206,#15207,#15208,#15209,#15210,#15211,#15212,#15213,
#15214,#15215,#15216,#15217,#15218,#15219,#15220,#15221,#15222,#15223,#15224,
#15225,#15226,#15227,#15228,#15229,#15230,#15231,#15232,#15233,#15234,#15235,
#15236,#15237,#15238,#15239,#15240,#15241,#15242,#15243,#15244,#15245,#15246,
#15247,#15248,#15249,#15250,#15251,#15252,#15253,#15254,#15255,#15256,#15257,
#15258,#15259,#15260,#15261,#15262,#15263,#15264,#15265,#15266,#15267,#15268,
#15269,#15270,#15271,#15272,#15273,#15274,#15275,#15276,#15277,#15278,#15279,
#15280,#15281,#15282,#15283,#15284,#15285,#15286,#15287,#15288,#15289,#15290,
#15291,#15292,#15293,#15294,#15295,#15296,#15297,#15298)) ;
#16208=AXIS2_PLACEMENT_3D('',#51949,#19242,#19243) ;
#16209=AXIS2_PLACEMENT_3D('',#51950,#19244,#19245) ;
#16210=AXIS2_PLACEMENT_3D('',#51959,#19250,#19251) ;
#16211=AXIS2_PLACEMENT_3D('',#51965,#19255,#19256) ;
#16212=AXIS2_PLACEMENT_3D('',#51971,#19260,#19261) ;
#16213=AXIS2_PLACEMENT_3D('',#51973,#19262,#19263) ;
#16214=AXIS2_PLACEMENT_3D('',#51974,#19264,#19265) ;
#16215=AXIS2_PLACEMENT_3D('',#51975,#19266,#19267) ;
#16216=AXIS2_PLACEMENT_3D('',#51980,#19269,#19270) ;
#16217=AXIS2_PLACEMENT_3D('',#51983,#19272,#19273) ;
#16218=AXIS2_PLACEMENT_3D('',#51984,#19274,#19275) ;
#16219=AXIS2_PLACEMENT_3D('',#51987,#19276,#19277) ;
#16220=AXIS2_PLACEMENT_3D('',#51991,#19279,#19280) ;
#16221=AXIS2_PLACEMENT_3D('',#51993,#19282,#19283) ;
#16222=AXIS2_PLACEMENT_3D('',#51996,#19284,#19285) ;
#16223=AXIS2_PLACEMENT_3D('',#52000,#19287,#19288) ;
#16224=AXIS2_PLACEMENT_3D('',#52002,#19290,#19291) ;
#16225=AXIS2_PLACEMENT_3D('',#52005,#19292,#19293) ;
#16226=AXIS2_PLACEMENT_3D('',#52009,#19295,#19296) ;
#16227=AXIS2_PLACEMENT_3D('',#52011,#19298,#19299) ;
#16228=AXIS2_PLACEMENT_3D('',#52016,#19301,#19302) ;
#16229=AXIS2_PLACEMENT_3D('',#52019,#19304,#19305) ;
#16230=AXIS2_PLACEMENT_3D('',#52020,#19306,#19307) ;
#16231=AXIS2_PLACEMENT_3D('',#52025,#19309,#19310) ;
#16232=AXIS2_PLACEMENT_3D('',#52028,#19312,#19313) ;
#16233=AXIS2_PLACEMENT_3D('',#52029,#19314,#19315) ;
#16234=AXIS2_PLACEMENT_3D('',#52034,#19317,#19318) ;
#16235=AXIS2_PLACEMENT_3D('',#52037,#19320,#19321) ;
#16236=AXIS2_PLACEMENT_3D('',#52038,#19322,#19323) ;
#16237=AXIS2_PLACEMENT_3D('',#52041,#19324,#19325) ;
#16238=AXIS2_PLACEMENT_3D('',#52045,#19327,#19328) ;
#16239=AXIS2_PLACEMENT_3D('',#52047,#19330,#19331) ;
#16240=AXIS2_PLACEMENT_3D('',#52050,#19332,#19333) ;
#16241=AXIS2_PLACEMENT_3D('',#52054,#19335,#19336) ;
#16242=AXIS2_PLACEMENT_3D('',#52056,#19338,#19339) ;
#16243=AXIS2_PLACEMENT_3D('',#52059,#19340,#19341) ;
#16244=AXIS2_PLACEMENT_3D('',#52063,#19343,#19344) ;
#16245=AXIS2_PLACEMENT_3D('',#52065,#19346,#19347) ;
#16246=AXIS2_PLACEMENT_3D('',#52068,#19348,#19349) ;
#16247=AXIS2_PLACEMENT_3D('',#52072,#19351,#19352) ;
#16248=AXIS2_PLACEMENT_3D('',#52074,#19354,#19355) ;
#16249=AXIS2_PLACEMENT_3D('',#52077,#19356,#19357) ;
#16250=AXIS2_PLACEMENT_3D('',#52081,#19359,#19360) ;
#16251=AXIS2_PLACEMENT_3D('',#52083,#19362,#19363) ;
#16252=AXIS2_PLACEMENT_3D('',#52086,#19364,#19365) ;
#16253=AXIS2_PLACEMENT_3D('',#52090,#19367,#19368) ;
#16254=AXIS2_PLACEMENT_3D('',#52092,#19370,#19371) ;
#16255=AXIS2_PLACEMENT_3D('',#52095,#19372,#19373) ;
#16256=AXIS2_PLACEMENT_3D('',#52099,#19375,#19376) ;
#16257=AXIS2_PLACEMENT_3D('',#52101,#19378,#19379) ;
#16258=AXIS2_PLACEMENT_3D('',#52104,#19380,#19381) ;
#16259=AXIS2_PLACEMENT_3D('',#52108,#19383,#19384) ;
#16260=AXIS2_PLACEMENT_3D('',#52110,#19386,#19387) ;
#16261=AXIS2_PLACEMENT_3D('',#52113,#19388,#19389) ;
#16262=AXIS2_PLACEMENT_3D('',#52117,#19391,#19392) ;
#16263=AXIS2_PLACEMENT_3D('',#52119,#19394,#19395) ;
#16264=AXIS2_PLACEMENT_3D('',#52122,#19396,#19397) ;
#16265=AXIS2_PLACEMENT_3D('',#52126,#19399,#19400) ;
#16266=AXIS2_PLACEMENT_3D('',#52128,#19402,#19403) ;
#16267=AXIS2_PLACEMENT_3D('',#52131,#19404,#19405) ;
#16268=AXIS2_PLACEMENT_3D('',#52135,#19407,#19408) ;
#16269=AXIS2_PLACEMENT_3D('',#52137,#19410,#19411) ;
#16270=AXIS2_PLACEMENT_3D('',#52140,#19412,#19413) ;
#16271=AXIS2_PLACEMENT_3D('',#52144,#19415,#19416) ;
#16272=AXIS2_PLACEMENT_3D('',#52146,#19418,#19419) ;
#16273=AXIS2_PLACEMENT_3D('',#52149,#19420,#19421) ;
#16274=AXIS2_PLACEMENT_3D('',#52153,#19423,#19424) ;
#16275=AXIS2_PLACEMENT_3D('',#52155,#19426,#19427) ;
#16276=AXIS2_PLACEMENT_3D('',#52160,#19429,#19430) ;
#16277=AXIS2_PLACEMENT_3D('',#52163,#19432,#19433) ;
#16278=AXIS2_PLACEMENT_3D('',#52164,#19434,#19435) ;
#16279=AXIS2_PLACEMENT_3D('',#52167,#19436,#19437) ;
#16280=AXIS2_PLACEMENT_3D('',#52171,#19439,#19440) ;
#16281=AXIS2_PLACEMENT_3D('',#52173,#19442,#19443) ;
#16282=AXIS2_PLACEMENT_3D('',#52176,#19444,#19445) ;
#16283=AXIS2_PLACEMENT_3D('',#52180,#19447,#19448) ;
#16284=AXIS2_PLACEMENT_3D('',#52182,#19450,#19451) ;
#16285=AXIS2_PLACEMENT_3D('',#52185,#19452,#19453) ;
#16286=AXIS2_PLACEMENT_3D('',#52189,#19455,#19456) ;
#16287=AXIS2_PLACEMENT_3D('',#52191,#19458,#19459) ;
#16288=AXIS2_PLACEMENT_3D('',#52194,#19460,#19461) ;
#16289=AXIS2_PLACEMENT_3D('',#52198,#19463,#19464) ;
#16290=AXIS2_PLACEMENT_3D('',#52200,#19466,#19467) ;
#16291=AXIS2_PLACEMENT_3D('',#52203,#19468,#19469) ;
#16292=AXIS2_PLACEMENT_3D('',#52207,#19471,#19472) ;
#16293=AXIS2_PLACEMENT_3D('',#52209,#19474,#19475) ;
#16294=AXIS2_PLACEMENT_3D('',#52212,#19476,#19477) ;
#16295=AXIS2_PLACEMENT_3D('',#52216,#19479,#19480) ;
#16296=AXIS2_PLACEMENT_3D('',#52218,#19482,#19483) ;
#16297=AXIS2_PLACEMENT_3D('',#52221,#19484,#19485) ;
#16298=AXIS2_PLACEMENT_3D('',#52225,#19487,#19488) ;
#16299=AXIS2_PLACEMENT_3D('',#52227,#19490,#19491) ;
#16300=AXIS2_PLACEMENT_3D('',#52230,#19492,#19493) ;
#16301=AXIS2_PLACEMENT_3D('',#52234,#19495,#19496) ;
#16302=AXIS2_PLACEMENT_3D('',#52236,#19498,#19499) ;
#16303=AXIS2_PLACEMENT_3D('',#52239,#19500,#19501) ;
#16304=AXIS2_PLACEMENT_3D('',#52243,#19503,#19504) ;
#16305=AXIS2_PLACEMENT_3D('',#52245,#19506,#19507) ;
#16306=AXIS2_PLACEMENT_3D('',#52248,#19508,#19509) ;
#16307=AXIS2_PLACEMENT_3D('',#52252,#19511,#19512) ;
#16308=AXIS2_PLACEMENT_3D('',#52254,#19514,#19515) ;
#16309=AXIS2_PLACEMENT_3D('',#52257,#19516,#19517) ;
#16310=AXIS2_PLACEMENT_3D('',#52261,#19519,#19520) ;
#16311=AXIS2_PLACEMENT_3D('',#52263,#19522,#19523) ;
#16312=AXIS2_PLACEMENT_3D('',#52268,#19525,#19526) ;
#16313=AXIS2_PLACEMENT_3D('',#52271,#19528,#19529) ;
#16314=AXIS2_PLACEMENT_3D('',#52272,#19530,#19531) ;
#16315=AXIS2_PLACEMENT_3D('',#52277,#19533,#19534) ;
#16316=AXIS2_PLACEMENT_3D('',#52280,#19536,#19537) ;
#16317=AXIS2_PLACEMENT_3D('',#52281,#19538,#19539) ;
#16318=AXIS2_PLACEMENT_3D('',#52286,#19541,#19542) ;
#16319=AXIS2_PLACEMENT_3D('',#52289,#19544,#19545) ;
#16320=AXIS2_PLACEMENT_3D('',#52290,#19546,#19547) ;
#16321=AXIS2_PLACEMENT_3D('',#52295,#19549,#19550) ;
#16322=AXIS2_PLACEMENT_3D('',#52298,#19552,#19553) ;
#16323=AXIS2_PLACEMENT_3D('',#52299,#19554,#19555) ;
#16324=AXIS2_PLACEMENT_3D('',#52304,#19557,#19558) ;
#16325=AXIS2_PLACEMENT_3D('',#52307,#19560,#19561) ;
#16326=AXIS2_PLACEMENT_3D('',#52308,#19562,#19563) ;
#16327=AXIS2_PLACEMENT_3D('',#52313,#19565,#19566) ;
#16328=AXIS2_PLACEMENT_3D('',#52316,#19568,#19569) ;
#16329=AXIS2_PLACEMENT_3D('',#52317,#19570,#19571) ;
#16330=AXIS2_PLACEMENT_3D('',#52322,#19573,#19574) ;
#16331=AXIS2_PLACEMENT_3D('',#52325,#19576,#19577) ;
#16332=AXIS2_PLACEMENT_3D('',#52326,#19578,#19579) ;
#16333=AXIS2_PLACEMENT_3D('',#52329,#19580,#19581) ;
#16334=AXIS2_PLACEMENT_3D('',#52333,#19583,#19584) ;
#16335=AXIS2_PLACEMENT_3D('',#52335,#19586,#19587) ;
#16336=AXIS2_PLACEMENT_3D('',#52338,#19588,#19589) ;
#16337=AXIS2_PLACEMENT_3D('',#52342,#19591,#19592) ;
#16338=AXIS2_PLACEMENT_3D('',#52344,#19594,#19595) ;
#16339=AXIS2_PLACEMENT_3D('',#52347,#19596,#19597) ;
#16340=AXIS2_PLACEMENT_3D('',#52351,#19599,#19600) ;
#16341=AXIS2_PLACEMENT_3D('',#52353,#19602,#19603) ;
#16342=AXIS2_PLACEMENT_3D('',#52356,#19604,#19605) ;
#16343=AXIS2_PLACEMENT_3D('',#52360,#19607,#19608) ;
#16344=AXIS2_PLACEMENT_3D('',#52362,#19610,#19611) ;
#16345=AXIS2_PLACEMENT_3D('',#52365,#19612,#19613) ;
#16346=AXIS2_PLACEMENT_3D('',#52369,#19615,#19616) ;
#16347=AXIS2_PLACEMENT_3D('',#52371,#19618,#19619) ;
#16348=AXIS2_PLACEMENT_3D('',#52374,#19620,#19621) ;
#16349=AXIS2_PLACEMENT_3D('',#52378,#19623,#19624) ;
#16350=AXIS2_PLACEMENT_3D('',#52380,#19626,#19627) ;
#16351=AXIS2_PLACEMENT_3D('',#52383,#19628,#19629) ;
#16352=AXIS2_PLACEMENT_3D('',#52387,#19631,#19632) ;
#16353=AXIS2_PLACEMENT_3D('',#52389,#19634,#19635) ;
#16354=AXIS2_PLACEMENT_3D('',#52392,#19636,#19637) ;
#16355=AXIS2_PLACEMENT_3D('',#52396,#19639,#19640) ;
#16356=AXIS2_PLACEMENT_3D('',#52398,#19642,#19643) ;
#16357=AXIS2_PLACEMENT_3D('',#52401,#19644,#19645) ;
#16358=AXIS2_PLACEMENT_3D('',#52405,#19647,#19648) ;
#16359=AXIS2_PLACEMENT_3D('',#52407,#19650,#19651) ;
#16360=AXIS2_PLACEMENT_3D('',#52410,#19652,#19653) ;
#16361=AXIS2_PLACEMENT_3D('',#52414,#19655,#19656) ;
#16362=AXIS2_PLACEMENT_3D('',#52416,#19658,#19659) ;
#16363=AXIS2_PLACEMENT_3D('',#52419,#19660,#19661) ;
#16364=AXIS2_PLACEMENT_3D('',#52423,#19663,#19664) ;
#16365=AXIS2_PLACEMENT_3D('',#52425,#19666,#19667) ;
#16366=AXIS2_PLACEMENT_3D('',#52430,#19669,#19670) ;
#16367=AXIS2_PLACEMENT_3D('',#52433,#19672,#19673) ;
#16368=AXIS2_PLACEMENT_3D('',#52434,#19674,#19675) ;
#16369=AXIS2_PLACEMENT_3D('',#52437,#19676,#19677) ;
#16370=AXIS2_PLACEMENT_3D('',#52441,#19679,#19680) ;
#16371=AXIS2_PLACEMENT_3D('',#52443,#19682,#19683) ;
#16372=AXIS2_PLACEMENT_3D('',#52446,#19684,#19685) ;
#16373=AXIS2_PLACEMENT_3D('',#52450,#19687,#19688) ;
#16374=AXIS2_PLACEMENT_3D('',#52452,#19690,#19691) ;
#16375=AXIS2_PLACEMENT_3D('',#52455,#19692,#19693) ;
#16376=AXIS2_PLACEMENT_3D('',#52459,#19695,#19696) ;
#16377=AXIS2_PLACEMENT_3D('',#52461,#19698,#19699) ;
#16378=AXIS2_PLACEMENT_3D('',#52464,#19700,#19701) ;
#16379=AXIS2_PLACEMENT_3D('',#52468,#19703,#19704) ;
#16380=AXIS2_PLACEMENT_3D('',#52470,#19706,#19707) ;
#16381=AXIS2_PLACEMENT_3D('',#52473,#19708,#19709) ;
#16382=AXIS2_PLACEMENT_3D('',#52477,#19711,#19712) ;
#16383=AXIS2_PLACEMENT_3D('',#52479,#19714,#19715) ;
#16384=AXIS2_PLACEMENT_3D('',#52482,#19716,#19717) ;
#16385=AXIS2_PLACEMENT_3D('',#52486,#19719,#19720) ;
#16386=AXIS2_PLACEMENT_3D('',#52488,#19722,#19723) ;
#16387=AXIS2_PLACEMENT_3D('',#52491,#19724,#19725) ;
#16388=AXIS2_PLACEMENT_3D('',#52495,#19727,#19728) ;
#16389=AXIS2_PLACEMENT_3D('',#52497,#19730,#19731) ;
#16390=AXIS2_PLACEMENT_3D('',#52502,#19733,#19734) ;
#16391=AXIS2_PLACEMENT_3D('',#52505,#19736,#19737) ;
#16392=AXIS2_PLACEMENT_3D('',#52506,#19738,#19739) ;
#16393=AXIS2_PLACEMENT_3D('',#52509,#19740,#19741) ;
#16394=AXIS2_PLACEMENT_3D('',#52513,#19743,#19744) ;
#16395=AXIS2_PLACEMENT_3D('',#52515,#19746,#19747) ;
#16396=AXIS2_PLACEMENT_3D('',#52517,#19748,#19749) ;
#16397=AXIS2_PLACEMENT_3D('',#52519,#19751,#19752) ;
#16398=AXIS2_PLACEMENT_3D('',#52521,#19753,#19754) ;
#16399=AXIS2_PLACEMENT_3D('',#52522,#19755,#19756) ;
#16400=AXIS2_PLACEMENT_3D('',#52526,#19758,#19759) ;
#16401=AXIS2_PLACEMENT_3D('',#52527,#19760,#19761) ;
#16402=AXIS2_PLACEMENT_3D('',#52528,#19762,#19763) ;
#16403=AXIS2_PLACEMENT_3D('',#52531,#19764,#19765) ;
#16404=AXIS2_PLACEMENT_3D('',#52532,#19766,#19767) ;
#16405=AXIS2_PLACEMENT_3D('',#52534,#19769,#19770) ;
#16406=AXIS2_PLACEMENT_3D('',#52537,#19772,#19773) ;
#16407=AXIS2_PLACEMENT_3D('',#52538,#19774,#19775) ;
#16408=AXIS2_PLACEMENT_3D('',#52539,#19776,#19777) ;
#16409=AXIS2_PLACEMENT_3D('',#52540,#19778,#19779) ;
#16410=AXIS2_PLACEMENT_3D('',#52541,#19780,#19781) ;
#16411=AXIS2_PLACEMENT_3D('',#52542,#19782,#19783) ;
#16412=AXIS2_PLACEMENT_3D('',#52543,#19784,#19785) ;
#16413=AXIS2_PLACEMENT_3D('',#52544,#19786,#19787) ;
#16414=AXIS2_PLACEMENT_3D('',#52545,#19788,#19789) ;
#16415=AXIS2_PLACEMENT_3D('',#52546,#19790,#19791) ;
#16416=AXIS2_PLACEMENT_3D('',#52547,#19792,#19793) ;
#16417=AXIS2_PLACEMENT_3D('',#52548,#19794,#19795) ;
#16418=AXIS2_PLACEMENT_3D('',#52549,#19796,#19797) ;
#16419=AXIS2_PLACEMENT_3D('',#52550,#19798,#19799) ;
#16420=AXIS2_PLACEMENT_3D('',#52551,#19800,#19801) ;
#16421=AXIS2_PLACEMENT_3D('',#52552,#19802,#19803) ;
#16422=AXIS2_PLACEMENT_3D('',#52553,#19804,#19805) ;
#16423=AXIS2_PLACEMENT_3D('',#52554,#19806,#19807) ;
#16424=AXIS2_PLACEMENT_3D('',#52555,#19808,#19809) ;
#16425=AXIS2_PLACEMENT_3D('',#52556,#19810,#19811) ;
#16426=AXIS2_PLACEMENT_3D('',#52557,#19812,#19813) ;
#16427=AXIS2_PLACEMENT_3D('',#52558,#19814,#19815) ;
#16428=AXIS2_PLACEMENT_3D('',#52559,#19816,#19817) ;
#16429=AXIS2_PLACEMENT_3D('',#52560,#19818,#19819) ;
#16430=AXIS2_PLACEMENT_3D('',#52561,#19820,#19821) ;
#16431=AXIS2_PLACEMENT_3D('',#52562,#19822,#19823) ;
#16432=AXIS2_PLACEMENT_3D('',#52563,#19824,#19825) ;
#16433=AXIS2_PLACEMENT_3D('',#52564,#19826,#19827) ;
#16434=AXIS2_PLACEMENT_3D('',#52565,#19828,#19829) ;
#16435=AXIS2_PLACEMENT_3D('',#52566,#19830,#19831) ;
#16436=AXIS2_PLACEMENT_3D('',#52567,#19832,#19833) ;
#16437=AXIS2_PLACEMENT_3D('',#52568,#19834,#19835) ;
#16438=AXIS2_PLACEMENT_3D('',#52569,#19836,#19837) ;
#16439=AXIS2_PLACEMENT_3D('',#52570,#19838,#19839) ;
#16440=AXIS2_PLACEMENT_3D('',#52571,#19840,#19841) ;
#16441=AXIS2_PLACEMENT_3D('',#52572,#19842,#19843) ;
#16442=AXIS2_PLACEMENT_3D('',#52573,#19844,#19845) ;
#16443=AXIS2_PLACEMENT_3D('',#52574,#19846,#19847) ;
#16444=AXIS2_PLACEMENT_3D('',#52575,#19848,#19849) ;
#16445=AXIS2_PLACEMENT_3D('',#52576,#19850,#19851) ;
#16446=AXIS2_PLACEMENT_3D('',#52577,#19852,#19853) ;
#16447=AXIS2_PLACEMENT_3D('',#52578,#19854,#19855) ;
#16448=AXIS2_PLACEMENT_3D('',#52579,#19856,#19857) ;
#16449=AXIS2_PLACEMENT_3D('',#52580,#19858,#19859) ;
#16450=AXIS2_PLACEMENT_3D('',#52581,#19860,#19861) ;
#16451=AXIS2_PLACEMENT_3D('',#52582,#19862,#19863) ;
#16452=AXIS2_PLACEMENT_3D('',#52583,#19864,#19865) ;
#16453=AXIS2_PLACEMENT_3D('',#52584,#19866,#19867) ;
#16454=AXIS2_PLACEMENT_3D('',#52585,#19868,#19869) ;
#16455=AXIS2_PLACEMENT_3D('',#52586,#19870,#19871) ;
#16456=AXIS2_PLACEMENT_3D('',#52587,#19872,#19873) ;
#16457=AXIS2_PLACEMENT_3D('',#52588,#19874,#19875) ;
#16458=AXIS2_PLACEMENT_3D('',#52589,#19876,#19877) ;
#16459=AXIS2_PLACEMENT_3D('',#52590,#19878,#19879) ;
#16460=AXIS2_PLACEMENT_3D('',#52591,#19880,#19881) ;
#16461=AXIS2_PLACEMENT_3D('',#52592,#19882,#19883) ;
#16462=AXIS2_PLACEMENT_3D('',#52593,#19884,#19885) ;
#16463=AXIS2_PLACEMENT_3D('',#52594,#19886,#19887) ;
#16464=AXIS2_PLACEMENT_3D('',#52595,#19888,#19889) ;
#16465=AXIS2_PLACEMENT_3D('',#52596,#19890,#19891) ;
#16466=AXIS2_PLACEMENT_3D('',#52597,#19892,#19893) ;
#16467=AXIS2_PLACEMENT_3D('',#52598,#19894,#19895) ;
#16468=AXIS2_PLACEMENT_3D('',#52601,#19896,#19897) ;
#16469=AXIS2_PLACEMENT_3D('',#52602,#19898,#19899) ;
#16470=AXIS2_PLACEMENT_3D('',#52605,#19901,#19902) ;
#16471=AXIS2_PLACEMENT_3D('',#52606,#19903,#19904) ;
#16472=AXIS2_PLACEMENT_3D('',#52607,#19905,#19906) ;
#16473=AXIS2_PLACEMENT_3D('',#52608,#19907,#19908) ;
#16474=AXIS2_PLACEMENT_3D('',#52609,#19909,#19910) ;
#16475=AXIS2_PLACEMENT_3D('',#52610,#19911,#19912) ;
#16476=AXIS2_PLACEMENT_3D('',#52611,#19913,#19914) ;
#16477=AXIS2_PLACEMENT_3D('',#52612,#19915,#19916) ;
#16478=AXIS2_PLACEMENT_3D('',#52613,#19917,#19918) ;
#16479=AXIS2_PLACEMENT_3D('',#52614,#19919,#19920) ;
#16480=AXIS2_PLACEMENT_3D('',#52615,#19921,#19922) ;
#16481=AXIS2_PLACEMENT_3D('',#52616,#19923,#19924) ;
#16482=AXIS2_PLACEMENT_3D('',#52617,#19925,#19926) ;
#16483=AXIS2_PLACEMENT_3D('',#52618,#19927,#19928) ;
#16484=AXIS2_PLACEMENT_3D('',#52619,#19929,#19930) ;
#16485=AXIS2_PLACEMENT_3D('',#52620,#19931,#19932) ;
#16486=AXIS2_PLACEMENT_3D('',#52621,#19933,#19934) ;
#16487=AXIS2_PLACEMENT_3D('',#52622,#19935,#19936) ;
#16488=AXIS2_PLACEMENT_3D('',#52623,#19937,#19938) ;
#16489=AXIS2_PLACEMENT_3D('',#52624,#19939,#19940) ;
#16490=AXIS2_PLACEMENT_3D('',#52625,#19941,#19942) ;
#16491=AXIS2_PLACEMENT_3D('',#52626,#19943,#19944) ;
#16492=AXIS2_PLACEMENT_3D('',#52627,#19945,#19946) ;
#16493=AXIS2_PLACEMENT_3D('',#52628,#19947,#19948) ;
#16494=AXIS2_PLACEMENT_3D('',#52629,#19949,#19950) ;
#16495=AXIS2_PLACEMENT_3D('',#52630,#19951,#19952) ;
#16496=AXIS2_PLACEMENT_3D('',#52631,#19953,#19954) ;
#16497=AXIS2_PLACEMENT_3D('',#52632,#19955,#19956) ;
#16498=AXIS2_PLACEMENT_3D('',#52633,#19957,#19958) ;
#16499=AXIS2_PLACEMENT_3D('',#52634,#19959,#19960) ;
#16500=AXIS2_PLACEMENT_3D('',#52635,#19961,#19962) ;
#16501=AXIS2_PLACEMENT_3D('',#52636,#19963,#19964) ;
#16502=AXIS2_PLACEMENT_3D('',#52637,#19965,#19966) ;
#16503=AXIS2_PLACEMENT_3D('',#52638,#19967,#19968) ;
#16504=AXIS2_PLACEMENT_3D('',#52639,#19969,#19970) ;
#16505=AXIS2_PLACEMENT_3D('',#52640,#19971,#19972) ;
#16506=AXIS2_PLACEMENT_3D('',#52641,#19973,#19974) ;
#16507=AXIS2_PLACEMENT_3D('',#52642,#19975,#19976) ;
#16508=AXIS2_PLACEMENT_3D('',#52643,#19977,#19978) ;
#16509=AXIS2_PLACEMENT_3D('',#52644,#19979,#19980) ;
#16510=AXIS2_PLACEMENT_3D('',#52645,#19981,#19982) ;
#16511=AXIS2_PLACEMENT_3D('',#52646,#19983,#19984) ;
#16512=AXIS2_PLACEMENT_3D('',#52647,#19985,#19986) ;
#16513=AXIS2_PLACEMENT_3D('',#52648,#19987,#19988) ;
#16514=AXIS2_PLACEMENT_3D('',#52649,#19989,#19990) ;
#16515=AXIS2_PLACEMENT_3D('',#52650,#19991,#19992) ;
#16516=AXIS2_PLACEMENT_3D('',#52651,#19993,#19994) ;
#16517=AXIS2_PLACEMENT_3D('',#52652,#19995,#19996) ;
#16518=AXIS2_PLACEMENT_3D('',#52653,#19997,#19998) ;
#16519=AXIS2_PLACEMENT_3D('',#52654,#19999,#20000) ;
#16520=AXIS2_PLACEMENT_3D('',#52655,#20001,#20002) ;
#16521=AXIS2_PLACEMENT_3D('',#52656,#20003,#20004) ;
#16522=AXIS2_PLACEMENT_3D('',#52657,#20005,#20006) ;
#16523=AXIS2_PLACEMENT_3D('',#52658,#20007,#20008) ;
#16524=AXIS2_PLACEMENT_3D('',#52659,#20009,#20010) ;
#16525=AXIS2_PLACEMENT_3D('',#52660,#20011,#20012) ;
#16526=AXIS2_PLACEMENT_3D('',#52661,#20013,#20014) ;
#16527=AXIS2_PLACEMENT_3D('',#52662,#20015,#20016) ;
#16528=AXIS2_PLACEMENT_3D('',#52663,#20017,#20018) ;
#16529=AXIS2_PLACEMENT_3D('',#52664,#20019,#20020) ;
#16530=AXIS2_PLACEMENT_3D('',#52665,#20021,#20022) ;
#16531=AXIS2_PLACEMENT_3D('',#52666,#20023,#20024) ;
#16532=AXIS2_PLACEMENT_3D('',#52670,#20026,#20027) ;
#16533=AXIS2_PLACEMENT_3D('',#52671,#20028,#20029) ;
#16534=AXIS2_PLACEMENT_3D('',#52672,#20030,#20031) ;
#16535=AXIS2_PLACEMENT_3D('',#52674,#20032,#20033) ;
#16536=AXIS2_PLACEMENT_3D('',#52676,#20035,#20036) ;
#16537=AXIS2_PLACEMENT_3D('',#52678,#20037,#20038) ;
#16538=AXIS2_PLACEMENT_3D('',#52679,#20039,#20040) ;
#16539=AXIS2_PLACEMENT_3D('',#52681,#20041,#20042) ;
#16540=AXIS2_PLACEMENT_3D('',#52683,#20044,#20045) ;
#16541=AXIS2_PLACEMENT_3D('',#52685,#20046,#20047) ;
#16542=AXIS2_PLACEMENT_3D('',#52686,#20048,#20049) ;
#16543=AXIS2_PLACEMENT_3D('',#52688,#20050,#20051) ;
#16544=AXIS2_PLACEMENT_3D('',#52690,#20053,#20054) ;
#16545=AXIS2_PLACEMENT_3D('',#52691,#20055,#20056) ;
#16546=AXIS2_PLACEMENT_3D('',#52692,#20057,#20058) ;
#16547=AXIS2_PLACEMENT_3D('',#52694,#20059,#20060) ;
#16548=AXIS2_PLACEMENT_3D('',#52696,#20061,#20062) ;
#16549=AXIS2_PLACEMENT_3D('',#52697,#20063,#20064) ;
#16550=AXIS2_PLACEMENT_3D('',#52698,#20065,#20066) ;
#16551=AXIS2_PLACEMENT_3D('',#52700,#20067,#20068) ;
#16552=AXIS2_PLACEMENT_3D('',#52702,#20069,#20070) ;
#16553=AXIS2_PLACEMENT_3D('',#52703,#20071,#20072) ;
#16554=AXIS2_PLACEMENT_3D('',#52704,#20073,#20074) ;
#16555=AXIS2_PLACEMENT_3D('',#52706,#20076,#20077) ;
#16556=AXIS2_PLACEMENT_3D('',#52708,#20079,#20080) ;
#16557=AXIS2_PLACEMENT_3D('',#52709,#20081,#20082) ;
#16558=AXIS2_PLACEMENT_3D('',#52711,#20083,#20084) ;
#16559=AXIS2_PLACEMENT_3D('',#52713,#20085,#20086) ;
#16560=AXIS2_PLACEMENT_3D('',#52714,#20087,#20088) ;
#16561=AXIS2_PLACEMENT_3D('',#52715,#20089,#20090) ;
#16562=AXIS2_PLACEMENT_3D('',#52717,#20091,#20092) ;
#16563=AXIS2_PLACEMENT_3D('',#52719,#20093,#20094) ;
#16564=AXIS2_PLACEMENT_3D('',#52720,#20095,#20096) ;
#16565=AXIS2_PLACEMENT_3D('',#52721,#20097,#20098) ;
#16566=AXIS2_PLACEMENT_3D('',#52723,#20100,#20101) ;
#16567=AXIS2_PLACEMENT_3D('',#52725,#20103,#20104) ;
#16568=AXIS2_PLACEMENT_3D('',#52726,#20105,#20106) ;
#16569=AXIS2_PLACEMENT_3D('',#52728,#20107,#20108) ;
#16570=AXIS2_PLACEMENT_3D('',#52730,#20109,#20110) ;
#16571=AXIS2_PLACEMENT_3D('',#52731,#20111,#20112) ;
#16572=AXIS2_PLACEMENT_3D('',#52732,#20113,#20114) ;
#16573=AXIS2_PLACEMENT_3D('',#52734,#20115,#20116) ;
#16574=AXIS2_PLACEMENT_3D('',#52736,#20117,#20118) ;
#16575=AXIS2_PLACEMENT_3D('',#52737,#20119,#20120) ;
#16576=AXIS2_PLACEMENT_3D('',#52738,#20121,#20122) ;
#16577=AXIS2_PLACEMENT_3D('',#52740,#20124,#20125) ;
#16578=AXIS2_PLACEMENT_3D('',#52742,#20127,#20128) ;
#16579=AXIS2_PLACEMENT_3D('',#52743,#20129,#20130) ;
#16580=AXIS2_PLACEMENT_3D('',#52745,#20131,#20132) ;
#16581=AXIS2_PLACEMENT_3D('',#52747,#20133,#20134) ;
#16582=AXIS2_PLACEMENT_3D('',#52748,#20135,#20136) ;
#16583=AXIS2_PLACEMENT_3D('',#52749,#20137,#20138) ;
#16584=AXIS2_PLACEMENT_3D('',#52751,#20139,#20140) ;
#16585=AXIS2_PLACEMENT_3D('',#52753,#20141,#20142) ;
#16586=AXIS2_PLACEMENT_3D('',#52754,#20143,#20144) ;
#16587=AXIS2_PLACEMENT_3D('',#52755,#20145,#20146) ;
#16588=AXIS2_PLACEMENT_3D('',#52757,#20148,#20149) ;
#16589=AXIS2_PLACEMENT_3D('',#52759,#20151,#20152) ;
#16590=AXIS2_PLACEMENT_3D('',#52760,#20153,#20154) ;
#16591=AXIS2_PLACEMENT_3D('',#52762,#20155,#20156) ;
#16592=AXIS2_PLACEMENT_3D('',#52764,#20157,#20158) ;
#16593=AXIS2_PLACEMENT_3D('',#52765,#20159,#20160) ;
#16594=AXIS2_PLACEMENT_3D('',#52766,#20161,#20162) ;
#16595=AXIS2_PLACEMENT_3D('',#52768,#20163,#20164) ;
#16596=AXIS2_PLACEMENT_3D('',#52770,#20165,#20166) ;
#16597=AXIS2_PLACEMENT_3D('',#52771,#20167,#20168) ;
#16598=AXIS2_PLACEMENT_3D('',#52772,#20169,#20170) ;
#16599=AXIS2_PLACEMENT_3D('',#52774,#20172,#20173) ;
#16600=AXIS2_PLACEMENT_3D('',#52776,#20175,#20176) ;
#16601=AXIS2_PLACEMENT_3D('',#52777,#20177,#20178) ;
#16602=AXIS2_PLACEMENT_3D('',#52779,#20179,#20180) ;
#16603=AXIS2_PLACEMENT_3D('',#52781,#20181,#20182) ;
#16604=AXIS2_PLACEMENT_3D('',#52782,#20183,#20184) ;
#16605=AXIS2_PLACEMENT_3D('',#52783,#20185,#20186) ;
#16606=AXIS2_PLACEMENT_3D('',#52785,#20187,#20188) ;
#16607=AXIS2_PLACEMENT_3D('',#52787,#20189,#20190) ;
#16608=AXIS2_PLACEMENT_3D('',#52788,#20191,#20192) ;
#16609=AXIS2_PLACEMENT_3D('',#52789,#20193,#20194) ;
#16610=AXIS2_PLACEMENT_3D('',#52791,#20196,#20197) ;
#16611=AXIS2_PLACEMENT_3D('',#52793,#20199,#20200) ;
#16612=AXIS2_PLACEMENT_3D('',#52794,#20201,#20202) ;
#16613=AXIS2_PLACEMENT_3D('',#52796,#20203,#20204) ;
#16614=AXIS2_PLACEMENT_3D('',#52798,#20205,#20206) ;
#16615=AXIS2_PLACEMENT_3D('',#52799,#20207,#20208) ;
#16616=AXIS2_PLACEMENT_3D('',#52800,#20209,#20210) ;
#16617=AXIS2_PLACEMENT_3D('',#52802,#20211,#20212) ;
#16618=AXIS2_PLACEMENT_3D('',#52804,#20213,#20214) ;
#16619=AXIS2_PLACEMENT_3D('',#52805,#20215,#20216) ;
#16620=AXIS2_PLACEMENT_3D('',#52806,#20217,#20218) ;
#16621=AXIS2_PLACEMENT_3D('',#52808,#20220,#20221) ;
#16622=AXIS2_PLACEMENT_3D('',#52810,#20223,#20224) ;
#16623=AXIS2_PLACEMENT_3D('',#52811,#20225,#20226) ;
#16624=AXIS2_PLACEMENT_3D('',#52813,#20227,#20228) ;
#16625=AXIS2_PLACEMENT_3D('',#52815,#20229,#20230) ;
#16626=AXIS2_PLACEMENT_3D('',#52816,#20231,#20232) ;
#16627=AXIS2_PLACEMENT_3D('',#52817,#20233,#20234) ;
#16628=AXIS2_PLACEMENT_3D('',#52819,#20235,#20236) ;
#16629=AXIS2_PLACEMENT_3D('',#52821,#20237,#20238) ;
#16630=AXIS2_PLACEMENT_3D('',#52822,#20239,#20240) ;
#16631=AXIS2_PLACEMENT_3D('',#52823,#20241,#20242) ;
#16632=AXIS2_PLACEMENT_3D('',#52825,#20244,#20245) ;
#16633=AXIS2_PLACEMENT_3D('',#52827,#20247,#20248) ;
#16634=AXIS2_PLACEMENT_3D('',#52828,#20249,#20250) ;
#16635=AXIS2_PLACEMENT_3D('',#52830,#20251,#20252) ;
#16636=AXIS2_PLACEMENT_3D('',#52832,#20253,#20254) ;
#16637=AXIS2_PLACEMENT_3D('',#52833,#20255,#20256) ;
#16638=AXIS2_PLACEMENT_3D('',#52834,#20257,#20258) ;
#16639=AXIS2_PLACEMENT_3D('',#52836,#20259,#20260) ;
#16640=AXIS2_PLACEMENT_3D('',#52838,#20261,#20262) ;
#16641=AXIS2_PLACEMENT_3D('',#52839,#20263,#20264) ;
#16642=AXIS2_PLACEMENT_3D('',#52840,#20265,#20266) ;
#16643=AXIS2_PLACEMENT_3D('',#52842,#20268,#20269) ;
#16644=AXIS2_PLACEMENT_3D('',#52844,#20271,#20272) ;
#16645=AXIS2_PLACEMENT_3D('',#52845,#20273,#20274) ;
#16646=AXIS2_PLACEMENT_3D('',#52847,#20275,#20276) ;
#16647=AXIS2_PLACEMENT_3D('',#52849,#20277,#20278) ;
#16648=AXIS2_PLACEMENT_3D('',#52850,#20279,#20280) ;
#16649=AXIS2_PLACEMENT_3D('',#52851,#20281,#20282) ;
#16650=AXIS2_PLACEMENT_3D('',#52853,#20283,#20284) ;
#16651=AXIS2_PLACEMENT_3D('',#52855,#20285,#20286) ;
#16652=AXIS2_PLACEMENT_3D('',#52856,#20287,#20288) ;
#16653=AXIS2_PLACEMENT_3D('',#52857,#20289,#20290) ;
#16654=AXIS2_PLACEMENT_3D('',#52859,#20292,#20293) ;
#16655=AXIS2_PLACEMENT_3D('',#52861,#20295,#20296) ;
#16656=AXIS2_PLACEMENT_3D('',#52862,#20297,#20298) ;
#16657=AXIS2_PLACEMENT_3D('',#52864,#20299,#20300) ;
#16658=AXIS2_PLACEMENT_3D('',#52866,#20301,#20302) ;
#16659=AXIS2_PLACEMENT_3D('',#52867,#20303,#20304) ;
#16660=AXIS2_PLACEMENT_3D('',#52868,#20305,#20306) ;
#16661=AXIS2_PLACEMENT_3D('',#52870,#20307,#20308) ;
#16662=AXIS2_PLACEMENT_3D('',#52872,#20309,#20310) ;
#16663=AXIS2_PLACEMENT_3D('',#52873,#20311,#20312) ;
#16664=AXIS2_PLACEMENT_3D('',#52874,#20313,#20314) ;
#16665=AXIS2_PLACEMENT_3D('',#52876,#20316,#20317) ;
#16666=AXIS2_PLACEMENT_3D('',#52878,#20319,#20320) ;
#16667=AXIS2_PLACEMENT_3D('',#52879,#20321,#20322) ;
#16668=AXIS2_PLACEMENT_3D('',#52881,#20323,#20324) ;
#16669=AXIS2_PLACEMENT_3D('',#52883,#20325,#20326) ;
#16670=AXIS2_PLACEMENT_3D('',#52884,#20327,#20328) ;
#16671=AXIS2_PLACEMENT_3D('',#52885,#20329,#20330) ;
#16672=AXIS2_PLACEMENT_3D('',#52887,#20331,#20332) ;
#16673=AXIS2_PLACEMENT_3D('',#52889,#20333,#20334) ;
#16674=AXIS2_PLACEMENT_3D('',#52890,#20335,#20336) ;
#16675=AXIS2_PLACEMENT_3D('',#52891,#20337,#20338) ;
#16676=AXIS2_PLACEMENT_3D('',#52893,#20340,#20341) ;
#16677=AXIS2_PLACEMENT_3D('',#52895,#20343,#20344) ;
#16678=AXIS2_PLACEMENT_3D('',#52896,#20345,#20346) ;
#16679=AXIS2_PLACEMENT_3D('',#52898,#20347,#20348) ;
#16680=AXIS2_PLACEMENT_3D('',#52900,#20349,#20350) ;
#16681=AXIS2_PLACEMENT_3D('',#52901,#20351,#20352) ;
#16682=AXIS2_PLACEMENT_3D('',#52902,#20353,#20354) ;
#16683=AXIS2_PLACEMENT_3D('',#52904,#20355,#20356) ;
#16684=AXIS2_PLACEMENT_3D('',#52906,#20357,#20358) ;
#16685=AXIS2_PLACEMENT_3D('',#52907,#20359,#20360) ;
#16686=AXIS2_PLACEMENT_3D('',#52908,#20361,#20362) ;
#16687=AXIS2_PLACEMENT_3D('',#52910,#20364,#20365) ;
#16688=AXIS2_PLACEMENT_3D('',#52912,#20367,#20368) ;
#16689=AXIS2_PLACEMENT_3D('',#52913,#20369,#20370) ;
#16690=AXIS2_PLACEMENT_3D('',#52915,#20371,#20372) ;
#16691=AXIS2_PLACEMENT_3D('',#52917,#20373,#20374) ;
#16692=AXIS2_PLACEMENT_3D('',#52918,#20375,#20376) ;
#16693=AXIS2_PLACEMENT_3D('',#52919,#20377,#20378) ;
#16694=AXIS2_PLACEMENT_3D('',#52921,#20379,#20380) ;
#16695=AXIS2_PLACEMENT_3D('',#52923,#20381,#20382) ;
#16696=AXIS2_PLACEMENT_3D('',#52924,#20383,#20384) ;
#16697=AXIS2_PLACEMENT_3D('',#52925,#20385,#20386) ;
#16698=AXIS2_PLACEMENT_3D('',#52927,#20388,#20389) ;
#16699=AXIS2_PLACEMENT_3D('',#52929,#20391,#20392) ;
#16700=AXIS2_PLACEMENT_3D('',#52930,#20393,#20394) ;
#16701=AXIS2_PLACEMENT_3D('',#52932,#20395,#20396) ;
#16702=AXIS2_PLACEMENT_3D('',#52934,#20397,#20398) ;
#16703=AXIS2_PLACEMENT_3D('',#52935,#20399,#20400) ;
#16704=AXIS2_PLACEMENT_3D('',#52936,#20401,#20402) ;
#16705=AXIS2_PLACEMENT_3D('',#52938,#20403,#20404) ;
#16706=AXIS2_PLACEMENT_3D('',#52940,#20405,#20406) ;
#16707=AXIS2_PLACEMENT_3D('',#52941,#20407,#20408) ;
#16708=AXIS2_PLACEMENT_3D('',#52942,#20409,#20410) ;
#16709=AXIS2_PLACEMENT_3D('',#52944,#20412,#20413) ;
#16710=AXIS2_PLACEMENT_3D('',#52946,#20415,#20416) ;
#16711=AXIS2_PLACEMENT_3D('',#52947,#20417,#20418) ;
#16712=AXIS2_PLACEMENT_3D('',#52949,#20419,#20420) ;
#16713=AXIS2_PLACEMENT_3D('',#52951,#20421,#20422) ;
#16714=AXIS2_PLACEMENT_3D('',#52952,#20423,#20424) ;
#16715=AXIS2_PLACEMENT_3D('',#52953,#20425,#20426) ;
#16716=AXIS2_PLACEMENT_3D('',#52955,#20427,#20428) ;
#16717=AXIS2_PLACEMENT_3D('',#52957,#20429,#20430) ;
#16718=AXIS2_PLACEMENT_3D('',#52958,#20431,#20432) ;
#16719=AXIS2_PLACEMENT_3D('',#52959,#20433,#20434) ;
#16720=AXIS2_PLACEMENT_3D('',#52961,#20436,#20437) ;
#16721=AXIS2_PLACEMENT_3D('',#52963,#20439,#20440) ;
#16722=AXIS2_PLACEMENT_3D('',#52964,#20441,#20442) ;
#16723=AXIS2_PLACEMENT_3D('',#52966,#20443,#20444) ;
#16724=AXIS2_PLACEMENT_3D('',#52968,#20445,#20446) ;
#16725=AXIS2_PLACEMENT_3D('',#52969,#20447,#20448) ;
#16726=AXIS2_PLACEMENT_3D('',#52970,#20449,#20450) ;
#16727=AXIS2_PLACEMENT_3D('',#52972,#20451,#20452) ;
#16728=AXIS2_PLACEMENT_3D('',#52974,#20453,#20454) ;
#16729=AXIS2_PLACEMENT_3D('',#52975,#20455,#20456) ;
#16730=AXIS2_PLACEMENT_3D('',#52976,#20457,#20458) ;
#16731=AXIS2_PLACEMENT_3D('',#52978,#20460,#20461) ;
#16732=AXIS2_PLACEMENT_3D('',#52980,#20463,#20464) ;
#16733=AXIS2_PLACEMENT_3D('',#52981,#20465,#20466) ;
#16734=AXIS2_PLACEMENT_3D('',#52983,#20467,#20468) ;
#16735=AXIS2_PLACEMENT_3D('',#52985,#20469,#20470) ;
#16736=AXIS2_PLACEMENT_3D('',#52986,#20471,#20472) ;
#16737=AXIS2_PLACEMENT_3D('',#52987,#20473,#20474) ;
#16738=AXIS2_PLACEMENT_3D('',#52989,#20475,#20476) ;
#16739=AXIS2_PLACEMENT_3D('',#52991,#20477,#20478) ;
#16740=AXIS2_PLACEMENT_3D('',#52992,#20479,#20480) ;
#16741=AXIS2_PLACEMENT_3D('',#52993,#20481,#20482) ;
#16742=AXIS2_PLACEMENT_3D('',#52995,#20484,#20485) ;
#16743=AXIS2_PLACEMENT_3D('',#52997,#20487,#20488) ;
#16744=AXIS2_PLACEMENT_3D('',#52998,#20489,#20490) ;
#16745=AXIS2_PLACEMENT_3D('',#53000,#20491,#20492) ;
#16746=AXIS2_PLACEMENT_3D('',#53002,#20493,#20494) ;
#16747=AXIS2_PLACEMENT_3D('',#53003,#20495,#20496) ;
#16748=AXIS2_PLACEMENT_3D('',#53004,#20497,#20498) ;
#16749=AXIS2_PLACEMENT_3D('',#53006,#20499,#20500) ;
#16750=AXIS2_PLACEMENT_3D('',#53008,#20501,#20502) ;
#16751=AXIS2_PLACEMENT_3D('',#53009,#20503,#20504) ;
#16752=AXIS2_PLACEMENT_3D('',#53010,#20505,#20506) ;
#16753=AXIS2_PLACEMENT_3D('',#53012,#20508,#20509) ;
#16754=AXIS2_PLACEMENT_3D('',#53014,#20511,#20512) ;
#16755=AXIS2_PLACEMENT_3D('',#53015,#20513,#20514) ;
#16756=AXIS2_PLACEMENT_3D('',#53017,#20515,#20516) ;
#16757=AXIS2_PLACEMENT_3D('',#53019,#20517,#20518) ;
#16758=AXIS2_PLACEMENT_3D('',#53020,#20519,#20520) ;
#16759=AXIS2_PLACEMENT_3D('',#53021,#20521,#20522) ;
#16760=AXIS2_PLACEMENT_3D('',#53023,#20523,#20524) ;
#16761=AXIS2_PLACEMENT_3D('',#53025,#20525,#20526) ;
#16762=AXIS2_PLACEMENT_3D('',#53026,#20527,#20528) ;
#16763=AXIS2_PLACEMENT_3D('',#53027,#20529,#20530) ;
#16764=AXIS2_PLACEMENT_3D('',#53029,#20532,#20533) ;
#16765=AXIS2_PLACEMENT_3D('',#53031,#20535,#20536) ;
#16766=AXIS2_PLACEMENT_3D('',#53032,#20537,#20538) ;
#16767=AXIS2_PLACEMENT_3D('',#53034,#20539,#20540) ;
#16768=AXIS2_PLACEMENT_3D('',#53036,#20541,#20542) ;
#16769=AXIS2_PLACEMENT_3D('',#53037,#20543,#20544) ;
#16770=AXIS2_PLACEMENT_3D('',#53038,#20545,#20546) ;
#16771=AXIS2_PLACEMENT_3D('',#53040,#20547,#20548) ;
#16772=AXIS2_PLACEMENT_3D('',#53042,#20549,#20550) ;
#16773=AXIS2_PLACEMENT_3D('',#53043,#20551,#20552) ;
#16774=AXIS2_PLACEMENT_3D('',#53044,#20553,#20554) ;
#16775=AXIS2_PLACEMENT_3D('',#53046,#20556,#20557) ;
#16776=AXIS2_PLACEMENT_3D('',#53048,#20559,#20560) ;
#16777=AXIS2_PLACEMENT_3D('',#53049,#20561,#20562) ;
#16778=AXIS2_PLACEMENT_3D('',#53051,#20563,#20564) ;
#16779=AXIS2_PLACEMENT_3D('',#53053,#20565,#20566) ;
#16780=AXIS2_PLACEMENT_3D('',#53054,#20567,#20568) ;
#16781=AXIS2_PLACEMENT_3D('',#53055,#20569,#20570) ;
#16782=AXIS2_PLACEMENT_3D('',#53057,#20571,#20572) ;
#16783=AXIS2_PLACEMENT_3D('',#53059,#20573,#20574) ;
#16784=AXIS2_PLACEMENT_3D('',#53060,#20575,#20576) ;
#16785=AXIS2_PLACEMENT_3D('',#53061,#20577,#20578) ;
#16786=AXIS2_PLACEMENT_3D('',#53063,#20580,#20581) ;
#16787=AXIS2_PLACEMENT_3D('',#53065,#20583,#20584) ;
#16788=AXIS2_PLACEMENT_3D('',#53066,#20585,#20586) ;
#16789=AXIS2_PLACEMENT_3D('',#53068,#20587,#20588) ;
#16790=AXIS2_PLACEMENT_3D('',#53070,#20589,#20590) ;
#16791=AXIS2_PLACEMENT_3D('',#53071,#20591,#20592) ;
#16792=AXIS2_PLACEMENT_3D('',#53072,#20593,#20594) ;
#16793=AXIS2_PLACEMENT_3D('',#53074,#20595,#20596) ;
#16794=AXIS2_PLACEMENT_3D('',#53076,#20597,#20598) ;
#16795=AXIS2_PLACEMENT_3D('',#53077,#20599,#20600) ;
#16796=AXIS2_PLACEMENT_3D('',#53078,#20601,#20602) ;
#16797=AXIS2_PLACEMENT_3D('',#53080,#20604,#20605) ;
#16798=AXIS2_PLACEMENT_3D('',#53082,#20607,#20608) ;
#16799=AXIS2_PLACEMENT_3D('',#53083,#20609,#20610) ;
#16800=AXIS2_PLACEMENT_3D('',#53085,#20611,#20612) ;
#16801=AXIS2_PLACEMENT_3D('',#53087,#20613,#20614) ;
#16802=AXIS2_PLACEMENT_3D('',#53088,#20615,#20616) ;
#16803=AXIS2_PLACEMENT_3D('',#53089,#20617,#20618) ;
#16804=AXIS2_PLACEMENT_3D('',#53091,#20619,#20620) ;
#16805=AXIS2_PLACEMENT_3D('',#53093,#20621,#20622) ;
#16806=AXIS2_PLACEMENT_3D('',#53094,#20623,#20624) ;
#16807=AXIS2_PLACEMENT_3D('',#53095,#20625,#20626) ;
#16808=AXIS2_PLACEMENT_3D('',#53097,#20628,#20629) ;
#16809=AXIS2_PLACEMENT_3D('',#53099,#20631,#20632) ;
#16810=AXIS2_PLACEMENT_3D('',#53100,#20633,#20634) ;
#16811=AXIS2_PLACEMENT_3D('',#53102,#20635,#20636) ;
#16812=AXIS2_PLACEMENT_3D('',#53104,#20637,#20638) ;
#16813=AXIS2_PLACEMENT_3D('',#53105,#20639,#20640) ;
#16814=AXIS2_PLACEMENT_3D('',#53106,#20641,#20642) ;
#16815=AXIS2_PLACEMENT_3D('',#53108,#20643,#20644) ;
#16816=AXIS2_PLACEMENT_3D('',#53110,#20645,#20646) ;
#16817=AXIS2_PLACEMENT_3D('',#53111,#20647,#20648) ;
#16818=AXIS2_PLACEMENT_3D('',#53112,#20649,#20650) ;
#16819=AXIS2_PLACEMENT_3D('',#53114,#20652,#20653) ;
#16820=AXIS2_PLACEMENT_3D('',#53116,#20655,#20656) ;
#16821=AXIS2_PLACEMENT_3D('',#53117,#20657,#20658) ;
#16822=AXIS2_PLACEMENT_3D('',#53119,#20659,#20660) ;
#16823=AXIS2_PLACEMENT_3D('',#53121,#20661,#20662) ;
#16824=AXIS2_PLACEMENT_3D('',#53122,#20663,#20664) ;
#16825=AXIS2_PLACEMENT_3D('',#53123,#20665,#20666) ;
#16826=AXIS2_PLACEMENT_3D('',#53125,#20667,#20668) ;
#16827=AXIS2_PLACEMENT_3D('',#53127,#20669,#20670) ;
#16828=AXIS2_PLACEMENT_3D('',#53128,#20671,#20672) ;
#16829=AXIS2_PLACEMENT_3D('',#53129,#20673,#20674) ;
#16830=AXIS2_PLACEMENT_3D('',#53131,#20676,#20677) ;
#16831=AXIS2_PLACEMENT_3D('',#53133,#20679,#20680) ;
#16832=AXIS2_PLACEMENT_3D('',#53134,#20681,#20682) ;
#16833=AXIS2_PLACEMENT_3D('',#53136,#20683,#20684) ;
#16834=AXIS2_PLACEMENT_3D('',#53138,#20685,#20686) ;
#16835=AXIS2_PLACEMENT_3D('',#53139,#20687,#20688) ;
#16836=AXIS2_PLACEMENT_3D('',#53140,#20689,#20690) ;
#16837=AXIS2_PLACEMENT_3D('',#53142,#20691,#20692) ;
#16838=AXIS2_PLACEMENT_3D('',#53144,#20693,#20694) ;
#16839=AXIS2_PLACEMENT_3D('',#53145,#20695,#20696) ;
#16840=AXIS2_PLACEMENT_3D('',#53146,#20697,#20698) ;
#16841=AXIS2_PLACEMENT_3D('',#53148,#20700,#20701) ;
#16842=AXIS2_PLACEMENT_3D('',#53150,#20703,#20704) ;
#16843=AXIS2_PLACEMENT_3D('',#53151,#20705,#20706) ;
#16844=AXIS2_PLACEMENT_3D('',#53153,#20707,#20708) ;
#16845=AXIS2_PLACEMENT_3D('',#53155,#20709,#20710) ;
#16846=AXIS2_PLACEMENT_3D('',#53156,#20711,#20712) ;
#16847=AXIS2_PLACEMENT_3D('',#53157,#20713,#20714) ;
#16848=AXIS2_PLACEMENT_3D('',#53159,#20715,#20716) ;
#16849=AXIS2_PLACEMENT_3D('',#53161,#20717,#20718) ;
#16850=AXIS2_PLACEMENT_3D('',#53162,#20719,#20720) ;
#16851=AXIS2_PLACEMENT_3D('',#53163,#20721,#20722) ;
#16852=AXIS2_PLACEMENT_3D('',#53165,#20724,#20725) ;
#16853=AXIS2_PLACEMENT_3D('',#53167,#20727,#20728) ;
#16854=AXIS2_PLACEMENT_3D('',#53168,#20729,#20730) ;
#16855=AXIS2_PLACEMENT_3D('',#53170,#20731,#20732) ;
#16856=AXIS2_PLACEMENT_3D('',#53172,#20733,#20734) ;
#16857=AXIS2_PLACEMENT_3D('',#53173,#20735,#20736) ;
#16858=AXIS2_PLACEMENT_3D('',#53174,#20737,#20738) ;
#16859=AXIS2_PLACEMENT_3D('',#53176,#20739,#20740) ;
#16860=AXIS2_PLACEMENT_3D('',#53178,#20741,#20742) ;
#16861=AXIS2_PLACEMENT_3D('',#53179,#20743,#20744) ;
#16862=AXIS2_PLACEMENT_3D('',#53180,#20745,#20746) ;
#16863=AXIS2_PLACEMENT_3D('',#53182,#20748,#20749) ;
#16864=AXIS2_PLACEMENT_3D('',#53184,#20751,#20752) ;
#16865=AXIS2_PLACEMENT_3D('',#53185,#20753,#20754) ;
#16866=AXIS2_PLACEMENT_3D('',#53187,#20755,#20756) ;
#16867=AXIS2_PLACEMENT_3D('',#53189,#20757,#20758) ;
#16868=AXIS2_PLACEMENT_3D('',#53190,#20759,#20760) ;
#16869=AXIS2_PLACEMENT_3D('',#53191,#20761,#20762) ;
#16870=AXIS2_PLACEMENT_3D('',#53193,#20763,#20764) ;
#16871=AXIS2_PLACEMENT_3D('',#53195,#20765,#20766) ;
#16872=AXIS2_PLACEMENT_3D('',#53196,#20767,#20768) ;
#16873=AXIS2_PLACEMENT_3D('',#53197,#20769,#20770) ;
#16874=AXIS2_PLACEMENT_3D('',#53199,#20772,#20773) ;
#16875=AXIS2_PLACEMENT_3D('',#53201,#20775,#20776) ;
#16876=AXIS2_PLACEMENT_3D('',#53202,#20777,#20778) ;
#16877=AXIS2_PLACEMENT_3D('',#53204,#20779,#20780) ;
#16878=AXIS2_PLACEMENT_3D('',#53206,#20781,#20782) ;
#16879=AXIS2_PLACEMENT_3D('',#53207,#20783,#20784) ;
#16880=AXIS2_PLACEMENT_3D('',#53208,#20785,#20786) ;
#16881=AXIS2_PLACEMENT_3D('',#53210,#20787,#20788) ;
#16882=AXIS2_PLACEMENT_3D('',#53212,#20789,#20790) ;
#16883=AXIS2_PLACEMENT_3D('',#53213,#20791,#20792) ;
#16884=AXIS2_PLACEMENT_3D('',#53214,#20793,#20794) ;
#16885=AXIS2_PLACEMENT_3D('',#53216,#20796,#20797) ;
#16886=AXIS2_PLACEMENT_3D('',#53218,#20799,#20800) ;
#16887=AXIS2_PLACEMENT_3D('',#53219,#20801,#20802) ;
#16888=AXIS2_PLACEMENT_3D('',#53221,#20803,#20804) ;
#16889=AXIS2_PLACEMENT_3D('',#53223,#20805,#20806) ;
#16890=AXIS2_PLACEMENT_3D('',#53224,#20807,#20808) ;
#16891=AXIS2_PLACEMENT_3D('',#53225,#20809,#20810) ;
#16892=AXIS2_PLACEMENT_3D('',#53227,#20811,#20812) ;
#16893=AXIS2_PLACEMENT_3D('',#53229,#20813,#20814) ;
#16894=AXIS2_PLACEMENT_3D('',#53230,#20815,#20816) ;
#16895=AXIS2_PLACEMENT_3D('',#53231,#20817,#20818) ;
#16896=AXIS2_PLACEMENT_3D('',#53233,#20820,#20821) ;
#16897=AXIS2_PLACEMENT_3D('',#53235,#20823,#20824) ;
#16898=AXIS2_PLACEMENT_3D('',#53236,#20825,#20826) ;
#16899=AXIS2_PLACEMENT_3D('',#53238,#20827,#20828) ;
#16900=AXIS2_PLACEMENT_3D('',#53240,#20829,#20830) ;
#16901=AXIS2_PLACEMENT_3D('',#53241,#20831,#20832) ;
#16902=AXIS2_PLACEMENT_3D('',#53242,#20833,#20834) ;
#16903=AXIS2_PLACEMENT_3D('',#53244,#20835,#20836) ;
#16904=AXIS2_PLACEMENT_3D('',#53246,#20837,#20838) ;
#16905=AXIS2_PLACEMENT_3D('',#53247,#20839,#20840) ;
#16906=AXIS2_PLACEMENT_3D('',#53248,#20841,#20842) ;
#16907=AXIS2_PLACEMENT_3D('',#53250,#20844,#20845) ;
#16908=AXIS2_PLACEMENT_3D('',#53252,#20847,#20848) ;
#16909=AXIS2_PLACEMENT_3D('',#53253,#20849,#20850) ;
#16910=AXIS2_PLACEMENT_3D('',#53255,#20851,#20852) ;
#16911=AXIS2_PLACEMENT_3D('',#53257,#20853,#20854) ;
#16912=AXIS2_PLACEMENT_3D('',#53258,#20855,#20856) ;
#16913=AXIS2_PLACEMENT_3D('',#53259,#20857,#20858) ;
#16914=AXIS2_PLACEMENT_3D('',#53261,#20859,#20860) ;
#16915=AXIS2_PLACEMENT_3D('',#53263,#20861,#20862) ;
#16916=AXIS2_PLACEMENT_3D('',#53264,#20863,#20864) ;
#16917=AXIS2_PLACEMENT_3D('',#53265,#20865,#20866) ;
#16918=AXIS2_PLACEMENT_3D('',#53267,#20868,#20869) ;
#16919=AXIS2_PLACEMENT_3D('',#53269,#20871,#20872) ;
#16920=AXIS2_PLACEMENT_3D('',#53270,#20873,#20874) ;
#16921=AXIS2_PLACEMENT_3D('',#53272,#20875,#20876) ;
#16922=AXIS2_PLACEMENT_3D('',#53274,#20877,#20878) ;
#16923=AXIS2_PLACEMENT_3D('',#53275,#20879,#20880) ;
#16924=AXIS2_PLACEMENT_3D('',#53276,#20881,#20882) ;
#16925=AXIS2_PLACEMENT_3D('',#53278,#20883,#20884) ;
#16926=AXIS2_PLACEMENT_3D('',#53280,#20885,#20886) ;
#16927=AXIS2_PLACEMENT_3D('',#53281,#20887,#20888) ;
#16928=AXIS2_PLACEMENT_3D('',#53282,#20889,#20890) ;
#16929=AXIS2_PLACEMENT_3D('',#53284,#20892,#20893) ;
#16930=AXIS2_PLACEMENT_3D('',#53286,#20895,#20896) ;
#16931=AXIS2_PLACEMENT_3D('',#53287,#20897,#20898) ;
#16932=AXIS2_PLACEMENT_3D('',#53289,#20899,#20900) ;
#16933=AXIS2_PLACEMENT_3D('',#53291,#20901,#20902) ;
#16934=AXIS2_PLACEMENT_3D('',#53292,#20903,#20904) ;
#16935=AXIS2_PLACEMENT_3D('',#53293,#20905,#20906) ;
#16936=AXIS2_PLACEMENT_3D('',#53295,#20907,#20908) ;
#16937=AXIS2_PLACEMENT_3D('',#53297,#20909,#20910) ;
#16938=AXIS2_PLACEMENT_3D('',#53298,#20911,#20912) ;
#16939=AXIS2_PLACEMENT_3D('',#53299,#20913,#20914) ;
#16940=AXIS2_PLACEMENT_3D('',#53301,#20916,#20917) ;
#16941=AXIS2_PLACEMENT_3D('',#53303,#20919,#20920) ;
#16942=AXIS2_PLACEMENT_3D('',#53304,#20921,#20922) ;
#16943=AXIS2_PLACEMENT_3D('',#53306,#20923,#20924) ;
#16944=AXIS2_PLACEMENT_3D('',#53308,#20925,#20926) ;
#16945=AXIS2_PLACEMENT_3D('',#53309,#20927,#20928) ;
#16946=AXIS2_PLACEMENT_3D('',#53310,#20929,#20930) ;
#16947=AXIS2_PLACEMENT_3D('',#53312,#20931,#20932) ;
#16948=AXIS2_PLACEMENT_3D('',#53314,#20933,#20934) ;
#16949=AXIS2_PLACEMENT_3D('',#53315,#20935,#20936) ;
#16950=AXIS2_PLACEMENT_3D('',#53316,#20937,#20938) ;
#16951=AXIS2_PLACEMENT_3D('',#53318,#20940,#20941) ;
#16952=AXIS2_PLACEMENT_3D('',#53320,#20943,#20944) ;
#16953=AXIS2_PLACEMENT_3D('',#53321,#20945,#20946) ;
#16954=AXIS2_PLACEMENT_3D('',#53323,#20947,#20948) ;
#16955=AXIS2_PLACEMENT_3D('',#53325,#20949,#20950) ;
#16956=AXIS2_PLACEMENT_3D('',#53326,#20951,#20952) ;
#16957=AXIS2_PLACEMENT_3D('',#53327,#20953,#20954) ;
#16958=AXIS2_PLACEMENT_3D('',#53329,#20955,#20956) ;
#16959=AXIS2_PLACEMENT_3D('',#53331,#20957,#20958) ;
#16960=AXIS2_PLACEMENT_3D('',#53332,#20959,#20960) ;
#16961=AXIS2_PLACEMENT_3D('',#53333,#20961,#20962) ;
#16962=AXIS2_PLACEMENT_3D('',#53335,#20964,#20965) ;
#16963=AXIS2_PLACEMENT_3D('',#53337,#20967,#20968) ;
#16964=AXIS2_PLACEMENT_3D('',#53338,#20969,#20970) ;
#16965=AXIS2_PLACEMENT_3D('',#53340,#20971,#20972) ;
#16966=AXIS2_PLACEMENT_3D('',#53342,#20973,#20974) ;
#16967=AXIS2_PLACEMENT_3D('',#53343,#20975,#20976) ;
#16968=AXIS2_PLACEMENT_3D('',#53344,#20977,#20978) ;
#16969=AXIS2_PLACEMENT_3D('',#53346,#20979,#20980) ;
#16970=AXIS2_PLACEMENT_3D('',#53348,#20981,#20982) ;
#16971=AXIS2_PLACEMENT_3D('',#53349,#20983,#20984) ;
#16972=AXIS2_PLACEMENT_3D('',#53350,#20985,#20986) ;
#16973=AXIS2_PLACEMENT_3D('',#53352,#20988,#20989) ;
#16974=AXIS2_PLACEMENT_3D('',#53354,#20991,#20992) ;
#16975=AXIS2_PLACEMENT_3D('',#53355,#20993,#20994) ;
#16976=AXIS2_PLACEMENT_3D('',#53357,#20995,#20996) ;
#16977=AXIS2_PLACEMENT_3D('',#53359,#20997,#20998) ;
#16978=AXIS2_PLACEMENT_3D('',#53360,#20999,#21000) ;
#16979=AXIS2_PLACEMENT_3D('',#53361,#21001,#21002) ;
#16980=AXIS2_PLACEMENT_3D('',#53363,#21003,#21004) ;
#16981=AXIS2_PLACEMENT_3D('',#53365,#21005,#21006) ;
#16982=AXIS2_PLACEMENT_3D('',#53366,#21007,#21008) ;
#16983=AXIS2_PLACEMENT_3D('',#53367,#21009,#21010) ;
#16984=AXIS2_PLACEMENT_3D('',#53369,#21012,#21013) ;
#16985=AXIS2_PLACEMENT_3D('',#53371,#21015,#21016) ;
#16986=AXIS2_PLACEMENT_3D('',#53372,#21017,#21018) ;
#16987=AXIS2_PLACEMENT_3D('',#53374,#21019,#21020) ;
#16988=AXIS2_PLACEMENT_3D('',#53376,#21021,#21022) ;
#16989=AXIS2_PLACEMENT_3D('',#53377,#21023,#21024) ;
#16990=AXIS2_PLACEMENT_3D('',#53378,#21025,#21026) ;
#16991=AXIS2_PLACEMENT_3D('',#53380,#21027,#21028) ;
#16992=AXIS2_PLACEMENT_3D('',#53382,#21029,#21030) ;
#16993=AXIS2_PLACEMENT_3D('',#53383,#21031,#21032) ;
#16994=AXIS2_PLACEMENT_3D('',#53384,#21033,#21034) ;
#16995=AXIS2_PLACEMENT_3D('',#53386,#21036,#21037) ;
#16996=AXIS2_PLACEMENT_3D('',#53388,#21039,#21040) ;
#16997=AXIS2_PLACEMENT_3D('',#53389,#21041,#21042) ;
#16998=AXIS2_PLACEMENT_3D('',#53391,#21043,#21044) ;
#16999=AXIS2_PLACEMENT_3D('',#53393,#21045,#21046) ;
#17000=AXIS2_PLACEMENT_3D('',#53394,#21047,#21048) ;
#17001=AXIS2_PLACEMENT_3D('',#53395,#21049,#21050) ;
#17002=AXIS2_PLACEMENT_3D('',#53397,#21051,#21052) ;
#17003=AXIS2_PLACEMENT_3D('',#53399,#21053,#21054) ;
#17004=AXIS2_PLACEMENT_3D('',#53400,#21055,#21056) ;
#17005=AXIS2_PLACEMENT_3D('',#53401,#21057,#21058) ;
#17006=AXIS2_PLACEMENT_3D('',#53403,#21060,#21061) ;
#17007=AXIS2_PLACEMENT_3D('',#53405,#21063,#21064) ;
#17008=AXIS2_PLACEMENT_3D('',#53406,#21065,#21066) ;
#17009=AXIS2_PLACEMENT_3D('',#53408,#21067,#21068) ;
#17010=AXIS2_PLACEMENT_3D('',#53410,#21069,#21070) ;
#17011=AXIS2_PLACEMENT_3D('',#53411,#21071,#21072) ;
#17012=AXIS2_PLACEMENT_3D('',#53412,#21073,#21074) ;
#17013=AXIS2_PLACEMENT_3D('',#53414,#21075,#21076) ;
#17014=AXIS2_PLACEMENT_3D('',#53416,#21077,#21078) ;
#17015=AXIS2_PLACEMENT_3D('',#53417,#21079,#21080) ;
#17016=AXIS2_PLACEMENT_3D('',#53418,#21081,#21082) ;
#17017=AXIS2_PLACEMENT_3D('',#53420,#21084,#21085) ;
#17018=AXIS2_PLACEMENT_3D('',#53422,#21087,#21088) ;
#17019=AXIS2_PLACEMENT_3D('',#53423,#21089,#21090) ;
#17020=AXIS2_PLACEMENT_3D('',#53425,#21091,#21092) ;
#17021=AXIS2_PLACEMENT_3D('',#53427,#21093,#21094) ;
#17022=AXIS2_PLACEMENT_3D('',#53428,#21095,#21096) ;
#17023=AXIS2_PLACEMENT_3D('',#53429,#21097,#21098) ;
#17024=AXIS2_PLACEMENT_3D('',#53431,#21099,#21100) ;
#17025=AXIS2_PLACEMENT_3D('',#53433,#21101,#21102) ;
#17026=AXIS2_PLACEMENT_3D('',#53434,#21103,#21104) ;
#17027=AXIS2_PLACEMENT_3D('',#53435,#21105,#21106) ;
#17028=AXIS2_PLACEMENT_3D('',#53437,#21108,#21109) ;
#17029=AXIS2_PLACEMENT_3D('',#53439,#21111,#21112) ;
#17030=AXIS2_PLACEMENT_3D('',#53440,#21113,#21114) ;
#17031=AXIS2_PLACEMENT_3D('',#53442,#21115,#21116) ;
#17032=AXIS2_PLACEMENT_3D('',#53444,#21117,#21118) ;
#17033=AXIS2_PLACEMENT_3D('',#53445,#21119,#21120) ;
#17034=AXIS2_PLACEMENT_3D('',#53446,#21121,#21122) ;
#17035=AXIS2_PLACEMENT_3D('',#53448,#21123,#21124) ;
#17036=AXIS2_PLACEMENT_3D('',#53450,#21125,#21126) ;
#17037=AXIS2_PLACEMENT_3D('',#53451,#21127,#21128) ;
#17038=AXIS2_PLACEMENT_3D('',#53452,#21129,#21130) ;
#17039=AXIS2_PLACEMENT_3D('',#53454,#21132,#21133) ;
#17040=AXIS2_PLACEMENT_3D('',#53456,#21135,#21136) ;
#17041=AXIS2_PLACEMENT_3D('',#53457,#21137,#21138) ;
#17042=AXIS2_PLACEMENT_3D('',#53459,#21139,#21140) ;
#17043=AXIS2_PLACEMENT_3D('',#53461,#21141,#21142) ;
#17044=AXIS2_PLACEMENT_3D('',#53462,#21143,#21144) ;
#17045=AXIS2_PLACEMENT_3D('',#53463,#21145,#21146) ;
#17046=AXIS2_PLACEMENT_3D('',#53465,#21147,#21148) ;
#17047=AXIS2_PLACEMENT_3D('',#53467,#21149,#21150) ;
#17048=AXIS2_PLACEMENT_3D('',#53468,#21151,#21152) ;
#17049=AXIS2_PLACEMENT_3D('',#53469,#21153,#21154) ;
#17050=AXIS2_PLACEMENT_3D('',#53471,#21156,#21157) ;
#17051=AXIS2_PLACEMENT_3D('',#53473,#21159,#21160) ;
#17052=AXIS2_PLACEMENT_3D('',#53474,#21161,#21162) ;
#17053=AXIS2_PLACEMENT_3D('',#53476,#21163,#21164) ;
#17054=AXIS2_PLACEMENT_3D('',#53478,#21165,#21166) ;
#17055=AXIS2_PLACEMENT_3D('',#53479,#21167,#21168) ;
#17056=AXIS2_PLACEMENT_3D('',#53480,#21169,#21170) ;
#17057=AXIS2_PLACEMENT_3D('',#53482,#21171,#21172) ;
#17058=AXIS2_PLACEMENT_3D('',#53484,#21173,#21174) ;
#17059=AXIS2_PLACEMENT_3D('',#53485,#21175,#21176) ;
#17060=AXIS2_PLACEMENT_3D('',#53486,#21177,#21178) ;
#17061=AXIS2_PLACEMENT_3D('',#53488,#21180,#21181) ;
#17062=AXIS2_PLACEMENT_3D('',#53490,#21183,#21184) ;
#17063=AXIS2_PLACEMENT_3D('',#53491,#21185,#21186) ;
#17064=AXIS2_PLACEMENT_3D('',#53493,#21187,#21188) ;
#17065=AXIS2_PLACEMENT_3D('',#53495,#21189,#21190) ;
#17066=AXIS2_PLACEMENT_3D('',#53496,#21191,#21192) ;
#17067=AXIS2_PLACEMENT_3D('',#53497,#21193,#21194) ;
#17068=AXIS2_PLACEMENT_3D('',#53499,#21195,#21196) ;
#17069=AXIS2_PLACEMENT_3D('',#53501,#21197,#21198) ;
#17070=AXIS2_PLACEMENT_3D('',#53502,#21199,#21200) ;
#17071=AXIS2_PLACEMENT_3D('',#53503,#21201,#21202) ;
#17072=AXIS2_PLACEMENT_3D('',#53505,#21204,#21205) ;
#17073=AXIS2_PLACEMENT_3D('',#53507,#21207,#21208) ;
#17074=AXIS2_PLACEMENT_3D('',#53508,#21209,#21210) ;
#17075=AXIS2_PLACEMENT_3D('',#53510,#21211,#21212) ;
#17076=AXIS2_PLACEMENT_3D('',#53512,#21213,#21214) ;
#17077=AXIS2_PLACEMENT_3D('',#53513,#21215,#21216) ;
#17078=AXIS2_PLACEMENT_3D('',#53514,#21217,#21218) ;
#17079=AXIS2_PLACEMENT_3D('',#53516,#21219,#21220) ;
#17080=AXIS2_PLACEMENT_3D('',#53518,#21221,#21222) ;
#17081=AXIS2_PLACEMENT_3D('',#53519,#21223,#21224) ;
#17082=AXIS2_PLACEMENT_3D('',#53520,#21225,#21226) ;
#17083=AXIS2_PLACEMENT_3D('',#53522,#21228,#21229) ;
#17084=AXIS2_PLACEMENT_3D('',#53524,#21231,#21232) ;
#17085=AXIS2_PLACEMENT_3D('',#53525,#21233,#21234) ;
#17086=AXIS2_PLACEMENT_3D('',#53527,#21235,#21236) ;
#17087=AXIS2_PLACEMENT_3D('',#53529,#21237,#21238) ;
#17088=AXIS2_PLACEMENT_3D('',#53530,#21239,#21240) ;
#17089=AXIS2_PLACEMENT_3D('',#53531,#21241,#21242) ;
#17090=AXIS2_PLACEMENT_3D('',#53533,#21243,#21244) ;
#17091=AXIS2_PLACEMENT_3D('',#53535,#21245,#21246) ;
#17092=AXIS2_PLACEMENT_3D('',#53536,#21247,#21248) ;
#17093=AXIS2_PLACEMENT_3D('',#53537,#21249,#21250) ;
#17094=AXIS2_PLACEMENT_3D('',#53539,#21252,#21253) ;
#17095=AXIS2_PLACEMENT_3D('',#53541,#21255,#21256) ;
#17096=AXIS2_PLACEMENT_3D('',#53542,#21257,#21258) ;
#17097=AXIS2_PLACEMENT_3D('',#53544,#21259,#21260) ;
#17098=AXIS2_PLACEMENT_3D('',#53546,#21261,#21262) ;
#17099=AXIS2_PLACEMENT_3D('',#53547,#21263,#21264) ;
#17100=AXIS2_PLACEMENT_3D('',#53548,#21265,#21266) ;
#17101=AXIS2_PLACEMENT_3D('',#53550,#21267,#21268) ;
#17102=AXIS2_PLACEMENT_3D('',#53552,#21269,#21270) ;
#17103=AXIS2_PLACEMENT_3D('',#53553,#21271,#21272) ;
#17104=AXIS2_PLACEMENT_3D('',#53554,#21273,#21274) ;
#17105=AXIS2_PLACEMENT_3D('',#53556,#21276,#21277) ;
#17106=AXIS2_PLACEMENT_3D('',#53558,#21279,#21280) ;
#17107=AXIS2_PLACEMENT_3D('',#53559,#21281,#21282) ;
#17108=AXIS2_PLACEMENT_3D('',#53561,#21283,#21284) ;
#17109=AXIS2_PLACEMENT_3D('',#53563,#21285,#21286) ;
#17110=AXIS2_PLACEMENT_3D('',#53564,#21287,#21288) ;
#17111=AXIS2_PLACEMENT_3D('',#53565,#21289,#21290) ;
#17112=AXIS2_PLACEMENT_3D('',#53567,#21291,#21292) ;
#17113=AXIS2_PLACEMENT_3D('',#53569,#21293,#21294) ;
#17114=AXIS2_PLACEMENT_3D('',#53570,#21295,#21296) ;
#17115=AXIS2_PLACEMENT_3D('',#53571,#21297,#21298) ;
#17116=AXIS2_PLACEMENT_3D('',#53573,#21300,#21301) ;
#17117=AXIS2_PLACEMENT_3D('',#53575,#21303,#21304) ;
#17118=AXIS2_PLACEMENT_3D('',#53576,#21305,#21306) ;
#17119=AXIS2_PLACEMENT_3D('',#53578,#21307,#21308) ;
#17120=AXIS2_PLACEMENT_3D('',#53580,#21309,#21310) ;
#17121=AXIS2_PLACEMENT_3D('',#53581,#21311,#21312) ;
#17122=AXIS2_PLACEMENT_3D('',#53582,#21313,#21314) ;
#17123=AXIS2_PLACEMENT_3D('',#53584,#21315,#21316) ;
#17124=AXIS2_PLACEMENT_3D('',#53586,#21317,#21318) ;
#17125=AXIS2_PLACEMENT_3D('',#53587,#21319,#21320) ;
#17126=AXIS2_PLACEMENT_3D('',#53588,#21321,#21322) ;
#17127=AXIS2_PLACEMENT_3D('',#53590,#21324,#21325) ;
#17128=AXIS2_PLACEMENT_3D('',#53592,#21327,#21328) ;
#17129=AXIS2_PLACEMENT_3D('',#53593,#21329,#21330) ;
#17130=AXIS2_PLACEMENT_3D('',#53595,#21331,#21332) ;
#17131=AXIS2_PLACEMENT_3D('',#53597,#21333,#21334) ;
#17132=AXIS2_PLACEMENT_3D('',#53598,#21335,#21336) ;
#17133=AXIS2_PLACEMENT_3D('',#53599,#21337,#21338) ;
#17134=AXIS2_PLACEMENT_3D('',#53601,#21339,#21340) ;
#17135=AXIS2_PLACEMENT_3D('',#53603,#21341,#21342) ;
#17136=AXIS2_PLACEMENT_3D('',#53604,#21343,#21344) ;
#17137=AXIS2_PLACEMENT_3D('',#53605,#21345,#21346) ;
#17138=AXIS2_PLACEMENT_3D('',#53607,#21348,#21349) ;
#17139=AXIS2_PLACEMENT_3D('',#53609,#21351,#21352) ;
#17140=AXIS2_PLACEMENT_3D('',#53610,#21353,#21354) ;
#17141=AXIS2_PLACEMENT_3D('',#53612,#21355,#21356) ;
#17142=AXIS2_PLACEMENT_3D('',#53614,#21357,#21358) ;
#17143=AXIS2_PLACEMENT_3D('',#53615,#21359,#21360) ;
#17144=AXIS2_PLACEMENT_3D('',#53616,#21361,#21362) ;
#17145=AXIS2_PLACEMENT_3D('',#53618,#21363,#21364) ;
#17146=AXIS2_PLACEMENT_3D('',#53620,#21365,#21366) ;
#17147=AXIS2_PLACEMENT_3D('',#53621,#21367,#21368) ;
#17148=AXIS2_PLACEMENT_3D('',#53622,#21369,#21370) ;
#17149=AXIS2_PLACEMENT_3D('',#53624,#21372,#21373) ;
#17150=AXIS2_PLACEMENT_3D('',#53626,#21375,#21376) ;
#17151=AXIS2_PLACEMENT_3D('',#53627,#21377,#21378) ;
#17152=AXIS2_PLACEMENT_3D('',#53629,#21379,#21380) ;
#17153=AXIS2_PLACEMENT_3D('',#53631,#21381,#21382) ;
#17154=AXIS2_PLACEMENT_3D('',#53632,#21383,#21384) ;
#17155=AXIS2_PLACEMENT_3D('',#53633,#21385,#21386) ;
#17156=AXIS2_PLACEMENT_3D('',#53635,#21387,#21388) ;
#17157=AXIS2_PLACEMENT_3D('',#53637,#21389,#21390) ;
#17158=AXIS2_PLACEMENT_3D('',#53638,#21391,#21392) ;
#17159=AXIS2_PLACEMENT_3D('',#53639,#21393,#21394) ;
#17160=AXIS2_PLACEMENT_3D('',#53641,#21396,#21397) ;
#17161=AXIS2_PLACEMENT_3D('',#53643,#21399,#21400) ;
#17162=AXIS2_PLACEMENT_3D('',#53644,#21401,#21402) ;
#17163=AXIS2_PLACEMENT_3D('',#53646,#21403,#21404) ;
#17164=AXIS2_PLACEMENT_3D('',#53648,#21405,#21406) ;
#17165=AXIS2_PLACEMENT_3D('',#53649,#21407,#21408) ;
#17166=AXIS2_PLACEMENT_3D('',#53650,#21409,#21410) ;
#17167=AXIS2_PLACEMENT_3D('',#53652,#21411,#21412) ;
#17168=AXIS2_PLACEMENT_3D('',#53654,#21413,#21414) ;
#17169=AXIS2_PLACEMENT_3D('',#53655,#21415,#21416) ;
#17170=AXIS2_PLACEMENT_3D('',#53656,#21417,#21418) ;
#17171=AXIS2_PLACEMENT_3D('',#53658,#21420,#21421) ;
#17172=AXIS2_PLACEMENT_3D('',#53660,#21423,#21424) ;
#17173=AXIS2_PLACEMENT_3D('',#53661,#21425,#21426) ;
#17174=AXIS2_PLACEMENT_3D('',#53663,#21427,#21428) ;
#17175=AXIS2_PLACEMENT_3D('',#53665,#21429,#21430) ;
#17176=AXIS2_PLACEMENT_3D('',#53666,#21431,#21432) ;
#17177=AXIS2_PLACEMENT_3D('',#53667,#21433,#21434) ;
#17178=AXIS2_PLACEMENT_3D('',#53669,#21435,#21436) ;
#17179=AXIS2_PLACEMENT_3D('',#53671,#21437,#21438) ;
#17180=AXIS2_PLACEMENT_3D('',#53672,#21439,#21440) ;
#17181=AXIS2_PLACEMENT_3D('',#53673,#21441,#21442) ;
#17182=AXIS2_PLACEMENT_3D('',#53675,#21444,#21445) ;
#17183=AXIS2_PLACEMENT_3D('',#53677,#21447,#21448) ;
#17184=AXIS2_PLACEMENT_3D('',#53678,#21449,#21450) ;
#17185=AXIS2_PLACEMENT_3D('',#53680,#21451,#21452) ;
#17186=AXIS2_PLACEMENT_3D('',#53682,#21453,#21454) ;
#17187=AXIS2_PLACEMENT_3D('',#53683,#21455,#21456) ;
#17188=AXIS2_PLACEMENT_3D('',#53684,#21457,#21458) ;
#17189=AXIS2_PLACEMENT_3D('',#53686,#21459,#21460) ;
#17190=AXIS2_PLACEMENT_3D('',#53688,#21461,#21462) ;
#17191=AXIS2_PLACEMENT_3D('',#53689,#21463,#21464) ;
#17192=AXIS2_PLACEMENT_3D('',#53690,#21465,#21466) ;
#17193=AXIS2_PLACEMENT_3D('',#53692,#21468,#21469) ;
#17194=AXIS2_PLACEMENT_3D('',#53694,#21471,#21472) ;
#17195=AXIS2_PLACEMENT_3D('',#53695,#21473,#21474) ;
#17196=AXIS2_PLACEMENT_3D('',#53697,#21475,#21476) ;
#17197=AXIS2_PLACEMENT_3D('',#53699,#21477,#21478) ;
#17198=AXIS2_PLACEMENT_3D('',#53700,#21479,#21480) ;
#17199=AXIS2_PLACEMENT_3D('',#53701,#21481,#21482) ;
#17200=AXIS2_PLACEMENT_3D('',#53703,#21483,#21484) ;
#17201=AXIS2_PLACEMENT_3D('',#53705,#21485,#21486) ;
#17202=AXIS2_PLACEMENT_3D('',#53706,#21487,#21488) ;
#17203=AXIS2_PLACEMENT_3D('',#53707,#21489,#21490) ;
#17204=AXIS2_PLACEMENT_3D('',#53709,#21492,#21493) ;
#17205=AXIS2_PLACEMENT_3D('',#53711,#21495,#21496) ;
#17206=AXIS2_PLACEMENT_3D('',#53712,#21497,#21498) ;
#19242=DIRECTION('axis',(0.,0.,1.)) ;
#19243=DIRECTION('refdir',(1.,0.,0.)) ;
#19244=DIRECTION('center_axis',(0.,0.,1.)) ;
#19245=DIRECTION('ref_axis',(0.,-1.,0.)) ;
#19246=DIRECTION('',(1.,0.,0.)) ;
#19247=DIRECTION('',(0.,-1.,0.)) ;
#19248=DIRECTION('',(1.,0.,0.)) ;
#19249=DIRECTION('',(0.,1.,0.)) ;
#19250=DIRECTION('center_axis',(0.,1.,0.)) ;
#19251=DIRECTION('ref_axis',(0.,0.,1.)) ;
#19252=DIRECTION('',(0.,0.,1.)) ;
#19253=DIRECTION('',(1.,0.,0.)) ;
#19254=DIRECTION('',(0.,0.,-1.)) ;
#19255=DIRECTION('center_axis',(0.,0.,-1.)) ;
#19256=DIRECTION('ref_axis',(0.,1.,0.)) ;
#19257=DIRECTION('',(-1.,0.,0.)) ;
#19258=DIRECTION('',(0.,-1.,0.)) ;
#19259=DIRECTION('',(0.,1.,0.)) ;
#19260=DIRECTION('center_axis',(1.,0.,0.)) ;
#19261=DIRECTION('ref_axis',(0.,0.,-1.)) ;
#19262=DIRECTION('center_axis',(1.,0.,0.)) ;
#19263=DIRECTION('ref_axis',(0.,0.,-1.)) ;
#19264=DIRECTION('center_axis',(1.,0.,0.)) ;
#19265=DIRECTION('ref_axis',(0.,0.,-1.)) ;
#19266=DIRECTION('center_axis',(1.,0.,0.)) ;
#19267=DIRECTION('ref_axis',(0.,0.,-1.)) ;
#19268=DIRECTION('',(-1.,0.,0.)) ;
#19269=DIRECTION('center_axis',(1.,0.,0.)) ;
#19270=DIRECTION('ref_axis',(0.,0.,-1.)) ;
#19271=DIRECTION('',(-1.,0.,0.)) ;
#19272=DIRECTION('center_axis',(1.,0.,0.)) ;
#19273=DIRECTION('ref_axis',(0.,0.,-1.)) ;
#19274=DIRECTION('center_axis',(1.,0.,0.)) ;
#19275=DIRECTION('ref_axis',(0.,0.,-1.)) ;
#19276=DIRECTION('center_axis',(1.,0.,0.)) ;
#19277=DIRECTION('ref_axis',(0.,0.,-1.)) ;
#19278=DIRECTION('',(-1.,0.,0.)) ;
#19279=DIRECTION('center_axis',(1.,0.,0.)) ;
#19280=DIRECTION('ref_axis',(0.,0.,-1.)) ;
#19281=DIRECTION('',(-1.,0.,0.)) ;
#19282=DIRECTION('center_axis',(1.,0.,0.)) ;
#19283=DIRECTION('ref_axis',(0.,0.,-1.)) ;
#19284=DIRECTION('center_axis',(1.,0.,0.)) ;
#19285=DIRECTION('ref_axis',(0.,0.,-1.)) ;
#19286=DIRECTION('',(-1.,0.,0.)) ;
#19287=DIRECTION('center_axis',(1.,0.,0.)) ;
#19288=DIRECTION('ref_axis',(0.,0.,-1.)) ;
#19289=DIRECTION('',(-1.,0.,0.)) ;
#19290=DIRECTION('center_axis',(1.,0.,0.)) ;
#19291=DIRECTION('ref_axis',(0.,0.,-1.)) ;
#19292=DIRECTION('center_axis',(1.,0.,0.)) ;
#19293=DIRECTION('ref_axis',(0.,0.,-1.)) ;
#19294=DIRECTION('',(-1.,0.,0.)) ;
#19295=DIRECTION('center_axis',(1.,0.,0.)) ;
#19296=DIRECTION('ref_axis',(0.,0.,-1.)) ;
#19297=DIRECTION('',(-1.,0.,0.)) ;
#19298=DIRECTION('center_axis',(1.,0.,0.)) ;
#19299=DIRECTION('ref_axis',(0.,0.,-1.)) ;
#19300=DIRECTION('',(-1.,0.,0.)) ;
#19301=DIRECTION('center_axis',(1.,0.,0.)) ;
#19302=DIRECTION('ref_axis',(0.,0.,-1.)) ;
#19303=DIRECTION('',(-1.,0.,0.)) ;
#19304=DIRECTION('center_axis',(1.,0.,0.)) ;
#19305=DIRECTION('ref_axis',(0.,0.,-1.)) ;
#19306=DIRECTION('center_axis',(1.,0.,0.)) ;
#19307=DIRECTION('ref_axis',(0.,0.,-1.)) ;
#19308=DIRECTION('',(-1.,0.,0.)) ;
#19309=DIRECTION('center_axis',(1.,0.,0.)) ;
#19310=DIRECTION('ref_axis',(0.,0.,-1.)) ;
#19311=DIRECTION('',(-1.,0.,0.)) ;
#19312=DIRECTION('center_axis',(1.,0.,0.)) ;
#19313=DIRECTION('ref_axis',(0.,0.,-1.)) ;
#19314=DIRECTION('center_axis',(1.,0.,0.)) ;
#19315=DIRECTION('ref_axis',(0.,0.,-1.)) ;
#19316=DIRECTION('',(-1.,0.,0.)) ;
#19317=DIRECTION('center_axis',(1.,0.,0.)) ;
#19318=DIRECTION('ref_axis',(0.,0.,-1.)) ;
#19319=DIRECTION('',(-1.,0.,0.)) ;
#19320=DIRECTION('center_axis',(1.,0.,0.)) ;
#19321=DIRECTION('ref_axis',(0.,0.,-1.)) ;
#19322=DIRECTION('center_axis',(1.,0.,0.)) ;
#19323=DIRECTION('ref_axis',(0.,0.,-1.)) ;
#19324=DIRECTION('center_axis',(1.,0.,0.)) ;
#19325=DIRECTION('ref_axis',(0.,0.,-1.)) ;
#19326=DIRECTION('',(-1.,0.,0.)) ;
#19327=DIRECTION('center_axis',(1.,0.,0.)) ;
#19328=DIRECTION('ref_axis',(0.,0.,-1.)) ;
#19329=DIRECTION('',(-1.,0.,0.)) ;
#19330=DIRECTION('center_axis',(1.,0.,0.)) ;
#19331=DIRECTION('ref_axis',(0.,0.,-1.)) ;
#19332=DIRECTION('center_axis',(1.,0.,0.)) ;
#19333=DIRECTION('ref_axis',(0.,0.,-1.)) ;
#19334=DIRECTION('',(-1.,0.,0.)) ;
#19335=DIRECTION('center_axis',(1.,0.,0.)) ;
#19336=DIRECTION('ref_axis',(0.,0.,-1.)) ;
#19337=DIRECTION('',(-1.,0.,0.)) ;
#19338=DIRECTION('center_axis',(1.,0.,0.)) ;
#19339=DIRECTION('ref_axis',(0.,0.,-1.)) ;
#19340=DIRECTION('center_axis',(1.,0.,0.)) ;
#19341=DIRECTION('ref_axis',(0.,0.,-1.)) ;
#19342=DIRECTION('',(-1.,0.,0.)) ;
#19343=DIRECTION('center_axis',(1.,0.,0.)) ;
#19344=DIRECTION('ref_axis',(0.,0.,-1.)) ;
#19345=DIRECTION('',(-1.,0.,0.)) ;
#19346=DIRECTION('center_axis',(1.,0.,0.)) ;
#19347=DIRECTION('ref_axis',(0.,0.,-1.)) ;
#19348=DIRECTION('center_axis',(1.,0.,0.)) ;
#19349=DIRECTION('ref_axis',(0.,0.,-1.)) ;
#19350=DIRECTION('',(-1.,0.,0.)) ;
#19351=DIRECTION('center_axis',(1.,0.,0.)) ;
#19352=DIRECTION('ref_axis',(0.,0.,-1.)) ;
#19353=DIRECTION('',(-1.,0.,0.)) ;
#19354=DIRECTION('center_axis',(1.,0.,0.)) ;
#19355=DIRECTION('ref_axis',(0.,0.,-1.)) ;
#19356=DIRECTION('center_axis',(1.,0.,0.)) ;
#19357=DIRECTION('ref_axis',(0.,0.,-1.)) ;
#19358=DIRECTION('',(-1.,0.,0.)) ;
#19359=DIRECTION('center_axis',(1.,0.,0.)) ;
#19360=DIRECTION('ref_axis',(0.,0.,-1.)) ;
#19361=DIRECTION('',(-1.,0.,0.)) ;
#19362=DIRECTION('center_axis',(1.,0.,0.)) ;
#19363=DIRECTION('ref_axis',(0.,0.,-1.)) ;
#19364=DIRECTION('center_axis',(1.,0.,0.)) ;
#19365=DIRECTION('ref_axis',(0.,0.,-1.)) ;
#19366=DIRECTION('',(-1.,0.,0.)) ;
#19367=DIRECTION('center_axis',(1.,0.,0.)) ;
#19368=DIRECTION('ref_axis',(0.,0.,-1.)) ;
#19369=DIRECTION('',(-1.,0.,0.)) ;
#19370=DIRECTION('center_axis',(1.,0.,0.)) ;
#19371=DIRECTION('ref_axis',(0.,0.,-1.)) ;
#19372=DIRECTION('center_axis',(1.,0.,0.)) ;
#19373=DIRECTION('ref_axis',(0.,0.,-1.)) ;
#19374=DIRECTION('',(-1.,0.,0.)) ;
#19375=DIRECTION('center_axis',(1.,0.,0.)) ;
#19376=DIRECTION('ref_axis',(0.,0.,-1.)) ;
#19377=DIRECTION('',(-1.,0.,0.)) ;
#19378=DIRECTION('center_axis',(1.,0.,0.)) ;
#19379=DIRECTION('ref_axis',(0.,0.,-1.)) ;
#19380=DIRECTION('center_axis',(1.,0.,0.)) ;
#19381=DIRECTION('ref_axis',(0.,0.,-1.)) ;
#19382=DIRECTION('',(-1.,0.,0.)) ;
#19383=DIRECTION('center_axis',(1.,0.,0.)) ;
#19384=DIRECTION('ref_axis',(0.,0.,-1.)) ;
#19385=DIRECTION('',(-1.,0.,0.)) ;
#19386=DIRECTION('center_axis',(1.,0.,0.)) ;
#19387=DIRECTION('ref_axis',(0.,0.,-1.)) ;
#19388=DIRECTION('center_axis',(1.,0.,0.)) ;
#19389=DIRECTION('ref_axis',(0.,0.,-1.)) ;
#19390=DIRECTION('',(-1.,0.,0.)) ;
#19391=DIRECTION('center_axis',(1.,0.,0.)) ;
#19392=DIRECTION('ref_axis',(0.,0.,-1.)) ;
#19393=DIRECTION('',(-1.,0.,0.)) ;
#19394=DIRECTION('center_axis',(1.,0.,0.)) ;
#19395=DIRECTION('ref_axis',(0.,0.,-1.)) ;
#19396=DIRECTION('center_axis',(1.,0.,0.)) ;
#19397=DIRECTION('ref_axis',(0.,0.,-1.)) ;
#19398=DIRECTION('',(-1.,0.,0.)) ;
#19399=DIRECTION('center_axis',(1.,0.,0.)) ;
#19400=DIRECTION('ref_axis',(0.,0.,-1.)) ;
#19401=DIRECTION('',(-1.,0.,0.)) ;
#19402=DIRECTION('center_axis',(1.,0.,0.)) ;
#19403=DIRECTION('ref_axis',(0.,0.,-1.)) ;
#19404=DIRECTION('center_axis',(1.,0.,0.)) ;
#19405=DIRECTION('ref_axis',(0.,0.,-1.)) ;
#19406=DIRECTION('',(-1.,0.,0.)) ;
#19407=DIRECTION('center_axis',(1.,0.,0.)) ;
#19408=DIRECTION('ref_axis',(0.,0.,-1.)) ;
#19409=DIRECTION('',(-1.,0.,0.)) ;
#19410=DIRECTION('center_axis',(1.,0.,0.)) ;
#19411=DIRECTION('ref_axis',(0.,0.,-1.)) ;
#19412=DIRECTION('center_axis',(1.,0.,0.)) ;
#19413=DIRECTION('ref_axis',(0.,0.,-1.)) ;
#19414=DIRECTION('',(-1.,0.,0.)) ;
#19415=DIRECTION('center_axis',(1.,0.,0.)) ;
#19416=DIRECTION('ref_axis',(0.,0.,-1.)) ;
#19417=DIRECTION('',(-1.,0.,0.)) ;
#19418=DIRECTION('center_axis',(1.,0.,0.)) ;
#19419=DIRECTION('ref_axis',(0.,0.,-1.)) ;
#19420=DIRECTION('center_axis',(1.,0.,0.)) ;
#19421=DIRECTION('ref_axis',(0.,0.,-1.)) ;
#19422=DIRECTION('',(-1.,0.,0.)) ;
#19423=DIRECTION('center_axis',(1.,0.,0.)) ;
#19424=DIRECTION('ref_axis',(0.,0.,-1.)) ;
#19425=DIRECTION('',(-1.,0.,0.)) ;
#19426=DIRECTION('center_axis',(1.,0.,0.)) ;
#19427=DIRECTION('ref_axis',(0.,0.,-1.)) ;
#19428=DIRECTION('',(-1.,0.,0.)) ;
#19429=DIRECTION('center_axis',(1.,0.,0.)) ;
#19430=DIRECTION('ref_axis',(0.,0.,-1.)) ;
#19431=DIRECTION('',(-1.,0.,0.)) ;
#19432=DIRECTION('center_axis',(1.,0.,0.)) ;
#19433=DIRECTION('ref_axis',(0.,0.,-1.)) ;
#19434=DIRECTION('center_axis',(1.,0.,0.)) ;
#19435=DIRECTION('ref_axis',(0.,0.,-1.)) ;
#19436=DIRECTION('center_axis',(1.,0.,0.)) ;
#19437=DIRECTION('ref_axis',(0.,0.,-1.)) ;
#19438=DIRECTION('',(-1.,0.,0.)) ;
#19439=DIRECTION('center_axis',(1.,0.,0.)) ;
#19440=DIRECTION('ref_axis',(0.,0.,-1.)) ;
#19441=DIRECTION('',(-1.,0.,0.)) ;
#19442=DIRECTION('center_axis',(1.,0.,0.)) ;
#19443=DIRECTION('ref_axis',(0.,0.,-1.)) ;
#19444=DIRECTION('center_axis',(1.,0.,0.)) ;
#19445=DIRECTION('ref_axis',(0.,0.,-1.)) ;
#19446=DIRECTION('',(-1.,0.,0.)) ;
#19447=DIRECTION('center_axis',(1.,0.,0.)) ;
#19448=DIRECTION('ref_axis',(0.,0.,-1.)) ;
#19449=DIRECTION('',(-1.,0.,0.)) ;
#19450=DIRECTION('center_axis',(1.,0.,0.)) ;
#19451=DIRECTION('ref_axis',(0.,0.,-1.)) ;
#19452=DIRECTION('center_axis',(1.,0.,0.)) ;
#19453=DIRECTION('ref_axis',(0.,0.,-1.)) ;
#19454=DIRECTION('',(-1.,0.,0.)) ;
#19455=DIRECTION('center_axis',(1.,0.,0.)) ;
#19456=DIRECTION('ref_axis',(0.,0.,-1.)) ;
#19457=DIRECTION('',(-1.,0.,0.)) ;
#19458=DIRECTION('center_axis',(1.,0.,0.)) ;
#19459=DIRECTION('ref_axis',(0.,0.,-1.)) ;
#19460=DIRECTION('center_axis',(1.,0.,0.)) ;
#19461=DIRECTION('ref_axis',(0.,0.,-1.)) ;
#19462=DIRECTION('',(-1.,0.,0.)) ;
#19463=DIRECTION('center_axis',(1.,0.,0.)) ;
#19464=DIRECTION('ref_axis',(0.,0.,-1.)) ;
#19465=DIRECTION('',(-1.,0.,0.)) ;
#19466=DIRECTION('center_axis',(1.,0.,0.)) ;
#19467=DIRECTION('ref_axis',(0.,0.,-1.)) ;
#19468=DIRECTION('center_axis',(1.,0.,0.)) ;
#19469=DIRECTION('ref_axis',(0.,0.,-1.)) ;
#19470=DIRECTION('',(-1.,0.,0.)) ;
#19471=DIRECTION('center_axis',(1.,0.,0.)) ;
#19472=DIRECTION('ref_axis',(0.,0.,-1.)) ;
#19473=DIRECTION('',(-1.,0.,0.)) ;
#19474=DIRECTION('center_axis',(1.,0.,0.)) ;
#19475=DIRECTION('ref_axis',(0.,0.,-1.)) ;
#19476=DIRECTION('center_axis',(1.,0.,0.)) ;
#19477=DIRECTION('ref_axis',(0.,0.,-1.)) ;
#19478=DIRECTION('',(-1.,0.,0.)) ;
#19479=DIRECTION('center_axis',(1.,0.,0.)) ;
#19480=DIRECTION('ref_axis',(0.,0.,-1.)) ;
#19481=DIRECTION('',(-1.,0.,0.)) ;
#19482=DIRECTION('center_axis',(1.,0.,0.)) ;
#19483=DIRECTION('ref_axis',(0.,0.,-1.)) ;
#19484=DIRECTION('center_axis',(1.,0.,0.)) ;
#19485=DIRECTION('ref_axis',(0.,0.,-1.)) ;
#19486=DIRECTION('',(-1.,0.,0.)) ;
#19487=DIRECTION('center_axis',(1.,0.,0.)) ;
#19488=DIRECTION('ref_axis',(0.,0.,-1.)) ;
#19489=DIRECTION('',(-1.,0.,0.)) ;
#19490=DIRECTION('center_axis',(1.,0.,0.)) ;
#19491=DIRECTION('ref_axis',(0.,0.,-1.)) ;
#19492=DIRECTION('center_axis',(1.,0.,0.)) ;
#19493=DIRECTION('ref_axis',(0.,0.,-1.)) ;
#19494=DIRECTION('',(-1.,0.,0.)) ;
#19495=DIRECTION('center_axis',(1.,0.,0.)) ;
#19496=DIRECTION('ref_axis',(0.,0.,-1.)) ;
#19497=DIRECTION('',(-1.,0.,0.)) ;
#19498=DIRECTION('center_axis',(1.,0.,0.)) ;
#19499=DIRECTION('ref_axis',(0.,0.,-1.)) ;
#19500=DIRECTION('center_axis',(1.,0.,0.)) ;
#19501=DIRECTION('ref_axis',(0.,0.,-1.)) ;
#19502=DIRECTION('',(-1.,0.,0.)) ;
#19503=DIRECTION('center_axis',(1.,0.,0.)) ;
#19504=DIRECTION('ref_axis',(0.,0.,-1.)) ;
#19505=DIRECTION('',(-1.,0.,0.)) ;
#19506=DIRECTION('center_axis',(1.,0.,0.)) ;
#19507=DIRECTION('ref_axis',(0.,0.,-1.)) ;
#19508=DIRECTION('center_axis',(1.,0.,0.)) ;
#19509=DIRECTION('ref_axis',(0.,0.,-1.)) ;
#19510=DIRECTION('',(-1.,0.,0.)) ;
#19511=DIRECTION('center_axis',(1.,0.,0.)) ;
#19512=DIRECTION('ref_axis',(0.,0.,-1.)) ;
#19513=DIRECTION('',(-1.,0.,0.)) ;
#19514=DIRECTION('center_axis',(1.,0.,0.)) ;
#19515=DIRECTION('ref_axis',(0.,0.,-1.)) ;
#19516=DIRECTION('center_axis',(1.,0.,0.)) ;
#19517=DIRECTION('ref_axis',(0.,0.,-1.)) ;
#19518=DIRECTION('',(-1.,0.,0.)) ;
#19519=DIRECTION('center_axis',(1.,0.,0.)) ;
#19520=DIRECTION('ref_axis',(0.,0.,-1.)) ;
#19521=DIRECTION('',(-1.,0.,0.)) ;
#19522=DIRECTION('center_axis',(1.,0.,0.)) ;
#19523=DIRECTION('ref_axis',(0.,0.,-1.)) ;
#19524=DIRECTION('',(-1.,0.,0.)) ;
#19525=DIRECTION('center_axis',(1.,0.,0.)) ;
#19526=DIRECTION('ref_axis',(0.,0.,-1.)) ;
#19527=DIRECTION('',(-1.,0.,0.)) ;
#19528=DIRECTION('center_axis',(1.,0.,0.)) ;
#19529=DIRECTION('ref_axis',(0.,0.,-1.)) ;
#19530=DIRECTION('center_axis',(1.,0.,0.)) ;
#19531=DIRECTION('ref_axis',(0.,0.,-1.)) ;
#19532=DIRECTION('',(-1.,0.,0.)) ;
#19533=DIRECTION('center_axis',(1.,0.,0.)) ;
#19534=DIRECTION('ref_axis',(0.,0.,-1.)) ;
#19535=DIRECTION('',(-1.,0.,0.)) ;
#19536=DIRECTION('center_axis',(1.,0.,0.)) ;
#19537=DIRECTION('ref_axis',(0.,0.,-1.)) ;
#19538=DIRECTION('center_axis',(1.,0.,0.)) ;
#19539=DIRECTION('ref_axis',(0.,0.,-1.)) ;
#19540=DIRECTION('',(-1.,0.,0.)) ;
#19541=DIRECTION('center_axis',(1.,0.,0.)) ;
#19542=DIRECTION('ref_axis',(0.,0.,-1.)) ;
#19543=DIRECTION('',(-1.,0.,0.)) ;
#19544=DIRECTION('center_axis',(1.,0.,0.)) ;
#19545=DIRECTION('ref_axis',(0.,0.,-1.)) ;
#19546=DIRECTION('center_axis',(1.,0.,0.)) ;
#19547=DIRECTION('ref_axis',(0.,0.,-1.)) ;
#19548=DIRECTION('',(-1.,0.,0.)) ;
#19549=DIRECTION('center_axis',(1.,0.,0.)) ;
#19550=DIRECTION('ref_axis',(0.,0.,-1.)) ;
#19551=DIRECTION('',(-1.,0.,0.)) ;
#19552=DIRECTION('center_axis',(1.,0.,0.)) ;
#19553=DIRECTION('ref_axis',(0.,0.,-1.)) ;
#19554=DIRECTION('center_axis',(1.,0.,0.)) ;
#19555=DIRECTION('ref_axis',(0.,0.,-1.)) ;
#19556=DIRECTION('',(-1.,0.,0.)) ;
#19557=DIRECTION('center_axis',(1.,0.,0.)) ;
#19558=DIRECTION('ref_axis',(0.,0.,-1.)) ;
#19559=DIRECTION('',(-1.,0.,0.)) ;
#19560=DIRECTION('center_axis',(1.,0.,0.)) ;
#19561=DIRECTION('ref_axis',(0.,0.,-1.)) ;
#19562=DIRECTION('center_axis',(1.,0.,0.)) ;
#19563=DIRECTION('ref_axis',(0.,0.,-1.)) ;
#19564=DIRECTION('',(-1.,0.,0.)) ;
#19565=DIRECTION('center_axis',(1.,0.,0.)) ;
#19566=DIRECTION('ref_axis',(0.,0.,-1.)) ;
#19567=DIRECTION('',(-1.,0.,0.)) ;
#19568=DIRECTION('center_axis',(1.,0.,0.)) ;
#19569=DIRECTION('ref_axis',(0.,0.,-1.)) ;
#19570=DIRECTION('center_axis',(1.,0.,0.)) ;
#19571=DIRECTION('ref_axis',(0.,0.,-1.)) ;
#19572=DIRECTION('',(-1.,0.,0.)) ;
#19573=DIRECTION('center_axis',(1.,0.,0.)) ;
#19574=DIRECTION('ref_axis',(0.,0.,-1.)) ;
#19575=DIRECTION('',(-1.,0.,0.)) ;
#19576=DIRECTION('center_axis',(1.,0.,0.)) ;
#19577=DIRECTION('ref_axis',(0.,0.,-1.)) ;
#19578=DIRECTION('center_axis',(1.,0.,0.)) ;
#19579=DIRECTION('ref_axis',(0.,0.,-1.)) ;
#19580=DIRECTION('center_axis',(1.,0.,0.)) ;
#19581=DIRECTION('ref_axis',(0.,0.,-1.)) ;
#19582=DIRECTION('',(-1.,0.,0.)) ;
#19583=DIRECTION('center_axis',(1.,0.,0.)) ;
#19584=DIRECTION('ref_axis',(0.,0.,-1.)) ;
#19585=DIRECTION('',(-1.,0.,0.)) ;
#19586=DIRECTION('center_axis',(1.,0.,0.)) ;
#19587=DIRECTION('ref_axis',(0.,0.,-1.)) ;
#19588=DIRECTION('center_axis',(1.,0.,0.)) ;
#19589=DIRECTION('ref_axis',(0.,0.,-1.)) ;
#19590=DIRECTION('',(-1.,0.,0.)) ;
#19591=DIRECTION('center_axis',(1.,0.,0.)) ;
#19592=DIRECTION('ref_axis',(0.,0.,-1.)) ;
#19593=DIRECTION('',(-1.,0.,0.)) ;
#19594=DIRECTION('center_axis',(1.,0.,0.)) ;
#19595=DIRECTION('ref_axis',(0.,0.,-1.)) ;
#19596=DIRECTION('center_axis',(1.,0.,0.)) ;
#19597=DIRECTION('ref_axis',(0.,0.,-1.)) ;
#19598=DIRECTION('',(-1.,0.,0.)) ;
#19599=DIRECTION('center_axis',(1.,0.,0.)) ;
#19600=DIRECTION('ref_axis',(0.,0.,-1.)) ;
#19601=DIRECTION('',(-1.,0.,0.)) ;
#19602=DIRECTION('center_axis',(1.,0.,0.)) ;
#19603=DIRECTION('ref_axis',(0.,0.,-1.)) ;
#19604=DIRECTION('center_axis',(1.,0.,0.)) ;
#19605=DIRECTION('ref_axis',(0.,0.,-1.)) ;
#19606=DIRECTION('',(-1.,0.,0.)) ;
#19607=DIRECTION('center_axis',(1.,0.,0.)) ;
#19608=DIRECTION('ref_axis',(0.,0.,-1.)) ;
#19609=DIRECTION('',(-1.,0.,0.)) ;
#19610=DIRECTION('center_axis',(1.,0.,0.)) ;
#19611=DIRECTION('ref_axis',(0.,0.,-1.)) ;
#19612=DIRECTION('center_axis',(1.,0.,0.)) ;
#19613=DIRECTION('ref_axis',(0.,0.,-1.)) ;
#19614=DIRECTION('',(-1.,0.,0.)) ;
#19615=DIRECTION('center_axis',(1.,0.,0.)) ;
#19616=DIRECTION('ref_axis',(0.,0.,-1.)) ;
#19617=DIRECTION('',(-1.,0.,0.)) ;
#19618=DIRECTION('center_axis',(1.,0.,0.)) ;
#19619=DIRECTION('ref_axis',(0.,0.,-1.)) ;
#19620=DIRECTION('center_axis',(1.,0.,0.)) ;
#19621=DIRECTION('ref_axis',(0.,0.,-1.)) ;
#19622=DIRECTION('',(-1.,0.,0.)) ;
#19623=DIRECTION('center_axis',(1.,0.,0.)) ;
#19624=DIRECTION('ref_axis',(0.,0.,-1.)) ;
#19625=DIRECTION('',(-1.,0.,0.)) ;
#19626=DIRECTION('center_axis',(1.,0.,0.)) ;
#19627=DIRECTION('ref_axis',(0.,0.,-1.)) ;
#19628=DIRECTION('center_axis',(1.,0.,0.)) ;
#19629=DIRECTION('ref_axis',(0.,0.,-1.)) ;
#19630=DIRECTION('',(-1.,0.,0.)) ;
#19631=DIRECTION('center_axis',(1.,0.,0.)) ;
#19632=DIRECTION('ref_axis',(0.,0.,-1.)) ;
#19633=DIRECTION('',(-1.,0.,0.)) ;
#19634=DIRECTION('center_axis',(1.,0.,0.)) ;
#19635=DIRECTION('ref_axis',(0.,0.,-1.)) ;
#19636=DIRECTION('center_axis',(1.,0.,0.)) ;
#19637=DIRECTION('ref_axis',(0.,0.,-1.)) ;
#19638=DIRECTION('',(-1.,0.,0.)) ;
#19639=DIRECTION('center_axis',(1.,0.,0.)) ;
#19640=DIRECTION('ref_axis',(0.,0.,-1.)) ;
#19641=DIRECTION('',(-1.,0.,0.)) ;
#19642=DIRECTION('center_axis',(1.,0.,0.)) ;
#19643=DIRECTION('ref_axis',(0.,0.,-1.)) ;
#19644=DIRECTION('center_axis',(1.,0.,0.)) ;
#19645=DIRECTION('ref_axis',(0.,0.,-1.)) ;
#19646=DIRECTION('',(-1.,0.,0.)) ;
#19647=DIRECTION('center_axis',(1.,0.,0.)) ;
#19648=DIRECTION('ref_axis',(0.,0.,-1.)) ;
#19649=DIRECTION('',(-1.,0.,0.)) ;
#19650=DIRECTION('center_axis',(1.,0.,0.)) ;
#19651=DIRECTION('ref_axis',(0.,0.,-1.)) ;
#19652=DIRECTION('center_axis',(1.,0.,0.)) ;
#19653=DIRECTION('ref_axis',(0.,0.,-1.)) ;
#19654=DIRECTION('',(-1.,0.,0.)) ;
#19655=DIRECTION('center_axis',(1.,0.,0.)) ;
#19656=DIRECTION('ref_axis',(0.,0.,-1.)) ;
#19657=DIRECTION('',(-1.,0.,0.)) ;
#19658=DIRECTION('center_axis',(1.,0.,0.)) ;
#19659=DIRECTION('ref_axis',(0.,0.,-1.)) ;
#19660=DIRECTION('center_axis',(1.,0.,0.)) ;
#19661=DIRECTION('ref_axis',(0.,0.,-1.)) ;
#19662=DIRECTION('',(-1.,0.,0.)) ;
#19663=DIRECTION('center_axis',(1.,0.,0.)) ;
#19664=DIRECTION('ref_axis',(0.,0.,-1.)) ;
#19665=DIRECTION('',(-1.,0.,0.)) ;
#19666=DIRECTION('center_axis',(1.,0.,0.)) ;
#19667=DIRECTION('ref_axis',(0.,0.,-1.)) ;
#19668=DIRECTION('',(-1.,0.,0.)) ;
#19669=DIRECTION('center_axis',(1.,0.,0.)) ;
#19670=DIRECTION('ref_axis',(0.,0.,-1.)) ;
#19671=DIRECTION('',(-1.,0.,0.)) ;
#19672=DIRECTION('center_axis',(1.,0.,0.)) ;
#19673=DIRECTION('ref_axis',(0.,0.,-1.)) ;
#19674=DIRECTION('center_axis',(1.,0.,0.)) ;
#19675=DIRECTION('ref_axis',(0.,0.,-1.)) ;
#19676=DIRECTION('center_axis',(1.,0.,0.)) ;
#19677=DIRECTION('ref_axis',(0.,0.,-1.)) ;
#19678=DIRECTION('',(-1.,0.,0.)) ;
#19679=DIRECTION('center_axis',(1.,0.,0.)) ;
#19680=DIRECTION('ref_axis',(0.,0.,-1.)) ;
#19681=DIRECTION('',(-1.,0.,0.)) ;
#19682=DIRECTION('center_axis',(1.,0.,0.)) ;
#19683=DIRECTION('ref_axis',(0.,0.,-1.)) ;
#19684=DIRECTION('center_axis',(1.,0.,0.)) ;
#19685=DIRECTION('ref_axis',(0.,0.,-1.)) ;
#19686=DIRECTION('',(-1.,0.,0.)) ;
#19687=DIRECTION('center_axis',(1.,0.,0.)) ;
#19688=DIRECTION('ref_axis',(0.,0.,-1.)) ;
#19689=DIRECTION('',(-1.,0.,0.)) ;
#19690=DIRECTION('center_axis',(1.,0.,0.)) ;
#19691=DIRECTION('ref_axis',(0.,0.,-1.)) ;
#19692=DIRECTION('center_axis',(1.,0.,0.)) ;
#19693=DIRECTION('ref_axis',(0.,0.,-1.)) ;
#19694=DIRECTION('',(-1.,0.,0.)) ;
#19695=DIRECTION('center_axis',(1.,0.,0.)) ;
#19696=DIRECTION('ref_axis',(0.,0.,-1.)) ;
#19697=DIRECTION('',(-1.,0.,0.)) ;
#19698=DIRECTION('center_axis',(1.,0.,0.)) ;
#19699=DIRECTION('ref_axis',(0.,0.,-1.)) ;
#19700=DIRECTION('center_axis',(1.,0.,0.)) ;
#19701=DIRECTION('ref_axis',(0.,0.,-1.)) ;
#19702=DIRECTION('',(-1.,0.,0.)) ;
#19703=DIRECTION('center_axis',(1.,0.,0.)) ;
#19704=DIRECTION('ref_axis',(0.,0.,-1.)) ;
#19705=DIRECTION('',(-1.,0.,0.)) ;
#19706=DIRECTION('center_axis',(1.,0.,0.)) ;
#19707=DIRECTION('ref_axis',(0.,0.,-1.)) ;
#19708=DIRECTION('center_axis',(1.,0.,0.)) ;
#19709=DIRECTION('ref_axis',(0.,0.,-1.)) ;
#19710=DIRECTION('',(-1.,0.,0.)) ;
#19711=DIRECTION('center_axis',(1.,0.,0.)) ;
#19712=DIRECTION('ref_axis',(0.,0.,-1.)) ;
#19713=DIRECTION('',(-1.,0.,0.)) ;
#19714=DIRECTION('center_axis',(1.,0.,0.)) ;
#19715=DIRECTION('ref_axis',(0.,0.,-1.)) ;
#19716=DIRECTION('center_axis',(1.,0.,0.)) ;
#19717=DIRECTION('ref_axis',(0.,0.,-1.)) ;
#19718=DIRECTION('',(-1.,0.,0.)) ;
#19719=DIRECTION('center_axis',(1.,0.,0.)) ;
#19720=DIRECTION('ref_axis',(0.,0.,-1.)) ;
#19721=DIRECTION('',(-1.,0.,0.)) ;
#19722=DIRECTION('center_axis',(1.,0.,0.)) ;
#19723=DIRECTION('ref_axis',(0.,0.,-1.)) ;
#19724=DIRECTION('center_axis',(1.,0.,0.)) ;
#19725=DIRECTION('ref_axis',(0.,0.,-1.)) ;
#19726=DIRECTION('',(-1.,0.,0.)) ;
#19727=DIRECTION('center_axis',(1.,0.,0.)) ;
#19728=DIRECTION('ref_axis',(0.,0.,-1.)) ;
#19729=DIRECTION('',(-1.,0.,0.)) ;
#19730=DIRECTION('center_axis',(1.,0.,0.)) ;
#19731=DIRECTION('ref_axis',(0.,0.,-1.)) ;
#19732=DIRECTION('',(-1.,0.,0.)) ;
#19733=DIRECTION('center_axis',(1.,0.,0.)) ;
#19734=DIRECTION('ref_axis',(0.,0.,-1.)) ;
#19735=DIRECTION('',(-1.,0.,0.)) ;
#19736=DIRECTION('center_axis',(1.,0.,0.)) ;
#19737=DIRECTION('ref_axis',(0.,0.,-1.)) ;
#19738=DIRECTION('center_axis',(1.,0.,0.)) ;
#19739=DIRECTION('ref_axis',(0.,0.,-1.)) ;
#19740=DIRECTION('center_axis',(1.,0.,0.)) ;
#19741=DIRECTION('ref_axis',(0.,0.,-1.)) ;
#19742=DIRECTION('',(-1.,0.,0.)) ;
#19743=DIRECTION('center_axis',(1.,0.,0.)) ;
#19744=DIRECTION('ref_axis',(0.,0.,-1.)) ;
#19745=DIRECTION('',(-1.,0.,0.)) ;
#19746=DIRECTION('center_axis',(1.,0.,0.)) ;
#19747=DIRECTION('ref_axis',(0.,0.,-1.)) ;
#19748=DIRECTION('center_axis',(1.,0.,0.)) ;
#19749=DIRECTION('ref_axis',(0.,0.,-1.)) ;
#19750=DIRECTION('',(-1.,0.,0.)) ;
#19751=DIRECTION('center_axis',(1.,0.,0.)) ;
#19752=DIRECTION('ref_axis',(0.,0.,-1.)) ;
#19753=DIRECTION('center_axis',(1.,0.,0.)) ;
#19754=DIRECTION('ref_axis',(0.,0.,-1.)) ;
#19755=DIRECTION('center_axis',(-1.,0.,0.)) ;
#19756=DIRECTION('ref_axis',(0.,0.,1.)) ;
#19757=DIRECTION('',(-0.258819045102518,-1.18291797137867E-16,-0.965925826289069)) ;
#19758=DIRECTION('center_axis',(1.,0.,0.)) ;
#19759=DIRECTION('ref_axis',(0.,0.,-1.)) ;
#19760=DIRECTION('center_axis',(1.,0.,0.)) ;
#19761=DIRECTION('ref_axis',(0.,0.,-1.)) ;
#19762=DIRECTION('center_axis',(1.,0.,0.)) ;
#19763=DIRECTION('ref_axis',(0.,0.,-1.)) ;
#19764=DIRECTION('center_axis',(1.,0.,0.)) ;
#19765=DIRECTION('ref_axis',(0.,0.,-1.)) ;
#19766=DIRECTION('center_axis',(1.,0.,0.)) ;
#19767=DIRECTION('ref_axis',(0.,0.,-1.)) ;
#19768=DIRECTION('',(-0.965925826289059,3.16961915143221E-17,-0.258819045102557)) ;
#19769=DIRECTION('center_axis',(-1.,0.,0.)) ;
#19770=DIRECTION('ref_axis',(0.,0.,1.)) ;
#19771=DIRECTION('',(0.258819045102518,1.18291797137867E-16,0.965925826289069)) ;
#19772=DIRECTION('center_axis',(1.,0.,0.)) ;
#19773=DIRECTION('ref_axis',(0.,0.,-1.)) ;
#19774=DIRECTION('center_axis',(1.,0.,0.)) ;
#19775=DIRECTION('ref_axis',(0.,0.,-1.)) ;
#19776=DIRECTION('center_axis',(1.,0.,0.)) ;
#19777=DIRECTION('ref_axis',(0.,0.,-1.)) ;
#19778=DIRECTION('center_axis',(1.,0.,0.)) ;
#19779=DIRECTION('ref_axis',(0.,0.,-1.)) ;
#19780=DIRECTION('center_axis',(1.,0.,0.)) ;
#19781=DIRECTION('ref_axis',(0.,0.,-1.)) ;
#19782=DIRECTION('center_axis',(1.,0.,0.)) ;
#19783=DIRECTION('ref_axis',(0.,0.,-1.)) ;
#19784=DIRECTION('center_axis',(1.,0.,0.)) ;
#19785=DIRECTION('ref_axis',(0.,0.,-1.)) ;
#19786=DIRECTION('center_axis',(1.,0.,0.)) ;
#19787=DIRECTION('ref_axis',(0.,0.,-1.)) ;
#19788=DIRECTION('center_axis',(1.,0.,0.)) ;
#19789=DIRECTION('ref_axis',(0.,0.,-1.)) ;
#19790=DIRECTION('center_axis',(1.,0.,0.)) ;
#19791=DIRECTION('ref_axis',(0.,0.,-1.)) ;
#19792=DIRECTION('center_axis',(1.,0.,0.)) ;
#19793=DIRECTION('ref_axis',(0.,0.,-1.)) ;
#19794=DIRECTION('center_axis',(1.,0.,0.)) ;
#19795=DIRECTION('ref_axis',(0.,0.,-1.)) ;
#19796=DIRECTION('center_axis',(1.,0.,0.)) ;
#19797=DIRECTION('ref_axis',(0.,0.,-1.)) ;
#19798=DIRECTION('center_axis',(1.,0.,0.)) ;
#19799=DIRECTION('ref_axis',(0.,0.,-1.)) ;
#19800=DIRECTION('center_axis',(1.,0.,0.)) ;
#19801=DIRECTION('ref_axis',(0.,0.,-1.)) ;
#19802=DIRECTION('center_axis',(1.,0.,0.)) ;
#19803=DIRECTION('ref_axis',(0.,0.,-1.)) ;
#19804=DIRECTION('center_axis',(1.,0.,0.)) ;
#19805=DIRECTION('ref_axis',(0.,0.,-1.)) ;
#19806=DIRECTION('center_axis',(1.,0.,0.)) ;
#19807=DIRECTION('ref_axis',(0.,0.,-1.)) ;
#19808=DIRECTION('center_axis',(1.,0.,0.)) ;
#19809=DIRECTION('ref_axis',(0.,0.,-1.)) ;
#19810=DIRECTION('center_axis',(1.,0.,0.)) ;
#19811=DIRECTION('ref_axis',(0.,0.,-1.)) ;
#19812=DIRECTION('center_axis',(1.,0.,0.)) ;
#19813=DIRECTION('ref_axis',(0.,0.,-1.)) ;
#19814=DIRECTION('center_axis',(1.,0.,0.)) ;
#19815=DIRECTION('ref_axis',(0.,0.,-1.)) ;
#19816=DIRECTION('center_axis',(1.,0.,0.)) ;
#19817=DIRECTION('ref_axis',(0.,0.,-1.)) ;
#19818=DIRECTION('center_axis',(1.,0.,0.)) ;
#19819=DIRECTION('ref_axis',(0.,0.,-1.)) ;
#19820=DIRECTION('center_axis',(1.,0.,0.)) ;
#19821=DIRECTION('ref_axis',(0.,0.,-1.)) ;
#19822=DIRECTION('center_axis',(1.,0.,0.)) ;
#19823=DIRECTION('ref_axis',(0.,0.,-1.)) ;
#19824=DIRECTION('center_axis',(1.,0.,0.)) ;
#19825=DIRECTION('ref_axis',(0.,0.,-1.)) ;
#19826=DIRECTION('center_axis',(1.,0.,0.)) ;
#19827=DIRECTION('ref_axis',(0.,0.,-1.)) ;
#19828=DIRECTION('center_axis',(1.,0.,0.)) ;
#19829=DIRECTION('ref_axis',(0.,0.,-1.)) ;
#19830=DIRECTION('center_axis',(1.,0.,0.)) ;
#19831=DIRECTION('ref_axis',(0.,0.,-1.)) ;
#19832=DIRECTION('center_axis',(1.,0.,0.)) ;
#19833=DIRECTION('ref_axis',(0.,0.,-1.)) ;
#19834=DIRECTION('center_axis',(1.,0.,0.)) ;
#19835=DIRECTION('ref_axis',(0.,0.,-1.)) ;
#19836=DIRECTION('center_axis',(1.,0.,0.)) ;
#19837=DIRECTION('ref_axis',(0.,0.,-1.)) ;
#19838=DIRECTION('center_axis',(1.,0.,0.)) ;
#19839=DIRECTION('ref_axis',(0.,0.,-1.)) ;
#19840=DIRECTION('center_axis',(1.,0.,0.)) ;
#19841=DIRECTION('ref_axis',(0.,0.,-1.)) ;
#19842=DIRECTION('center_axis',(1.,0.,0.)) ;
#19843=DIRECTION('ref_axis',(0.,0.,-1.)) ;
#19844=DIRECTION('center_axis',(1.,0.,0.)) ;
#19845=DIRECTION('ref_axis',(0.,0.,-1.)) ;
#19846=DIRECTION('center_axis',(1.,0.,0.)) ;
#19847=DIRECTION('ref_axis',(0.,0.,-1.)) ;
#19848=DIRECTION('center_axis',(1.,0.,0.)) ;
#19849=DIRECTION('ref_axis',(0.,0.,-1.)) ;
#19850=DIRECTION('center_axis',(1.,0.,0.)) ;
#19851=DIRECTION('ref_axis',(0.,0.,-1.)) ;
#19852=DIRECTION('center_axis',(1.,0.,0.)) ;
#19853=DIRECTION('ref_axis',(0.,0.,-1.)) ;
#19854=DIRECTION('center_axis',(1.,0.,0.)) ;
#19855=DIRECTION('ref_axis',(0.,0.,-1.)) ;
#19856=DIRECTION('center_axis',(1.,0.,0.)) ;
#19857=DIRECTION('ref_axis',(0.,0.,-1.)) ;
#19858=DIRECTION('center_axis',(1.,0.,0.)) ;
#19859=DIRECTION('ref_axis',(0.,0.,-1.)) ;
#19860=DIRECTION('center_axis',(1.,0.,0.)) ;
#19861=DIRECTION('ref_axis',(0.,0.,-1.)) ;
#19862=DIRECTION('center_axis',(1.,0.,0.)) ;
#19863=DIRECTION('ref_axis',(0.,0.,-1.)) ;
#19864=DIRECTION('center_axis',(1.,0.,0.)) ;
#19865=DIRECTION('ref_axis',(0.,0.,-1.)) ;
#19866=DIRECTION('center_axis',(1.,0.,0.)) ;
#19867=DIRECTION('ref_axis',(0.,0.,-1.)) ;
#19868=DIRECTION('center_axis',(1.,0.,0.)) ;
#19869=DIRECTION('ref_axis',(0.,0.,-1.)) ;
#19870=DIRECTION('center_axis',(1.,0.,0.)) ;
#19871=DIRECTION('ref_axis',(0.,0.,-1.)) ;
#19872=DIRECTION('center_axis',(1.,0.,0.)) ;
#19873=DIRECTION('ref_axis',(0.,0.,-1.)) ;
#19874=DIRECTION('center_axis',(1.,0.,0.)) ;
#19875=DIRECTION('ref_axis',(0.,0.,-1.)) ;
#19876=DIRECTION('center_axis',(1.,0.,0.)) ;
#19877=DIRECTION('ref_axis',(0.,0.,-1.)) ;
#19878=DIRECTION('center_axis',(1.,0.,0.)) ;
#19879=DIRECTION('ref_axis',(0.,0.,-1.)) ;
#19880=DIRECTION('center_axis',(1.,0.,0.)) ;
#19881=DIRECTION('ref_axis',(0.,0.,-1.)) ;
#19882=DIRECTION('center_axis',(1.,0.,0.)) ;
#19883=DIRECTION('ref_axis',(0.,0.,-1.)) ;
#19884=DIRECTION('center_axis',(1.,0.,0.)) ;
#19885=DIRECTION('ref_axis',(0.,0.,-1.)) ;
#19886=DIRECTION('center_axis',(1.,0.,0.)) ;
#19887=DIRECTION('ref_axis',(0.,0.,-1.)) ;
#19888=DIRECTION('center_axis',(1.,0.,0.)) ;
#19889=DIRECTION('ref_axis',(0.,0.,-1.)) ;
#19890=DIRECTION('center_axis',(1.,0.,0.)) ;
#19891=DIRECTION('ref_axis',(0.,0.,-1.)) ;
#19892=DIRECTION('center_axis',(1.,0.,0.)) ;
#19893=DIRECTION('ref_axis',(0.,0.,-1.)) ;
#19894=DIRECTION('center_axis',(1.,0.,0.)) ;
#19895=DIRECTION('ref_axis',(0.,0.,-1.)) ;
#19896=DIRECTION('center_axis',(1.,0.,0.)) ;
#19897=DIRECTION('ref_axis',(0.,0.,-1.)) ;
#19898=DIRECTION('center_axis',(1.,0.,0.)) ;
#19899=DIRECTION('ref_axis',(0.,0.,-1.)) ;
#19900=DIRECTION('',(-0.258819045102518,1.18291797137867E-16,-0.965925826289069)) ;
#19901=DIRECTION('center_axis',(1.,0.,0.)) ;
#19902=DIRECTION('ref_axis',(0.,0.,-1.)) ;
#19903=DIRECTION('center_axis',(1.,0.,0.)) ;
#19904=DIRECTION('ref_axis',(0.,0.,-1.)) ;
#19905=DIRECTION('center_axis',(1.,0.,0.)) ;
#19906=DIRECTION('ref_axis',(0.,0.,-1.)) ;
#19907=DIRECTION('center_axis',(1.,0.,0.)) ;
#19908=DIRECTION('ref_axis',(0.,0.,-1.)) ;
#19909=DIRECTION('center_axis',(1.,0.,0.)) ;
#19910=DIRECTION('ref_axis',(0.,0.,-1.)) ;
#19911=DIRECTION('center_axis',(1.,0.,0.)) ;
#19912=DIRECTION('ref_axis',(0.,0.,-1.)) ;
#19913=DIRECTION('center_axis',(1.,0.,0.)) ;
#19914=DIRECTION('ref_axis',(0.,0.,-1.)) ;
#19915=DIRECTION('center_axis',(1.,0.,0.)) ;
#19916=DIRECTION('ref_axis',(0.,0.,-1.)) ;
#19917=DIRECTION('center_axis',(1.,0.,0.)) ;
#19918=DIRECTION('ref_axis',(0.,0.,-1.)) ;
#19919=DIRECTION('center_axis',(1.,0.,0.)) ;
#19920=DIRECTION('ref_axis',(0.,0.,-1.)) ;
#19921=DIRECTION('center_axis',(1.,0.,0.)) ;
#19922=DIRECTION('ref_axis',(0.,0.,-1.)) ;
#19923=DIRECTION('center_axis',(1.,0.,0.)) ;
#19924=DIRECTION('ref_axis',(0.,0.,-1.)) ;
#19925=DIRECTION('center_axis',(1.,0.,0.)) ;
#19926=DIRECTION('ref_axis',(0.,0.,-1.)) ;
#19927=DIRECTION('center_axis',(1.,0.,0.)) ;
#19928=DIRECTION('ref_axis',(0.,0.,-1.)) ;
#19929=DIRECTION('center_axis',(1.,0.,0.)) ;
#19930=DIRECTION('ref_axis',(0.,0.,-1.)) ;
#19931=DIRECTION('center_axis',(1.,0.,0.)) ;
#19932=DIRECTION('ref_axis',(0.,0.,-1.)) ;
#19933=DIRECTION('center_axis',(1.,0.,0.)) ;
#19934=DIRECTION('ref_axis',(0.,0.,-1.)) ;
#19935=DIRECTION('center_axis',(1.,0.,0.)) ;
#19936=DIRECTION('ref_axis',(0.,0.,-1.)) ;
#19937=DIRECTION('center_axis',(1.,0.,0.)) ;
#19938=DIRECTION('ref_axis',(0.,0.,-1.)) ;
#19939=DIRECTION('center_axis',(1.,0.,0.)) ;
#19940=DIRECTION('ref_axis',(0.,0.,-1.)) ;
#19941=DIRECTION('center_axis',(1.,0.,0.)) ;
#19942=DIRECTION('ref_axis',(0.,0.,-1.)) ;
#19943=DIRECTION('center_axis',(1.,0.,0.)) ;
#19944=DIRECTION('ref_axis',(0.,0.,-1.)) ;
#19945=DIRECTION('center_axis',(1.,0.,0.)) ;
#19946=DIRECTION('ref_axis',(0.,0.,-1.)) ;
#19947=DIRECTION('center_axis',(1.,0.,0.)) ;
#19948=DIRECTION('ref_axis',(0.,0.,-1.)) ;
#19949=DIRECTION('center_axis',(1.,0.,0.)) ;
#19950=DIRECTION('ref_axis',(0.,0.,-1.)) ;
#19951=DIRECTION('center_axis',(1.,0.,0.)) ;
#19952=DIRECTION('ref_axis',(0.,0.,-1.)) ;
#19953=DIRECTION('center_axis',(1.,0.,0.)) ;
#19954=DIRECTION('ref_axis',(0.,0.,-1.)) ;
#19955=DIRECTION('center_axis',(1.,0.,0.)) ;
#19956=DIRECTION('ref_axis',(0.,0.,-1.)) ;
#19957=DIRECTION('center_axis',(1.,0.,0.)) ;
#19958=DIRECTION('ref_axis',(0.,0.,-1.)) ;
#19959=DIRECTION('center_axis',(1.,0.,0.)) ;
#19960=DIRECTION('ref_axis',(0.,0.,-1.)) ;
#19961=DIRECTION('center_axis',(1.,0.,0.)) ;
#19962=DIRECTION('ref_axis',(0.,0.,-1.)) ;
#19963=DIRECTION('center_axis',(1.,0.,0.)) ;
#19964=DIRECTION('ref_axis',(0.,0.,-1.)) ;
#19965=DIRECTION('center_axis',(1.,0.,0.)) ;
#19966=DIRECTION('ref_axis',(0.,0.,-1.)) ;
#19967=DIRECTION('center_axis',(1.,0.,0.)) ;
#19968=DIRECTION('ref_axis',(0.,0.,-1.)) ;
#19969=DIRECTION('center_axis',(1.,0.,0.)) ;
#19970=DIRECTION('ref_axis',(0.,0.,-1.)) ;
#19971=DIRECTION('center_axis',(1.,0.,0.)) ;
#19972=DIRECTION('ref_axis',(0.,0.,-1.)) ;
#19973=DIRECTION('center_axis',(1.,0.,0.)) ;
#19974=DIRECTION('ref_axis',(0.,0.,-1.)) ;
#19975=DIRECTION('center_axis',(1.,0.,0.)) ;
#19976=DIRECTION('ref_axis',(0.,0.,-1.)) ;
#19977=DIRECTION('center_axis',(1.,0.,0.)) ;
#19978=DIRECTION('ref_axis',(0.,0.,-1.)) ;
#19979=DIRECTION('center_axis',(1.,0.,0.)) ;
#19980=DIRECTION('ref_axis',(0.,0.,-1.)) ;
#19981=DIRECTION('center_axis',(1.,0.,0.)) ;
#19982=DIRECTION('ref_axis',(0.,0.,-1.)) ;
#19983=DIRECTION('center_axis',(1.,0.,0.)) ;
#19984=DIRECTION('ref_axis',(0.,0.,-1.)) ;
#19985=DIRECTION('center_axis',(1.,0.,0.)) ;
#19986=DIRECTION('ref_axis',(0.,0.,-1.)) ;
#19987=DIRECTION('center_axis',(1.,0.,0.)) ;
#19988=DIRECTION('ref_axis',(0.,0.,-1.)) ;
#19989=DIRECTION('center_axis',(1.,0.,0.)) ;
#19990=DIRECTION('ref_axis',(0.,0.,-1.)) ;
#19991=DIRECTION('center_axis',(1.,0.,0.)) ;
#19992=DIRECTION('ref_axis',(0.,0.,-1.)) ;
#19993=DIRECTION('center_axis',(1.,0.,0.)) ;
#19994=DIRECTION('ref_axis',(0.,0.,-1.)) ;
#19995=DIRECTION('center_axis',(1.,0.,0.)) ;
#19996=DIRECTION('ref_axis',(0.,0.,-1.)) ;
#19997=DIRECTION('center_axis',(1.,0.,0.)) ;
#19998=DIRECTION('ref_axis',(0.,0.,-1.)) ;
#19999=DIRECTION('center_axis',(1.,0.,0.)) ;
#20000=DIRECTION('ref_axis',(0.,0.,-1.)) ;
#20001=DIRECTION('center_axis',(1.,0.,0.)) ;
#20002=DIRECTION('ref_axis',(0.,0.,-1.)) ;
#20003=DIRECTION('center_axis',(1.,0.,0.)) ;
#20004=DIRECTION('ref_axis',(0.,0.,-1.)) ;
#20005=DIRECTION('center_axis',(1.,0.,0.)) ;
#20006=DIRECTION('ref_axis',(0.,0.,-1.)) ;
#20007=DIRECTION('center_axis',(1.,0.,0.)) ;
#20008=DIRECTION('ref_axis',(0.,0.,-1.)) ;
#20009=DIRECTION('center_axis',(1.,0.,0.)) ;
#20010=DIRECTION('ref_axis',(0.,0.,-1.)) ;
#20011=DIRECTION('center_axis',(1.,0.,0.)) ;
#20012=DIRECTION('ref_axis',(0.,0.,-1.)) ;
#20013=DIRECTION('center_axis',(1.,0.,0.)) ;
#20014=DIRECTION('ref_axis',(0.,0.,-1.)) ;
#20015=DIRECTION('center_axis',(1.,0.,0.)) ;
#20016=DIRECTION('ref_axis',(0.,0.,-1.)) ;
#20017=DIRECTION('center_axis',(1.,0.,0.)) ;
#20018=DIRECTION('ref_axis',(0.,0.,-1.)) ;
#20019=DIRECTION('center_axis',(1.,0.,0.)) ;
#20020=DIRECTION('ref_axis',(0.,0.,-1.)) ;
#20021=DIRECTION('center_axis',(1.,0.,0.)) ;
#20022=DIRECTION('ref_axis',(0.,0.,-1.)) ;
#20023=DIRECTION('center_axis',(-1.,0.,0.)) ;
#20024=DIRECTION('ref_axis',(0.,0.,1.)) ;
#20025=DIRECTION('',(0.965925826289069,3.16961915143174E-17,0.258819045102518)) ;
#20026=DIRECTION('center_axis',(1.,0.,0.)) ;
#20027=DIRECTION('ref_axis',(0.,0.,-1.)) ;
#20028=DIRECTION('center_axis',(1.,0.,0.)) ;
#20029=DIRECTION('ref_axis',(0.,0.,-1.)) ;
#20030=DIRECTION('center_axis',(1.,0.,0.)) ;
#20031=DIRECTION('ref_axis',(0.,0.,-1.)) ;
#20032=DIRECTION('center_axis',(1.,0.,0.)) ;
#20033=DIRECTION('ref_axis',(0.,0.,-1.)) ;
#20034=DIRECTION('',(0.258819045102518,-1.18291797137867E-16,0.965925826289069)) ;
#20035=DIRECTION('center_axis',(-1.,0.,0.)) ;
#20036=DIRECTION('ref_axis',(0.,0.,1.)) ;
#20037=DIRECTION('center_axis',(1.,0.,0.)) ;
#20038=DIRECTION('ref_axis',(0.,0.,-1.)) ;
#20039=DIRECTION('center_axis',(1.,0.,0.)) ;
#20040=DIRECTION('ref_axis',(0.,0.,-1.)) ;
#20041=DIRECTION('center_axis',(1.,0.,0.)) ;
#20042=DIRECTION('ref_axis',(0.,0.,-1.)) ;
#20043=DIRECTION('',(-1.,0.,0.)) ;
#20044=DIRECTION('center_axis',(-1.,0.,0.)) ;
#20045=DIRECTION('ref_axis',(0.,0.,1.)) ;
#20046=DIRECTION('center_axis',(1.,0.,0.)) ;
#20047=DIRECTION('ref_axis',(0.,0.,-1.)) ;
#20048=DIRECTION('center_axis',(1.,0.,0.)) ;
#20049=DIRECTION('ref_axis',(0.,0.,-1.)) ;
#20050=DIRECTION('center_axis',(1.,0.,0.)) ;
#20051=DIRECTION('ref_axis',(0.,0.,-1.)) ;
#20052=DIRECTION('',(-1.,0.,0.)) ;
#20053=DIRECTION('center_axis',(-1.,0.,0.)) ;
#20054=DIRECTION('ref_axis',(0.,0.,1.)) ;
#20055=DIRECTION('center_axis',(1.,0.,0.)) ;
#20056=DIRECTION('ref_axis',(0.,0.,-1.)) ;
#20057=DIRECTION('center_axis',(1.,0.,0.)) ;
#20058=DIRECTION('ref_axis',(0.,0.,-1.)) ;
#20059=DIRECTION('center_axis',(1.,0.,0.)) ;
#20060=DIRECTION('ref_axis',(0.,0.,-1.)) ;
#20061=DIRECTION('center_axis',(1.,0.,0.)) ;
#20062=DIRECTION('ref_axis',(0.,0.,-1.)) ;
#20063=DIRECTION('center_axis',(1.,0.,0.)) ;
#20064=DIRECTION('ref_axis',(0.,0.,-1.)) ;
#20065=DIRECTION('center_axis',(1.,0.,0.)) ;
#20066=DIRECTION('ref_axis',(0.,0.,-1.)) ;
#20067=DIRECTION('center_axis',(1.,0.,0.)) ;
#20068=DIRECTION('ref_axis',(0.,0.,-1.)) ;
#20069=DIRECTION('center_axis',(1.,0.,0.)) ;
#20070=DIRECTION('ref_axis',(0.,0.,-1.)) ;
#20071=DIRECTION('center_axis',(1.,0.,0.)) ;
#20072=DIRECTION('ref_axis',(0.,0.,-1.)) ;
#20073=DIRECTION('center_axis',(-1.,0.,0.)) ;
#20074=DIRECTION('ref_axis',(0.,0.,1.)) ;
#20075=DIRECTION('',(-1.,0.,0.)) ;
#20076=DIRECTION('center_axis',(-1.,0.,0.)) ;
#20077=DIRECTION('ref_axis',(0.,0.,1.)) ;
#20078=DIRECTION('',(-1.,0.,0.)) ;
#20079=DIRECTION('center_axis',(-1.,0.,0.)) ;
#20080=DIRECTION('ref_axis',(0.,0.,1.)) ;
#20081=DIRECTION('center_axis',(1.,0.,0.)) ;
#20082=DIRECTION('ref_axis',(0.,0.104528463267653,-0.994521895368273)) ;
#20083=DIRECTION('center_axis',(1.,0.,0.)) ;
#20084=DIRECTION('ref_axis',(0.,0.104528463267653,-0.994521895368273)) ;
#20085=DIRECTION('center_axis',(1.,0.,0.)) ;
#20086=DIRECTION('ref_axis',(0.,0.104528463267653,-0.994521895368273)) ;
#20087=DIRECTION('center_axis',(1.,0.,0.)) ;
#20088=DIRECTION('ref_axis',(0.,0.104528463267653,-0.994521895368273)) ;
#20089=DIRECTION('center_axis',(1.,0.,0.)) ;
#20090=DIRECTION('ref_axis',(0.,0.104528463267653,-0.994521895368273)) ;
#20091=DIRECTION('center_axis',(1.,0.,0.)) ;
#20092=DIRECTION('ref_axis',(0.,0.104528463267653,-0.994521895368273)) ;
#20093=DIRECTION('center_axis',(1.,0.,0.)) ;
#20094=DIRECTION('ref_axis',(0.,0.104528463267653,-0.994521895368273)) ;
#20095=DIRECTION('center_axis',(1.,0.,0.)) ;
#20096=DIRECTION('ref_axis',(0.,0.104528463267653,-0.994521895368273)) ;
#20097=DIRECTION('center_axis',(-1.,0.,0.)) ;
#20098=DIRECTION('ref_axis',(0.,-0.104528463267653,0.994521895368273)) ;
#20099=DIRECTION('',(-1.,0.,0.)) ;
#20100=DIRECTION('center_axis',(-1.,0.,0.)) ;
#20101=DIRECTION('ref_axis',(0.,-0.104528463267653,0.994521895368273)) ;
#20102=DIRECTION('',(-1.,0.,0.)) ;
#20103=DIRECTION('center_axis',(-1.,0.,0.)) ;
#20104=DIRECTION('ref_axis',(0.,-0.104528463267653,0.994521895368273)) ;
#20105=DIRECTION('center_axis',(1.,0.,0.)) ;
#20106=DIRECTION('ref_axis',(0.,-0.104528463267653,-0.994521895368273)) ;
#20107=DIRECTION('center_axis',(1.,0.,0.)) ;
#20108=DIRECTION('ref_axis',(0.,-0.104528463267653,-0.994521895368273)) ;
#20109=DIRECTION('center_axis',(1.,0.,0.)) ;
#20110=DIRECTION('ref_axis',(0.,-0.104528463267653,-0.994521895368273)) ;
#20111=DIRECTION('center_axis',(1.,0.,0.)) ;
#20112=DIRECTION('ref_axis',(0.,-0.104528463267653,-0.994521895368273)) ;
#20113=DIRECTION('center_axis',(1.,0.,0.)) ;
#20114=DIRECTION('ref_axis',(0.,-0.104528463267653,-0.994521895368273)) ;
#20115=DIRECTION('center_axis',(1.,0.,0.)) ;
#20116=DIRECTION('ref_axis',(0.,-0.104528463267653,-0.994521895368273)) ;
#20117=DIRECTION('center_axis',(1.,0.,0.)) ;
#20118=DIRECTION('ref_axis',(0.,-0.104528463267653,-0.994521895368273)) ;
#20119=DIRECTION('center_axis',(1.,0.,0.)) ;
#20120=DIRECTION('ref_axis',(0.,-0.104528463267653,-0.994521895368273)) ;
#20121=DIRECTION('center_axis',(-1.,0.,0.)) ;
#20122=DIRECTION('ref_axis',(0.,0.104528463267653,0.994521895368273)) ;
#20123=DIRECTION('',(-1.,0.,0.)) ;
#20124=DIRECTION('center_axis',(-1.,0.,0.)) ;
#20125=DIRECTION('ref_axis',(0.,0.104528463267653,0.994521895368273)) ;
#20126=DIRECTION('',(-1.,0.,0.)) ;
#20127=DIRECTION('center_axis',(-1.,0.,0.)) ;
#20128=DIRECTION('ref_axis',(0.,0.104528463267653,0.994521895368273)) ;
#20129=DIRECTION('center_axis',(1.,0.,0.)) ;
#20130=DIRECTION('ref_axis',(0.,-0.207911690817759,-0.978147600733806)) ;
#20131=DIRECTION('center_axis',(1.,0.,0.)) ;
#20132=DIRECTION('ref_axis',(0.,-0.207911690817759,-0.978147600733806)) ;
#20133=DIRECTION('center_axis',(1.,0.,0.)) ;
#20134=DIRECTION('ref_axis',(0.,-0.207911690817759,-0.978147600733806)) ;
#20135=DIRECTION('center_axis',(1.,0.,0.)) ;
#20136=DIRECTION('ref_axis',(0.,-0.207911690817759,-0.978147600733806)) ;
#20137=DIRECTION('center_axis',(1.,0.,0.)) ;
#20138=DIRECTION('ref_axis',(0.,-0.207911690817759,-0.978147600733806)) ;
#20139=DIRECTION('center_axis',(1.,0.,0.)) ;
#20140=DIRECTION('ref_axis',(0.,-0.207911690817759,-0.978147600733806)) ;
#20141=DIRECTION('center_axis',(1.,0.,0.)) ;
#20142=DIRECTION('ref_axis',(0.,-0.207911690817759,-0.978147600733806)) ;
#20143=DIRECTION('center_axis',(1.,0.,0.)) ;
#20144=DIRECTION('ref_axis',(0.,-0.207911690817759,-0.978147600733806)) ;
#20145=DIRECTION('center_axis',(-1.,0.,0.)) ;
#20146=DIRECTION('ref_axis',(0.,0.207911690817759,0.978147600733806)) ;
#20147=DIRECTION('',(-1.,0.,0.)) ;
#20148=DIRECTION('center_axis',(-1.,0.,0.)) ;
#20149=DIRECTION('ref_axis',(0.,0.207911690817759,0.978147600733806)) ;
#20150=DIRECTION('',(-1.,0.,0.)) ;
#20151=DIRECTION('center_axis',(-1.,0.,0.)) ;
#20152=DIRECTION('ref_axis',(0.,0.207911690817759,0.978147600733806)) ;
#20153=DIRECTION('center_axis',(1.,0.,0.)) ;
#20154=DIRECTION('ref_axis',(0.,-0.309016994374947,-0.951056516295154)) ;
#20155=DIRECTION('center_axis',(1.,0.,0.)) ;
#20156=DIRECTION('ref_axis',(0.,-0.309016994374947,-0.951056516295154)) ;
#20157=DIRECTION('center_axis',(1.,0.,0.)) ;
#20158=DIRECTION('ref_axis',(0.,-0.309016994374947,-0.951056516295154)) ;
#20159=DIRECTION('center_axis',(1.,0.,0.)) ;
#20160=DIRECTION('ref_axis',(0.,-0.309016994374947,-0.951056516295154)) ;
#20161=DIRECTION('center_axis',(1.,0.,0.)) ;
#20162=DIRECTION('ref_axis',(0.,-0.309016994374947,-0.951056516295154)) ;
#20163=DIRECTION('center_axis',(1.,0.,0.)) ;
#20164=DIRECTION('ref_axis',(0.,-0.309016994374947,-0.951056516295154)) ;
#20165=DIRECTION('center_axis',(1.,0.,0.)) ;
#20166=DIRECTION('ref_axis',(0.,-0.309016994374947,-0.951056516295154)) ;
#20167=DIRECTION('center_axis',(1.,0.,0.)) ;
#20168=DIRECTION('ref_axis',(0.,-0.309016994374947,-0.951056516295154)) ;
#20169=DIRECTION('center_axis',(-1.,0.,0.)) ;
#20170=DIRECTION('ref_axis',(0.,0.309016994374947,0.951056516295154)) ;
#20171=DIRECTION('',(-1.,0.,0.)) ;
#20172=DIRECTION('center_axis',(-1.,0.,0.)) ;
#20173=DIRECTION('ref_axis',(0.,0.309016994374947,0.951056516295154)) ;
#20174=DIRECTION('',(-1.,0.,0.)) ;
#20175=DIRECTION('center_axis',(-1.,0.,0.)) ;
#20176=DIRECTION('ref_axis',(0.,0.309016994374947,0.951056516295154)) ;
#20177=DIRECTION('center_axis',(1.,0.,0.)) ;
#20178=DIRECTION('ref_axis',(0.,-0.4067366430758,-0.913545457642601)) ;
#20179=DIRECTION('center_axis',(1.,0.,0.)) ;
#20180=DIRECTION('ref_axis',(0.,-0.4067366430758,-0.913545457642601)) ;
#20181=DIRECTION('center_axis',(1.,0.,0.)) ;
#20182=DIRECTION('ref_axis',(0.,-0.4067366430758,-0.913545457642601)) ;
#20183=DIRECTION('center_axis',(1.,0.,0.)) ;
#20184=DIRECTION('ref_axis',(0.,-0.4067366430758,-0.913545457642601)) ;
#20185=DIRECTION('center_axis',(1.,0.,0.)) ;
#20186=DIRECTION('ref_axis',(0.,-0.4067366430758,-0.913545457642601)) ;
#20187=DIRECTION('center_axis',(1.,0.,0.)) ;
#20188=DIRECTION('ref_axis',(0.,-0.4067366430758,-0.913545457642601)) ;
#20189=DIRECTION('center_axis',(1.,0.,0.)) ;
#20190=DIRECTION('ref_axis',(0.,-0.4067366430758,-0.913545457642601)) ;
#20191=DIRECTION('center_axis',(1.,0.,0.)) ;
#20192=DIRECTION('ref_axis',(0.,-0.4067366430758,-0.913545457642601)) ;
#20193=DIRECTION('center_axis',(-1.,0.,0.)) ;
#20194=DIRECTION('ref_axis',(0.,0.4067366430758,0.913545457642601)) ;
#20195=DIRECTION('',(-1.,0.,0.)) ;
#20196=DIRECTION('center_axis',(-1.,0.,0.)) ;
#20197=DIRECTION('ref_axis',(0.,0.4067366430758,0.913545457642601)) ;
#20198=DIRECTION('',(-1.,0.,0.)) ;
#20199=DIRECTION('center_axis',(-1.,0.,0.)) ;
#20200=DIRECTION('ref_axis',(0.,0.4067366430758,0.913545457642601)) ;
#20201=DIRECTION('center_axis',(1.,0.,0.)) ;
#20202=DIRECTION('ref_axis',(0.,-0.5,-0.866025403784439)) ;
#20203=DIRECTION('center_axis',(1.,0.,0.)) ;
#20204=DIRECTION('ref_axis',(0.,-0.5,-0.866025403784439)) ;
#20205=DIRECTION('center_axis',(1.,0.,0.)) ;
#20206=DIRECTION('ref_axis',(0.,-0.5,-0.866025403784439)) ;
#20207=DIRECTION('center_axis',(1.,0.,0.)) ;
#20208=DIRECTION('ref_axis',(0.,-0.5,-0.866025403784439)) ;
#20209=DIRECTION('center_axis',(1.,0.,0.)) ;
#20210=DIRECTION('ref_axis',(0.,-0.5,-0.866025403784439)) ;
#20211=DIRECTION('center_axis',(1.,0.,0.)) ;
#20212=DIRECTION('ref_axis',(0.,-0.5,-0.866025403784439)) ;
#20213=DIRECTION('center_axis',(1.,0.,0.)) ;
#20214=DIRECTION('ref_axis',(0.,-0.5,-0.866025403784439)) ;
#20215=DIRECTION('center_axis',(1.,0.,0.)) ;
#20216=DIRECTION('ref_axis',(0.,-0.5,-0.866025403784439)) ;
#20217=DIRECTION('center_axis',(-1.,0.,0.)) ;
#20218=DIRECTION('ref_axis',(0.,0.5,0.866025403784439)) ;
#20219=DIRECTION('',(-1.,0.,0.)) ;
#20220=DIRECTION('center_axis',(-1.,0.,0.)) ;
#20221=DIRECTION('ref_axis',(0.,0.5,0.866025403784439)) ;
#20222=DIRECTION('',(-1.,0.,0.)) ;
#20223=DIRECTION('center_axis',(-1.,0.,0.)) ;
#20224=DIRECTION('ref_axis',(0.,0.5,0.866025403784439)) ;
#20225=DIRECTION('center_axis',(1.,0.,0.)) ;
#20226=DIRECTION('ref_axis',(0.,-0.587785252292473,-0.809016994374947)) ;
#20227=DIRECTION('center_axis',(1.,0.,0.)) ;
#20228=DIRECTION('ref_axis',(0.,-0.587785252292473,-0.809016994374947)) ;
#20229=DIRECTION('center_axis',(1.,0.,0.)) ;
#20230=DIRECTION('ref_axis',(0.,-0.587785252292473,-0.809016994374947)) ;
#20231=DIRECTION('center_axis',(1.,0.,0.)) ;
#20232=DIRECTION('ref_axis',(0.,-0.587785252292473,-0.809016994374947)) ;
#20233=DIRECTION('center_axis',(1.,0.,0.)) ;
#20234=DIRECTION('ref_axis',(0.,-0.587785252292473,-0.809016994374947)) ;
#20235=DIRECTION('center_axis',(1.,0.,0.)) ;
#20236=DIRECTION('ref_axis',(0.,-0.587785252292473,-0.809016994374947)) ;
#20237=DIRECTION('center_axis',(1.,0.,0.)) ;
#20238=DIRECTION('ref_axis',(0.,-0.587785252292473,-0.809016994374947)) ;
#20239=DIRECTION('center_axis',(1.,0.,0.)) ;
#20240=DIRECTION('ref_axis',(0.,-0.587785252292473,-0.809016994374947)) ;
#20241=DIRECTION('center_axis',(-1.,0.,0.)) ;
#20242=DIRECTION('ref_axis',(0.,0.587785252292473,0.809016994374947)) ;
#20243=DIRECTION('',(-1.,0.,0.)) ;
#20244=DIRECTION('center_axis',(-1.,0.,0.)) ;
#20245=DIRECTION('ref_axis',(0.,0.587785252292473,0.809016994374947)) ;
#20246=DIRECTION('',(-1.,0.,0.)) ;
#20247=DIRECTION('center_axis',(-1.,0.,0.)) ;
#20248=DIRECTION('ref_axis',(0.,0.587785252292473,0.809016994374947)) ;
#20249=DIRECTION('center_axis',(1.,0.,0.)) ;
#20250=DIRECTION('ref_axis',(0.,-0.743144825477394,-0.669130606358858)) ;
#20251=DIRECTION('center_axis',(1.,0.,0.)) ;
#20252=DIRECTION('ref_axis',(0.,-0.743144825477394,-0.669130606358858)) ;
#20253=DIRECTION('center_axis',(1.,0.,0.)) ;
#20254=DIRECTION('ref_axis',(0.,-0.743144825477394,-0.669130606358858)) ;
#20255=DIRECTION('center_axis',(1.,0.,0.)) ;
#20256=DIRECTION('ref_axis',(0.,-0.743144825477394,-0.669130606358858)) ;
#20257=DIRECTION('center_axis',(1.,0.,0.)) ;
#20258=DIRECTION('ref_axis',(0.,-0.743144825477394,-0.669130606358858)) ;
#20259=DIRECTION('center_axis',(1.,0.,0.)) ;
#20260=DIRECTION('ref_axis',(0.,-0.743144825477394,-0.669130606358858)) ;
#20261=DIRECTION('center_axis',(1.,0.,0.)) ;
#20262=DIRECTION('ref_axis',(0.,-0.743144825477394,-0.669130606358858)) ;
#20263=DIRECTION('center_axis',(1.,0.,0.)) ;
#20264=DIRECTION('ref_axis',(0.,-0.743144825477394,-0.669130606358858)) ;
#20265=DIRECTION('center_axis',(-1.,0.,0.)) ;
#20266=DIRECTION('ref_axis',(0.,0.743144825477394,0.669130606358858)) ;
#20267=DIRECTION('',(-1.,0.,0.)) ;
#20268=DIRECTION('center_axis',(-1.,0.,0.)) ;
#20269=DIRECTION('ref_axis',(0.,0.743144825477394,0.669130606358858)) ;
#20270=DIRECTION('',(-1.,0.,0.)) ;
#20271=DIRECTION('center_axis',(-1.,0.,0.)) ;
#20272=DIRECTION('ref_axis',(0.,0.743144825477394,0.669130606358858)) ;
#20273=DIRECTION('center_axis',(1.,0.,0.)) ;
#20274=DIRECTION('ref_axis',(0.,-0.669130606358858,-0.743144825477394)) ;
#20275=DIRECTION('center_axis',(1.,0.,0.)) ;
#20276=DIRECTION('ref_axis',(0.,-0.669130606358858,-0.743144825477394)) ;
#20277=DIRECTION('center_axis',(1.,0.,0.)) ;
#20278=DIRECTION('ref_axis',(0.,-0.669130606358858,-0.743144825477394)) ;
#20279=DIRECTION('center_axis',(1.,0.,0.)) ;
#20280=DIRECTION('ref_axis',(0.,-0.669130606358858,-0.743144825477394)) ;
#20281=DIRECTION('center_axis',(1.,0.,0.)) ;
#20282=DIRECTION('ref_axis',(0.,-0.669130606358858,-0.743144825477394)) ;
#20283=DIRECTION('center_axis',(1.,0.,0.)) ;
#20284=DIRECTION('ref_axis',(0.,-0.669130606358858,-0.743144825477394)) ;
#20285=DIRECTION('center_axis',(1.,0.,0.)) ;
#20286=DIRECTION('ref_axis',(0.,-0.669130606358858,-0.743144825477394)) ;
#20287=DIRECTION('center_axis',(1.,0.,0.)) ;
#20288=DIRECTION('ref_axis',(0.,-0.669130606358858,-0.743144825477394)) ;
#20289=DIRECTION('center_axis',(-1.,0.,0.)) ;
#20290=DIRECTION('ref_axis',(0.,0.669130606358858,0.743144825477394)) ;
#20291=DIRECTION('',(-1.,0.,0.)) ;
#20292=DIRECTION('center_axis',(-1.,0.,0.)) ;
#20293=DIRECTION('ref_axis',(0.,0.669130606358858,0.743144825477394)) ;
#20294=DIRECTION('',(-1.,0.,0.)) ;
#20295=DIRECTION('center_axis',(-1.,0.,0.)) ;
#20296=DIRECTION('ref_axis',(0.,0.669130606358858,0.743144825477394)) ;
#20297=DIRECTION('center_axis',(1.,0.,0.)) ;
#20298=DIRECTION('ref_axis',(0.,-0.809016994374947,-0.587785252292473)) ;
#20299=DIRECTION('center_axis',(1.,0.,0.)) ;
#20300=DIRECTION('ref_axis',(0.,-0.809016994374947,-0.587785252292473)) ;
#20301=DIRECTION('center_axis',(1.,0.,0.)) ;
#20302=DIRECTION('ref_axis',(0.,-0.809016994374947,-0.587785252292473)) ;
#20303=DIRECTION('center_axis',(1.,0.,0.)) ;
#20304=DIRECTION('ref_axis',(0.,-0.809016994374947,-0.587785252292473)) ;
#20305=DIRECTION('center_axis',(1.,0.,0.)) ;
#20306=DIRECTION('ref_axis',(0.,-0.809016994374947,-0.587785252292473)) ;
#20307=DIRECTION('center_axis',(1.,0.,0.)) ;
#20308=DIRECTION('ref_axis',(0.,-0.809016994374947,-0.587785252292473)) ;
#20309=DIRECTION('center_axis',(1.,0.,0.)) ;
#20310=DIRECTION('ref_axis',(0.,-0.809016994374947,-0.587785252292473)) ;
#20311=DIRECTION('center_axis',(1.,0.,0.)) ;
#20312=DIRECTION('ref_axis',(0.,-0.809016994374947,-0.587785252292473)) ;
#20313=DIRECTION('center_axis',(-1.,0.,0.)) ;
#20314=DIRECTION('ref_axis',(0.,0.809016994374947,0.587785252292473)) ;
#20315=DIRECTION('',(-1.,0.,0.)) ;
#20316=DIRECTION('center_axis',(-1.,0.,0.)) ;
#20317=DIRECTION('ref_axis',(0.,0.809016994374947,0.587785252292473)) ;
#20318=DIRECTION('',(-1.,0.,0.)) ;
#20319=DIRECTION('center_axis',(-1.,0.,0.)) ;
#20320=DIRECTION('ref_axis',(0.,0.809016994374947,0.587785252292473)) ;
#20321=DIRECTION('center_axis',(1.,0.,0.)) ;
#20322=DIRECTION('ref_axis',(0.,-0.866025403784439,-0.5)) ;
#20323=DIRECTION('center_axis',(1.,0.,0.)) ;
#20324=DIRECTION('ref_axis',(0.,-0.866025403784439,-0.5)) ;
#20325=DIRECTION('center_axis',(1.,0.,0.)) ;
#20326=DIRECTION('ref_axis',(0.,-0.866025403784439,-0.5)) ;
#20327=DIRECTION('center_axis',(1.,0.,0.)) ;
#20328=DIRECTION('ref_axis',(0.,-0.866025403784439,-0.5)) ;
#20329=DIRECTION('center_axis',(1.,0.,0.)) ;
#20330=DIRECTION('ref_axis',(0.,-0.866025403784439,-0.5)) ;
#20331=DIRECTION('center_axis',(1.,0.,0.)) ;
#20332=DIRECTION('ref_axis',(0.,-0.866025403784439,-0.5)) ;
#20333=DIRECTION('center_axis',(1.,0.,0.)) ;
#20334=DIRECTION('ref_axis',(0.,-0.866025403784439,-0.5)) ;
#20335=DIRECTION('center_axis',(1.,0.,0.)) ;
#20336=DIRECTION('ref_axis',(0.,-0.866025403784439,-0.5)) ;
#20337=DIRECTION('center_axis',(-1.,0.,0.)) ;
#20338=DIRECTION('ref_axis',(0.,0.866025403784439,0.5)) ;
#20339=DIRECTION('',(-1.,0.,0.)) ;
#20340=DIRECTION('center_axis',(-1.,0.,0.)) ;
#20341=DIRECTION('ref_axis',(0.,0.866025403784439,0.5)) ;
#20342=DIRECTION('',(-1.,0.,0.)) ;
#20343=DIRECTION('center_axis',(-1.,0.,0.)) ;
#20344=DIRECTION('ref_axis',(0.,0.866025403784439,0.5)) ;
#20345=DIRECTION('center_axis',(1.,0.,0.)) ;
#20346=DIRECTION('ref_axis',(0.,-0.913545457642601,-0.4067366430758)) ;
#20347=DIRECTION('center_axis',(1.,0.,0.)) ;
#20348=DIRECTION('ref_axis',(0.,-0.913545457642601,-0.4067366430758)) ;
#20349=DIRECTION('center_axis',(1.,0.,0.)) ;
#20350=DIRECTION('ref_axis',(0.,-0.913545457642601,-0.4067366430758)) ;
#20351=DIRECTION('center_axis',(1.,0.,0.)) ;
#20352=DIRECTION('ref_axis',(0.,-0.913545457642601,-0.4067366430758)) ;
#20353=DIRECTION('center_axis',(1.,0.,0.)) ;
#20354=DIRECTION('ref_axis',(0.,-0.913545457642601,-0.4067366430758)) ;
#20355=DIRECTION('center_axis',(1.,0.,0.)) ;
#20356=DIRECTION('ref_axis',(0.,-0.913545457642601,-0.4067366430758)) ;
#20357=DIRECTION('center_axis',(1.,0.,0.)) ;
#20358=DIRECTION('ref_axis',(0.,-0.913545457642601,-0.4067366430758)) ;
#20359=DIRECTION('center_axis',(1.,0.,0.)) ;
#20360=DIRECTION('ref_axis',(0.,-0.913545457642601,-0.4067366430758)) ;
#20361=DIRECTION('center_axis',(-1.,0.,0.)) ;
#20362=DIRECTION('ref_axis',(0.,0.913545457642601,0.4067366430758)) ;
#20363=DIRECTION('',(-1.,0.,0.)) ;
#20364=DIRECTION('center_axis',(-1.,0.,0.)) ;
#20365=DIRECTION('ref_axis',(0.,0.913545457642601,0.4067366430758)) ;
#20366=DIRECTION('',(-1.,0.,0.)) ;
#20367=DIRECTION('center_axis',(-1.,0.,0.)) ;
#20368=DIRECTION('ref_axis',(0.,0.913545457642601,0.4067366430758)) ;
#20369=DIRECTION('center_axis',(1.,0.,0.)) ;
#20370=DIRECTION('ref_axis',(0.,-0.951056516295154,-0.309016994374947)) ;
#20371=DIRECTION('center_axis',(1.,0.,0.)) ;
#20372=DIRECTION('ref_axis',(0.,-0.951056516295154,-0.309016994374947)) ;
#20373=DIRECTION('center_axis',(1.,0.,0.)) ;
#20374=DIRECTION('ref_axis',(0.,-0.951056516295154,-0.309016994374947)) ;
#20375=DIRECTION('center_axis',(1.,0.,0.)) ;
#20376=DIRECTION('ref_axis',(0.,-0.951056516295154,-0.309016994374947)) ;
#20377=DIRECTION('center_axis',(1.,0.,0.)) ;
#20378=DIRECTION('ref_axis',(0.,-0.951056516295154,-0.309016994374947)) ;
#20379=DIRECTION('center_axis',(1.,0.,0.)) ;
#20380=DIRECTION('ref_axis',(0.,-0.951056516295154,-0.309016994374947)) ;
#20381=DIRECTION('center_axis',(1.,0.,0.)) ;
#20382=DIRECTION('ref_axis',(0.,-0.951056516295154,-0.309016994374947)) ;
#20383=DIRECTION('center_axis',(1.,0.,0.)) ;
#20384=DIRECTION('ref_axis',(0.,-0.951056516295154,-0.309016994374947)) ;
#20385=DIRECTION('center_axis',(-1.,0.,0.)) ;
#20386=DIRECTION('ref_axis',(0.,0.951056516295154,0.309016994374947)) ;
#20387=DIRECTION('',(-1.,0.,0.)) ;
#20388=DIRECTION('center_axis',(-1.,0.,0.)) ;
#20389=DIRECTION('ref_axis',(0.,0.951056516295154,0.309016994374947)) ;
#20390=DIRECTION('',(-1.,0.,0.)) ;
#20391=DIRECTION('center_axis',(-1.,0.,0.)) ;
#20392=DIRECTION('ref_axis',(0.,0.951056516295154,0.309016994374947)) ;
#20393=DIRECTION('center_axis',(1.,0.,0.)) ;
#20394=DIRECTION('ref_axis',(0.,-0.978147600733806,-0.207911690817759)) ;
#20395=DIRECTION('center_axis',(1.,0.,0.)) ;
#20396=DIRECTION('ref_axis',(0.,-0.978147600733806,-0.207911690817759)) ;
#20397=DIRECTION('center_axis',(1.,0.,0.)) ;
#20398=DIRECTION('ref_axis',(0.,-0.978147600733806,-0.207911690817759)) ;
#20399=DIRECTION('center_axis',(1.,0.,0.)) ;
#20400=DIRECTION('ref_axis',(0.,-0.978147600733806,-0.207911690817759)) ;
#20401=DIRECTION('center_axis',(1.,0.,0.)) ;
#20402=DIRECTION('ref_axis',(0.,-0.978147600733806,-0.207911690817759)) ;
#20403=DIRECTION('center_axis',(1.,0.,0.)) ;
#20404=DIRECTION('ref_axis',(0.,-0.978147600733806,-0.207911690817759)) ;
#20405=DIRECTION('center_axis',(1.,0.,0.)) ;
#20406=DIRECTION('ref_axis',(0.,-0.978147600733806,-0.207911690817759)) ;
#20407=DIRECTION('center_axis',(1.,0.,0.)) ;
#20408=DIRECTION('ref_axis',(0.,-0.978147600733806,-0.207911690817759)) ;
#20409=DIRECTION('center_axis',(-1.,0.,0.)) ;
#20410=DIRECTION('ref_axis',(0.,0.978147600733806,0.207911690817759)) ;
#20411=DIRECTION('',(-1.,0.,0.)) ;
#20412=DIRECTION('center_axis',(-1.,0.,0.)) ;
#20413=DIRECTION('ref_axis',(0.,0.978147600733806,0.207911690817759)) ;
#20414=DIRECTION('',(-1.,0.,0.)) ;
#20415=DIRECTION('center_axis',(-1.,0.,0.)) ;
#20416=DIRECTION('ref_axis',(0.,0.978147600733806,0.207911690817759)) ;
#20417=DIRECTION('center_axis',(1.,0.,0.)) ;
#20418=DIRECTION('ref_axis',(0.,-0.994521895368273,-0.104528463267653)) ;
#20419=DIRECTION('center_axis',(1.,0.,0.)) ;
#20420=DIRECTION('ref_axis',(0.,-0.994521895368273,-0.104528463267653)) ;
#20421=DIRECTION('center_axis',(1.,0.,0.)) ;
#20422=DIRECTION('ref_axis',(0.,-0.994521895368273,-0.104528463267653)) ;
#20423=DIRECTION('center_axis',(1.,0.,0.)) ;
#20424=DIRECTION('ref_axis',(0.,-0.994521895368273,-0.104528463267653)) ;
#20425=DIRECTION('center_axis',(1.,0.,0.)) ;
#20426=DIRECTION('ref_axis',(0.,-0.994521895368273,-0.104528463267653)) ;
#20427=DIRECTION('center_axis',(1.,0.,0.)) ;
#20428=DIRECTION('ref_axis',(0.,-0.994521895368273,-0.104528463267653)) ;
#20429=DIRECTION('center_axis',(1.,0.,0.)) ;
#20430=DIRECTION('ref_axis',(0.,-0.994521895368273,-0.104528463267653)) ;
#20431=DIRECTION('center_axis',(1.,0.,0.)) ;
#20432=DIRECTION('ref_axis',(0.,-0.994521895368273,-0.104528463267653)) ;
#20433=DIRECTION('center_axis',(-1.,0.,0.)) ;
#20434=DIRECTION('ref_axis',(0.,0.994521895368273,0.104528463267653)) ;
#20435=DIRECTION('',(-1.,0.,0.)) ;
#20436=DIRECTION('center_axis',(-1.,0.,0.)) ;
#20437=DIRECTION('ref_axis',(0.,0.994521895368273,0.104528463267653)) ;
#20438=DIRECTION('',(-1.,0.,0.)) ;
#20439=DIRECTION('center_axis',(-1.,0.,0.)) ;
#20440=DIRECTION('ref_axis',(0.,0.994521895368273,0.104528463267653)) ;
#20441=DIRECTION('center_axis',(1.,0.,0.)) ;
#20442=DIRECTION('ref_axis',(0.,-1.,1.83697019872103E-16)) ;
#20443=DIRECTION('center_axis',(1.,0.,0.)) ;
#20444=DIRECTION('ref_axis',(0.,-1.,1.83697019872103E-16)) ;
#20445=DIRECTION('center_axis',(1.,0.,0.)) ;
#20446=DIRECTION('ref_axis',(0.,-1.,1.83697019872103E-16)) ;
#20447=DIRECTION('center_axis',(1.,0.,0.)) ;
#20448=DIRECTION('ref_axis',(0.,-1.,1.83697019872103E-16)) ;
#20449=DIRECTION('center_axis',(1.,0.,0.)) ;
#20450=DIRECTION('ref_axis',(0.,-1.,1.83697019872103E-16)) ;
#20451=DIRECTION('center_axis',(1.,0.,0.)) ;
#20452=DIRECTION('ref_axis',(0.,-1.,1.83697019872103E-16)) ;
#20453=DIRECTION('center_axis',(1.,0.,0.)) ;
#20454=DIRECTION('ref_axis',(0.,-1.,1.83697019872103E-16)) ;
#20455=DIRECTION('center_axis',(1.,0.,0.)) ;
#20456=DIRECTION('ref_axis',(0.,-1.,1.83697019872103E-16)) ;
#20457=DIRECTION('center_axis',(-1.,0.,0.)) ;
#20458=DIRECTION('ref_axis',(0.,1.,-1.83697019872103E-16)) ;
#20459=DIRECTION('',(-1.,0.,0.)) ;
#20460=DIRECTION('center_axis',(-1.,0.,0.)) ;
#20461=DIRECTION('ref_axis',(0.,1.,-1.83697019872103E-16)) ;
#20462=DIRECTION('',(-1.,0.,0.)) ;
#20463=DIRECTION('center_axis',(-1.,0.,0.)) ;
#20464=DIRECTION('ref_axis',(0.,1.,-1.83697019872103E-16)) ;
#20465=DIRECTION('center_axis',(1.,0.,0.)) ;
#20466=DIRECTION('ref_axis',(0.,-0.994521895368273,0.104528463267653)) ;
#20467=DIRECTION('center_axis',(1.,0.,0.)) ;
#20468=DIRECTION('ref_axis',(0.,-0.994521895368273,0.104528463267653)) ;
#20469=DIRECTION('center_axis',(1.,0.,0.)) ;
#20470=DIRECTION('ref_axis',(0.,-0.994521895368273,0.104528463267653)) ;
#20471=DIRECTION('center_axis',(1.,0.,0.)) ;
#20472=DIRECTION('ref_axis',(0.,-0.994521895368273,0.104528463267653)) ;
#20473=DIRECTION('center_axis',(1.,0.,0.)) ;
#20474=DIRECTION('ref_axis',(0.,-0.994521895368273,0.104528463267653)) ;
#20475=DIRECTION('center_axis',(1.,0.,0.)) ;
#20476=DIRECTION('ref_axis',(0.,-0.994521895368273,0.104528463267653)) ;
#20477=DIRECTION('center_axis',(1.,0.,0.)) ;
#20478=DIRECTION('ref_axis',(0.,-0.994521895368273,0.104528463267653)) ;
#20479=DIRECTION('center_axis',(1.,0.,0.)) ;
#20480=DIRECTION('ref_axis',(0.,-0.994521895368273,0.104528463267653)) ;
#20481=DIRECTION('center_axis',(-1.,0.,0.)) ;
#20482=DIRECTION('ref_axis',(0.,0.994521895368273,-0.104528463267653)) ;
#20483=DIRECTION('',(-1.,0.,0.)) ;
#20484=DIRECTION('center_axis',(-1.,0.,0.)) ;
#20485=DIRECTION('ref_axis',(0.,0.994521895368273,-0.104528463267653)) ;
#20486=DIRECTION('',(-1.,0.,0.)) ;
#20487=DIRECTION('center_axis',(-1.,0.,0.)) ;
#20488=DIRECTION('ref_axis',(0.,0.994521895368273,-0.104528463267653)) ;
#20489=DIRECTION('center_axis',(1.,0.,0.)) ;
#20490=DIRECTION('ref_axis',(0.,-0.978147600733805,0.20791169081776)) ;
#20491=DIRECTION('center_axis',(1.,0.,0.)) ;
#20492=DIRECTION('ref_axis',(0.,-0.978147600733805,0.20791169081776)) ;
#20493=DIRECTION('center_axis',(1.,0.,0.)) ;
#20494=DIRECTION('ref_axis',(0.,-0.978147600733805,0.20791169081776)) ;
#20495=DIRECTION('center_axis',(1.,0.,0.)) ;
#20496=DIRECTION('ref_axis',(0.,-0.978147600733805,0.20791169081776)) ;
#20497=DIRECTION('center_axis',(1.,0.,0.)) ;
#20498=DIRECTION('ref_axis',(0.,-0.978147600733805,0.20791169081776)) ;
#20499=DIRECTION('center_axis',(1.,0.,0.)) ;
#20500=DIRECTION('ref_axis',(0.,-0.978147600733805,0.20791169081776)) ;
#20501=DIRECTION('center_axis',(1.,0.,0.)) ;
#20502=DIRECTION('ref_axis',(0.,-0.978147600733805,0.20791169081776)) ;
#20503=DIRECTION('center_axis',(1.,0.,0.)) ;
#20504=DIRECTION('ref_axis',(0.,-0.978147600733805,0.20791169081776)) ;
#20505=DIRECTION('center_axis',(-1.,0.,0.)) ;
#20506=DIRECTION('ref_axis',(0.,0.978147600733805,-0.20791169081776)) ;
#20507=DIRECTION('',(-1.,0.,0.)) ;
#20508=DIRECTION('center_axis',(-1.,0.,0.)) ;
#20509=DIRECTION('ref_axis',(0.,0.978147600733805,-0.20791169081776)) ;
#20510=DIRECTION('',(-1.,0.,0.)) ;
#20511=DIRECTION('center_axis',(-1.,0.,0.)) ;
#20512=DIRECTION('ref_axis',(0.,0.978147600733805,-0.20791169081776)) ;
#20513=DIRECTION('center_axis',(1.,0.,0.)) ;
#20514=DIRECTION('ref_axis',(0.,-0.951056516295154,0.309016994374948)) ;
#20515=DIRECTION('center_axis',(1.,0.,0.)) ;
#20516=DIRECTION('ref_axis',(0.,-0.951056516295153,0.309016994374948)) ;
#20517=DIRECTION('center_axis',(1.,0.,0.)) ;
#20518=DIRECTION('ref_axis',(0.,-0.951056516295154,0.309016994374948)) ;
#20519=DIRECTION('center_axis',(1.,0.,0.)) ;
#20520=DIRECTION('ref_axis',(0.,-0.951056516295153,0.309016994374948)) ;
#20521=DIRECTION('center_axis',(1.,0.,0.)) ;
#20522=DIRECTION('ref_axis',(0.,-0.951056516295154,0.309016994374948)) ;
#20523=DIRECTION('center_axis',(1.,0.,0.)) ;
#20524=DIRECTION('ref_axis',(0.,-0.951056516295153,0.309016994374948)) ;
#20525=DIRECTION('center_axis',(1.,0.,0.)) ;
#20526=DIRECTION('ref_axis',(0.,-0.951056516295154,0.309016994374948)) ;
#20527=DIRECTION('center_axis',(1.,0.,0.)) ;
#20528=DIRECTION('ref_axis',(0.,-0.951056516295153,0.309016994374948)) ;
#20529=DIRECTION('center_axis',(-1.,0.,0.)) ;
#20530=DIRECTION('ref_axis',(0.,0.951056516295153,-0.309016994374948)) ;
#20531=DIRECTION('',(-1.,0.,0.)) ;
#20532=DIRECTION('center_axis',(-1.,0.,0.)) ;
#20533=DIRECTION('ref_axis',(0.,0.951056516295154,-0.309016994374948)) ;
#20534=DIRECTION('',(-1.,0.,0.)) ;
#20535=DIRECTION('center_axis',(-1.,0.,0.)) ;
#20536=DIRECTION('ref_axis',(0.,0.951056516295153,-0.309016994374948)) ;
#20537=DIRECTION('center_axis',(1.,0.,0.)) ;
#20538=DIRECTION('ref_axis',(0.,-0.4067366430758,0.913545457642601)) ;
#20539=DIRECTION('center_axis',(1.,0.,0.)) ;
#20540=DIRECTION('ref_axis',(0.,-0.4067366430758,0.913545457642601)) ;
#20541=DIRECTION('center_axis',(1.,0.,0.)) ;
#20542=DIRECTION('ref_axis',(0.,-0.4067366430758,0.913545457642601)) ;
#20543=DIRECTION('center_axis',(1.,0.,0.)) ;
#20544=DIRECTION('ref_axis',(0.,-0.4067366430758,0.913545457642601)) ;
#20545=DIRECTION('center_axis',(1.,0.,0.)) ;
#20546=DIRECTION('ref_axis',(0.,-0.4067366430758,0.913545457642601)) ;
#20547=DIRECTION('center_axis',(1.,0.,0.)) ;
#20548=DIRECTION('ref_axis',(0.,-0.4067366430758,0.913545457642601)) ;
#20549=DIRECTION('center_axis',(1.,0.,0.)) ;
#20550=DIRECTION('ref_axis',(0.,-0.4067366430758,0.913545457642601)) ;
#20551=DIRECTION('center_axis',(1.,0.,0.)) ;
#20552=DIRECTION('ref_axis',(0.,-0.4067366430758,0.913545457642601)) ;
#20553=DIRECTION('center_axis',(-1.,0.,0.)) ;
#20554=DIRECTION('ref_axis',(0.,0.4067366430758,-0.913545457642601)) ;
#20555=DIRECTION('',(-1.,0.,0.)) ;
#20556=DIRECTION('center_axis',(-1.,0.,0.)) ;
#20557=DIRECTION('ref_axis',(0.,0.4067366430758,-0.913545457642601)) ;
#20558=DIRECTION('',(-1.,0.,0.)) ;
#20559=DIRECTION('center_axis',(-1.,0.,0.)) ;
#20560=DIRECTION('ref_axis',(0.,0.4067366430758,-0.913545457642601)) ;
#20561=DIRECTION('center_axis',(1.,0.,0.)) ;
#20562=DIRECTION('ref_axis',(0.,-0.499999999999999,0.866025403784439)) ;
#20563=DIRECTION('center_axis',(1.,0.,0.)) ;
#20564=DIRECTION('ref_axis',(0.,-0.499999999999999,0.866025403784439)) ;
#20565=DIRECTION('center_axis',(1.,0.,0.)) ;
#20566=DIRECTION('ref_axis',(0.,-0.499999999999999,0.866025403784439)) ;
#20567=DIRECTION('center_axis',(1.,0.,0.)) ;
#20568=DIRECTION('ref_axis',(0.,-0.499999999999999,0.866025403784439)) ;
#20569=DIRECTION('center_axis',(1.,0.,0.)) ;
#20570=DIRECTION('ref_axis',(0.,-0.499999999999999,0.866025403784439)) ;
#20571=DIRECTION('center_axis',(1.,0.,0.)) ;
#20572=DIRECTION('ref_axis',(0.,-0.499999999999999,0.866025403784439)) ;
#20573=DIRECTION('center_axis',(1.,0.,0.)) ;
#20574=DIRECTION('ref_axis',(0.,-0.499999999999999,0.866025403784439)) ;
#20575=DIRECTION('center_axis',(1.,0.,0.)) ;
#20576=DIRECTION('ref_axis',(0.,-0.499999999999999,0.866025403784439)) ;
#20577=DIRECTION('center_axis',(-1.,0.,0.)) ;
#20578=DIRECTION('ref_axis',(0.,0.499999999999999,-0.866025403784439)) ;
#20579=DIRECTION('',(-1.,0.,0.)) ;
#20580=DIRECTION('center_axis',(-1.,0.,0.)) ;
#20581=DIRECTION('ref_axis',(0.,0.499999999999999,-0.866025403784439)) ;
#20582=DIRECTION('',(-1.,0.,0.)) ;
#20583=DIRECTION('center_axis',(-1.,0.,0.)) ;
#20584=DIRECTION('ref_axis',(0.,0.499999999999999,-0.866025403784439)) ;
#20585=DIRECTION('center_axis',(1.,0.,0.)) ;
#20586=DIRECTION('ref_axis',(0.,-0.587785252292473,0.809016994374947)) ;
#20587=DIRECTION('center_axis',(1.,0.,0.)) ;
#20588=DIRECTION('ref_axis',(0.,-0.587785252292473,0.809016994374947)) ;
#20589=DIRECTION('center_axis',(1.,0.,0.)) ;
#20590=DIRECTION('ref_axis',(0.,-0.587785252292473,0.809016994374947)) ;
#20591=DIRECTION('center_axis',(1.,0.,0.)) ;
#20592=DIRECTION('ref_axis',(0.,-0.587785252292473,0.809016994374947)) ;
#20593=DIRECTION('center_axis',(1.,0.,0.)) ;
#20594=DIRECTION('ref_axis',(0.,-0.587785252292473,0.809016994374947)) ;
#20595=DIRECTION('center_axis',(1.,0.,0.)) ;
#20596=DIRECTION('ref_axis',(0.,-0.587785252292473,0.809016994374947)) ;
#20597=DIRECTION('center_axis',(1.,0.,0.)) ;
#20598=DIRECTION('ref_axis',(0.,-0.587785252292473,0.809016994374947)) ;
#20599=DIRECTION('center_axis',(1.,0.,0.)) ;
#20600=DIRECTION('ref_axis',(0.,-0.587785252292473,0.809016994374947)) ;
#20601=DIRECTION('center_axis',(-1.,0.,0.)) ;
#20602=DIRECTION('ref_axis',(0.,0.587785252292473,-0.809016994374947)) ;
#20603=DIRECTION('',(-1.,0.,0.)) ;
#20604=DIRECTION('center_axis',(-1.,0.,0.)) ;
#20605=DIRECTION('ref_axis',(0.,0.587785252292473,-0.809016994374947)) ;
#20606=DIRECTION('',(-1.,0.,0.)) ;
#20607=DIRECTION('center_axis',(-1.,0.,0.)) ;
#20608=DIRECTION('ref_axis',(0.,0.587785252292473,-0.809016994374947)) ;
#20609=DIRECTION('center_axis',(1.,0.,0.)) ;
#20610=DIRECTION('ref_axis',(0.,-0.669130606358858,0.743144825477394)) ;
#20611=DIRECTION('center_axis',(1.,0.,0.)) ;
#20612=DIRECTION('ref_axis',(0.,-0.669130606358858,0.743144825477394)) ;
#20613=DIRECTION('center_axis',(1.,0.,0.)) ;
#20614=DIRECTION('ref_axis',(0.,-0.669130606358858,0.743144825477394)) ;
#20615=DIRECTION('center_axis',(1.,0.,0.)) ;
#20616=DIRECTION('ref_axis',(0.,-0.669130606358858,0.743144825477394)) ;
#20617=DIRECTION('center_axis',(1.,0.,0.)) ;
#20618=DIRECTION('ref_axis',(0.,-0.669130606358858,0.743144825477394)) ;
#20619=DIRECTION('center_axis',(1.,0.,0.)) ;
#20620=DIRECTION('ref_axis',(0.,-0.669130606358858,0.743144825477394)) ;
#20621=DIRECTION('center_axis',(1.,0.,0.)) ;
#20622=DIRECTION('ref_axis',(0.,-0.669130606358858,0.743144825477394)) ;
#20623=DIRECTION('center_axis',(1.,0.,0.)) ;
#20624=DIRECTION('ref_axis',(0.,-0.669130606358858,0.743144825477394)) ;
#20625=DIRECTION('center_axis',(-1.,0.,0.)) ;
#20626=DIRECTION('ref_axis',(0.,0.669130606358858,-0.743144825477394)) ;
#20627=DIRECTION('',(-1.,0.,0.)) ;
#20628=DIRECTION('center_axis',(-1.,0.,0.)) ;
#20629=DIRECTION('ref_axis',(0.,0.669130606358858,-0.743144825477394)) ;
#20630=DIRECTION('',(-1.,0.,0.)) ;
#20631=DIRECTION('center_axis',(-1.,0.,0.)) ;
#20632=DIRECTION('ref_axis',(0.,0.669130606358858,-0.743144825477394)) ;
#20633=DIRECTION('center_axis',(1.,0.,0.)) ;
#20634=DIRECTION('ref_axis',(0.,-0.743144825477394,0.669130606358858)) ;
#20635=DIRECTION('center_axis',(1.,0.,0.)) ;
#20636=DIRECTION('ref_axis',(0.,-0.743144825477394,0.669130606358858)) ;
#20637=DIRECTION('center_axis',(1.,0.,0.)) ;
#20638=DIRECTION('ref_axis',(0.,-0.743144825477394,0.669130606358858)) ;
#20639=DIRECTION('center_axis',(1.,0.,0.)) ;
#20640=DIRECTION('ref_axis',(0.,-0.743144825477394,0.669130606358858)) ;
#20641=DIRECTION('center_axis',(1.,0.,0.)) ;
#20642=DIRECTION('ref_axis',(0.,-0.743144825477394,0.669130606358858)) ;
#20643=DIRECTION('center_axis',(1.,0.,0.)) ;
#20644=DIRECTION('ref_axis',(0.,-0.743144825477394,0.669130606358858)) ;
#20645=DIRECTION('center_axis',(1.,0.,0.)) ;
#20646=DIRECTION('ref_axis',(0.,-0.743144825477394,0.669130606358858)) ;
#20647=DIRECTION('center_axis',(1.,0.,0.)) ;
#20648=DIRECTION('ref_axis',(0.,-0.743144825477394,0.669130606358858)) ;
#20649=DIRECTION('center_axis',(-1.,0.,0.)) ;
#20650=DIRECTION('ref_axis',(0.,0.743144825477394,-0.669130606358858)) ;
#20651=DIRECTION('',(-1.,0.,0.)) ;
#20652=DIRECTION('center_axis',(-1.,0.,0.)) ;
#20653=DIRECTION('ref_axis',(0.,0.743144825477394,-0.669130606358858)) ;
#20654=DIRECTION('',(-1.,0.,0.)) ;
#20655=DIRECTION('center_axis',(-1.,0.,0.)) ;
#20656=DIRECTION('ref_axis',(0.,0.743144825477394,-0.669130606358858)) ;
#20657=DIRECTION('center_axis',(1.,0.,0.)) ;
#20658=DIRECTION('ref_axis',(0.,-0.809016994374947,0.587785252292473)) ;
#20659=DIRECTION('center_axis',(1.,0.,0.)) ;
#20660=DIRECTION('ref_axis',(0.,-0.809016994374947,0.587785252292473)) ;
#20661=DIRECTION('center_axis',(1.,0.,0.)) ;
#20662=DIRECTION('ref_axis',(0.,-0.809016994374947,0.587785252292473)) ;
#20663=DIRECTION('center_axis',(1.,0.,0.)) ;
#20664=DIRECTION('ref_axis',(0.,-0.809016994374947,0.587785252292473)) ;
#20665=DIRECTION('center_axis',(1.,0.,0.)) ;
#20666=DIRECTION('ref_axis',(0.,-0.809016994374947,0.587785252292473)) ;
#20667=DIRECTION('center_axis',(1.,0.,0.)) ;
#20668=DIRECTION('ref_axis',(0.,-0.809016994374947,0.587785252292473)) ;
#20669=DIRECTION('center_axis',(1.,0.,0.)) ;
#20670=DIRECTION('ref_axis',(0.,-0.809016994374947,0.587785252292473)) ;
#20671=DIRECTION('center_axis',(1.,0.,0.)) ;
#20672=DIRECTION('ref_axis',(0.,-0.809016994374947,0.587785252292473)) ;
#20673=DIRECTION('center_axis',(-1.,0.,0.)) ;
#20674=DIRECTION('ref_axis',(0.,0.809016994374947,-0.587785252292473)) ;
#20675=DIRECTION('',(-1.,0.,0.)) ;
#20676=DIRECTION('center_axis',(-1.,0.,0.)) ;
#20677=DIRECTION('ref_axis',(0.,0.809016994374947,-0.587785252292473)) ;
#20678=DIRECTION('',(-1.,0.,0.)) ;
#20679=DIRECTION('center_axis',(-1.,0.,0.)) ;
#20680=DIRECTION('ref_axis',(0.,0.809016994374947,-0.587785252292473)) ;
#20681=DIRECTION('center_axis',(1.,0.,0.)) ;
#20682=DIRECTION('ref_axis',(0.,-0.866025403784438,0.5)) ;
#20683=DIRECTION('center_axis',(1.,0.,0.)) ;
#20684=DIRECTION('ref_axis',(0.,-0.866025403784438,0.5)) ;
#20685=DIRECTION('center_axis',(1.,0.,0.)) ;
#20686=DIRECTION('ref_axis',(0.,-0.866025403784438,0.5)) ;
#20687=DIRECTION('center_axis',(1.,0.,0.)) ;
#20688=DIRECTION('ref_axis',(0.,-0.866025403784438,0.5)) ;
#20689=DIRECTION('center_axis',(1.,0.,0.)) ;
#20690=DIRECTION('ref_axis',(0.,-0.866025403784438,0.5)) ;
#20691=DIRECTION('center_axis',(1.,0.,0.)) ;
#20692=DIRECTION('ref_axis',(0.,-0.866025403784438,0.5)) ;
#20693=DIRECTION('center_axis',(1.,0.,0.)) ;
#20694=DIRECTION('ref_axis',(0.,-0.866025403784438,0.5)) ;
#20695=DIRECTION('center_axis',(1.,0.,0.)) ;
#20696=DIRECTION('ref_axis',(0.,-0.866025403784438,0.5)) ;
#20697=DIRECTION('center_axis',(-1.,0.,0.)) ;
#20698=DIRECTION('ref_axis',(0.,0.866025403784438,-0.5)) ;
#20699=DIRECTION('',(-1.,0.,0.)) ;
#20700=DIRECTION('center_axis',(-1.,0.,0.)) ;
#20701=DIRECTION('ref_axis',(0.,0.866025403784438,-0.5)) ;
#20702=DIRECTION('',(-1.,0.,0.)) ;
#20703=DIRECTION('center_axis',(-1.,0.,0.)) ;
#20704=DIRECTION('ref_axis',(0.,0.866025403784438,-0.5)) ;
#20705=DIRECTION('center_axis',(1.,0.,0.)) ;
#20706=DIRECTION('ref_axis',(0.,-0.913545457642601,0.4067366430758)) ;
#20707=DIRECTION('center_axis',(1.,0.,0.)) ;
#20708=DIRECTION('ref_axis',(0.,-0.913545457642601,0.4067366430758)) ;
#20709=DIRECTION('center_axis',(1.,0.,0.)) ;
#20710=DIRECTION('ref_axis',(0.,-0.913545457642601,0.4067366430758)) ;
#20711=DIRECTION('center_axis',(1.,0.,0.)) ;
#20712=DIRECTION('ref_axis',(0.,-0.913545457642601,0.4067366430758)) ;
#20713=DIRECTION('center_axis',(1.,0.,0.)) ;
#20714=DIRECTION('ref_axis',(0.,-0.913545457642601,0.4067366430758)) ;
#20715=DIRECTION('center_axis',(1.,0.,0.)) ;
#20716=DIRECTION('ref_axis',(0.,-0.913545457642601,0.4067366430758)) ;
#20717=DIRECTION('center_axis',(1.,0.,0.)) ;
#20718=DIRECTION('ref_axis',(0.,-0.913545457642601,0.4067366430758)) ;
#20719=DIRECTION('center_axis',(1.,0.,0.)) ;
#20720=DIRECTION('ref_axis',(0.,-0.913545457642601,0.4067366430758)) ;
#20721=DIRECTION('center_axis',(-1.,0.,0.)) ;
#20722=DIRECTION('ref_axis',(0.,0.913545457642601,-0.4067366430758)) ;
#20723=DIRECTION('',(-1.,0.,0.)) ;
#20724=DIRECTION('center_axis',(-1.,0.,0.)) ;
#20725=DIRECTION('ref_axis',(0.,0.913545457642601,-0.4067366430758)) ;
#20726=DIRECTION('',(-1.,0.,0.)) ;
#20727=DIRECTION('center_axis',(-1.,0.,0.)) ;
#20728=DIRECTION('ref_axis',(0.,0.913545457642601,-0.4067366430758)) ;
#20729=DIRECTION('center_axis',(1.,0.,0.)) ;
#20730=DIRECTION('ref_axis',(0.,-0.309016994374948,0.951056516295154)) ;
#20731=DIRECTION('center_axis',(1.,0.,0.)) ;
#20732=DIRECTION('ref_axis',(0.,-0.309016994374948,0.951056516295153)) ;
#20733=DIRECTION('center_axis',(1.,0.,0.)) ;
#20734=DIRECTION('ref_axis',(0.,-0.309016994374948,0.951056516295154)) ;
#20735=DIRECTION('center_axis',(1.,0.,0.)) ;
#20736=DIRECTION('ref_axis',(0.,-0.309016994374948,0.951056516295153)) ;
#20737=DIRECTION('center_axis',(1.,0.,0.)) ;
#20738=DIRECTION('ref_axis',(0.,-0.309016994374948,0.951056516295154)) ;
#20739=DIRECTION('center_axis',(1.,0.,0.)) ;
#20740=DIRECTION('ref_axis',(0.,-0.309016994374948,0.951056516295153)) ;
#20741=DIRECTION('center_axis',(1.,0.,0.)) ;
#20742=DIRECTION('ref_axis',(0.,-0.309016994374948,0.951056516295154)) ;
#20743=DIRECTION('center_axis',(1.,0.,0.)) ;
#20744=DIRECTION('ref_axis',(0.,-0.309016994374948,0.951056516295153)) ;
#20745=DIRECTION('center_axis',(-1.,0.,0.)) ;
#20746=DIRECTION('ref_axis',(0.,0.309016994374948,-0.951056516295153)) ;
#20747=DIRECTION('',(-1.,0.,0.)) ;
#20748=DIRECTION('center_axis',(-1.,0.,0.)) ;
#20749=DIRECTION('ref_axis',(0.,0.309016994374948,-0.951056516295154)) ;
#20750=DIRECTION('',(-1.,0.,0.)) ;
#20751=DIRECTION('center_axis',(-1.,0.,0.)) ;
#20752=DIRECTION('ref_axis',(0.,0.309016994374948,-0.951056516295153)) ;
#20753=DIRECTION('center_axis',(1.,0.,0.)) ;
#20754=DIRECTION('ref_axis',(0.,-0.207911690817759,0.978147600733806)) ;
#20755=DIRECTION('center_axis',(1.,0.,0.)) ;
#20756=DIRECTION('ref_axis',(0.,-0.207911690817759,0.978147600733806)) ;
#20757=DIRECTION('center_axis',(1.,0.,0.)) ;
#20758=DIRECTION('ref_axis',(0.,-0.207911690817759,0.978147600733806)) ;
#20759=DIRECTION('center_axis',(1.,0.,0.)) ;
#20760=DIRECTION('ref_axis',(0.,-0.207911690817759,0.978147600733806)) ;
#20761=DIRECTION('center_axis',(1.,0.,0.)) ;
#20762=DIRECTION('ref_axis',(0.,-0.207911690817759,0.978147600733806)) ;
#20763=DIRECTION('center_axis',(1.,0.,0.)) ;
#20764=DIRECTION('ref_axis',(0.,-0.207911690817759,0.978147600733806)) ;
#20765=DIRECTION('center_axis',(1.,0.,0.)) ;
#20766=DIRECTION('ref_axis',(0.,-0.207911690817759,0.978147600733806)) ;
#20767=DIRECTION('center_axis',(1.,0.,0.)) ;
#20768=DIRECTION('ref_axis',(0.,-0.207911690817759,0.978147600733806)) ;
#20769=DIRECTION('center_axis',(-1.,0.,0.)) ;
#20770=DIRECTION('ref_axis',(0.,0.207911690817759,-0.978147600733806)) ;
#20771=DIRECTION('',(-1.,0.,0.)) ;
#20772=DIRECTION('center_axis',(-1.,0.,0.)) ;
#20773=DIRECTION('ref_axis',(0.,0.207911690817759,-0.978147600733806)) ;
#20774=DIRECTION('',(-1.,0.,0.)) ;
#20775=DIRECTION('center_axis',(-1.,0.,0.)) ;
#20776=DIRECTION('ref_axis',(0.,0.207911690817759,-0.978147600733806)) ;
#20777=DIRECTION('center_axis',(1.,0.,0.)) ;
#20778=DIRECTION('ref_axis',(0.,-0.104528463267653,0.994521895368273)) ;
#20779=DIRECTION('center_axis',(1.,0.,0.)) ;
#20780=DIRECTION('ref_axis',(0.,-0.104528463267653,0.994521895368273)) ;
#20781=DIRECTION('center_axis',(1.,0.,0.)) ;
#20782=DIRECTION('ref_axis',(0.,-0.104528463267653,0.994521895368273)) ;
#20783=DIRECTION('center_axis',(1.,0.,0.)) ;
#20784=DIRECTION('ref_axis',(0.,-0.104528463267653,0.994521895368273)) ;
#20785=DIRECTION('center_axis',(1.,0.,0.)) ;
#20786=DIRECTION('ref_axis',(0.,-0.104528463267653,0.994521895368273)) ;
#20787=DIRECTION('center_axis',(1.,0.,0.)) ;
#20788=DIRECTION('ref_axis',(0.,-0.104528463267653,0.994521895368273)) ;
#20789=DIRECTION('center_axis',(1.,0.,0.)) ;
#20790=DIRECTION('ref_axis',(0.,-0.104528463267653,0.994521895368273)) ;
#20791=DIRECTION('center_axis',(1.,0.,0.)) ;
#20792=DIRECTION('ref_axis',(0.,-0.104528463267653,0.994521895368273)) ;
#20793=DIRECTION('center_axis',(-1.,0.,0.)) ;
#20794=DIRECTION('ref_axis',(0.,0.104528463267653,-0.994521895368273)) ;
#20795=DIRECTION('',(-1.,0.,0.)) ;
#20796=DIRECTION('center_axis',(-1.,0.,0.)) ;
#20797=DIRECTION('ref_axis',(0.,0.104528463267653,-0.994521895368273)) ;
#20798=DIRECTION('',(-1.,0.,0.)) ;
#20799=DIRECTION('center_axis',(-1.,0.,0.)) ;
#20800=DIRECTION('ref_axis',(0.,0.104528463267653,-0.994521895368273)) ;
#20801=DIRECTION('center_axis',(1.,0.,0.)) ;
#20802=DIRECTION('ref_axis',(0.,1.22464679914735E-16,1.)) ;
#20803=DIRECTION('center_axis',(1.,0.,0.)) ;
#20804=DIRECTION('ref_axis',(0.,1.22464679914735E-16,1.)) ;
#20805=DIRECTION('center_axis',(1.,0.,0.)) ;
#20806=DIRECTION('ref_axis',(0.,1.22464679914735E-16,1.)) ;
#20807=DIRECTION('center_axis',(1.,0.,0.)) ;
#20808=DIRECTION('ref_axis',(0.,1.22464679914735E-16,1.)) ;
#20809=DIRECTION('center_axis',(1.,0.,0.)) ;
#20810=DIRECTION('ref_axis',(0.,1.22464679914735E-16,1.)) ;
#20811=DIRECTION('center_axis',(1.,0.,0.)) ;
#20812=DIRECTION('ref_axis',(0.,1.22464679914735E-16,1.)) ;
#20813=DIRECTION('center_axis',(1.,0.,0.)) ;
#20814=DIRECTION('ref_axis',(0.,1.22464679914735E-16,1.)) ;
#20815=DIRECTION('center_axis',(1.,0.,0.)) ;
#20816=DIRECTION('ref_axis',(0.,1.22464679914735E-16,1.)) ;
#20817=DIRECTION('center_axis',(-1.,0.,0.)) ;
#20818=DIRECTION('ref_axis',(0.,-1.22464679914735E-16,-1.)) ;
#20819=DIRECTION('',(-1.,0.,0.)) ;
#20820=DIRECTION('center_axis',(-1.,0.,0.)) ;
#20821=DIRECTION('ref_axis',(0.,-1.22464679914735E-16,-1.)) ;
#20822=DIRECTION('',(-1.,0.,0.)) ;
#20823=DIRECTION('center_axis',(-1.,0.,0.)) ;
#20824=DIRECTION('ref_axis',(0.,-1.22464679914735E-16,-1.)) ;
#20825=DIRECTION('center_axis',(1.,0.,0.)) ;
#20826=DIRECTION('ref_axis',(0.,0.104528463267654,0.994521895368273)) ;
#20827=DIRECTION('center_axis',(1.,0.,0.)) ;
#20828=DIRECTION('ref_axis',(0.,0.104528463267654,0.994521895368273)) ;
#20829=DIRECTION('center_axis',(1.,0.,0.)) ;
#20830=DIRECTION('ref_axis',(0.,0.104528463267654,0.994521895368273)) ;
#20831=DIRECTION('center_axis',(1.,0.,0.)) ;
#20832=DIRECTION('ref_axis',(0.,0.104528463267654,0.994521895368273)) ;
#20833=DIRECTION('center_axis',(1.,0.,0.)) ;
#20834=DIRECTION('ref_axis',(0.,0.104528463267654,0.994521895368273)) ;
#20835=DIRECTION('center_axis',(1.,0.,0.)) ;
#20836=DIRECTION('ref_axis',(0.,0.104528463267654,0.994521895368273)) ;
#20837=DIRECTION('center_axis',(1.,0.,0.)) ;
#20838=DIRECTION('ref_axis',(0.,0.104528463267654,0.994521895368273)) ;
#20839=DIRECTION('center_axis',(1.,0.,0.)) ;
#20840=DIRECTION('ref_axis',(0.,0.104528463267654,0.994521895368273)) ;
#20841=DIRECTION('center_axis',(-1.,0.,0.)) ;
#20842=DIRECTION('ref_axis',(0.,-0.104528463267654,-0.994521895368273)) ;
#20843=DIRECTION('',(-1.,0.,0.)) ;
#20844=DIRECTION('center_axis',(-1.,0.,0.)) ;
#20845=DIRECTION('ref_axis',(0.,-0.104528463267654,-0.994521895368273)) ;
#20846=DIRECTION('',(-1.,0.,0.)) ;
#20847=DIRECTION('center_axis',(-1.,0.,0.)) ;
#20848=DIRECTION('ref_axis',(0.,-0.104528463267654,-0.994521895368273)) ;
#20849=DIRECTION('center_axis',(1.,0.,0.)) ;
#20850=DIRECTION('ref_axis',(0.,0.207911690817759,0.978147600733806)) ;
#20851=DIRECTION('center_axis',(1.,0.,0.)) ;
#20852=DIRECTION('ref_axis',(0.,0.207911690817759,0.978147600733806)) ;
#20853=DIRECTION('center_axis',(1.,0.,0.)) ;
#20854=DIRECTION('ref_axis',(0.,0.207911690817759,0.978147600733806)) ;
#20855=DIRECTION('center_axis',(1.,0.,0.)) ;
#20856=DIRECTION('ref_axis',(0.,0.207911690817759,0.978147600733806)) ;
#20857=DIRECTION('center_axis',(1.,0.,0.)) ;
#20858=DIRECTION('ref_axis',(0.,0.207911690817759,0.978147600733806)) ;
#20859=DIRECTION('center_axis',(1.,0.,0.)) ;
#20860=DIRECTION('ref_axis',(0.,0.207911690817759,0.978147600733806)) ;
#20861=DIRECTION('center_axis',(1.,0.,0.)) ;
#20862=DIRECTION('ref_axis',(0.,0.207911690817759,0.978147600733806)) ;
#20863=DIRECTION('center_axis',(1.,0.,0.)) ;
#20864=DIRECTION('ref_axis',(0.,0.207911690817759,0.978147600733806)) ;
#20865=DIRECTION('center_axis',(-1.,0.,0.)) ;
#20866=DIRECTION('ref_axis',(0.,-0.207911690817759,-0.978147600733806)) ;
#20867=DIRECTION('',(-1.,0.,0.)) ;
#20868=DIRECTION('center_axis',(-1.,0.,0.)) ;
#20869=DIRECTION('ref_axis',(0.,-0.207911690817759,-0.978147600733806)) ;
#20870=DIRECTION('',(-1.,0.,0.)) ;
#20871=DIRECTION('center_axis',(-1.,0.,0.)) ;
#20872=DIRECTION('ref_axis',(0.,-0.207911690817759,-0.978147600733806)) ;
#20873=DIRECTION('center_axis',(1.,0.,0.)) ;
#20874=DIRECTION('ref_axis',(0.,0.309016994374948,0.951056516295154)) ;
#20875=DIRECTION('center_axis',(1.,0.,0.)) ;
#20876=DIRECTION('ref_axis',(0.,0.309016994374948,0.951056516295153)) ;
#20877=DIRECTION('center_axis',(1.,0.,0.)) ;
#20878=DIRECTION('ref_axis',(0.,0.309016994374948,0.951056516295154)) ;
#20879=DIRECTION('center_axis',(1.,0.,0.)) ;
#20880=DIRECTION('ref_axis',(0.,0.309016994374948,0.951056516295153)) ;
#20881=DIRECTION('center_axis',(1.,0.,0.)) ;
#20882=DIRECTION('ref_axis',(0.,0.309016994374948,0.951056516295154)) ;
#20883=DIRECTION('center_axis',(1.,0.,0.)) ;
#20884=DIRECTION('ref_axis',(0.,0.309016994374948,0.951056516295153)) ;
#20885=DIRECTION('center_axis',(1.,0.,0.)) ;
#20886=DIRECTION('ref_axis',(0.,0.309016994374948,0.951056516295154)) ;
#20887=DIRECTION('center_axis',(1.,0.,0.)) ;
#20888=DIRECTION('ref_axis',(0.,0.309016994374948,0.951056516295153)) ;
#20889=DIRECTION('center_axis',(-1.,0.,0.)) ;
#20890=DIRECTION('ref_axis',(0.,-0.309016994374948,-0.951056516295153)) ;
#20891=DIRECTION('',(-1.,0.,0.)) ;
#20892=DIRECTION('center_axis',(-1.,0.,0.)) ;
#20893=DIRECTION('ref_axis',(0.,-0.309016994374948,-0.951056516295154)) ;
#20894=DIRECTION('',(-1.,0.,0.)) ;
#20895=DIRECTION('center_axis',(-1.,0.,0.)) ;
#20896=DIRECTION('ref_axis',(0.,-0.309016994374948,-0.951056516295153)) ;
#20897=DIRECTION('center_axis',(1.,0.,0.)) ;
#20898=DIRECTION('ref_axis',(0.,0.4067366430758,0.913545457642601)) ;
#20899=DIRECTION('center_axis',(1.,0.,0.)) ;
#20900=DIRECTION('ref_axis',(0.,0.4067366430758,0.913545457642601)) ;
#20901=DIRECTION('center_axis',(1.,0.,0.)) ;
#20902=DIRECTION('ref_axis',(0.,0.4067366430758,0.913545457642601)) ;
#20903=DIRECTION('center_axis',(1.,0.,0.)) ;
#20904=DIRECTION('ref_axis',(0.,0.4067366430758,0.913545457642601)) ;
#20905=DIRECTION('center_axis',(1.,0.,0.)) ;
#20906=DIRECTION('ref_axis',(0.,0.4067366430758,0.913545457642601)) ;
#20907=DIRECTION('center_axis',(1.,0.,0.)) ;
#20908=DIRECTION('ref_axis',(0.,0.4067366430758,0.913545457642601)) ;
#20909=DIRECTION('center_axis',(1.,0.,0.)) ;
#20910=DIRECTION('ref_axis',(0.,0.4067366430758,0.913545457642601)) ;
#20911=DIRECTION('center_axis',(1.,0.,0.)) ;
#20912=DIRECTION('ref_axis',(0.,0.4067366430758,0.913545457642601)) ;
#20913=DIRECTION('center_axis',(-1.,0.,0.)) ;
#20914=DIRECTION('ref_axis',(0.,-0.4067366430758,-0.913545457642601)) ;
#20915=DIRECTION('',(-1.,0.,0.)) ;
#20916=DIRECTION('center_axis',(-1.,0.,0.)) ;
#20917=DIRECTION('ref_axis',(0.,-0.4067366430758,-0.913545457642601)) ;
#20918=DIRECTION('',(-1.,0.,0.)) ;
#20919=DIRECTION('center_axis',(-1.,0.,0.)) ;
#20920=DIRECTION('ref_axis',(0.,-0.4067366430758,-0.913545457642601)) ;
#20921=DIRECTION('center_axis',(1.,0.,0.)) ;
#20922=DIRECTION('ref_axis',(0.,0.5,0.866025403784439)) ;
#20923=DIRECTION('center_axis',(1.,0.,0.)) ;
#20924=DIRECTION('ref_axis',(0.,0.5,0.866025403784439)) ;
#20925=DIRECTION('center_axis',(1.,0.,0.)) ;
#20926=DIRECTION('ref_axis',(0.,0.5,0.866025403784439)) ;
#20927=DIRECTION('center_axis',(1.,0.,0.)) ;
#20928=DIRECTION('ref_axis',(0.,0.5,0.866025403784439)) ;
#20929=DIRECTION('center_axis',(1.,0.,0.)) ;
#20930=DIRECTION('ref_axis',(0.,0.5,0.866025403784439)) ;
#20931=DIRECTION('center_axis',(1.,0.,0.)) ;
#20932=DIRECTION('ref_axis',(0.,0.5,0.866025403784439)) ;
#20933=DIRECTION('center_axis',(1.,0.,0.)) ;
#20934=DIRECTION('ref_axis',(0.,0.5,0.866025403784439)) ;
#20935=DIRECTION('center_axis',(1.,0.,0.)) ;
#20936=DIRECTION('ref_axis',(0.,0.5,0.866025403784439)) ;
#20937=DIRECTION('center_axis',(-1.,0.,0.)) ;
#20938=DIRECTION('ref_axis',(0.,-0.5,-0.866025403784439)) ;
#20939=DIRECTION('',(-1.,0.,0.)) ;
#20940=DIRECTION('center_axis',(-1.,0.,0.)) ;
#20941=DIRECTION('ref_axis',(0.,-0.5,-0.866025403784439)) ;
#20942=DIRECTION('',(-1.,0.,0.)) ;
#20943=DIRECTION('center_axis',(-1.,0.,0.)) ;
#20944=DIRECTION('ref_axis',(0.,-0.5,-0.866025403784439)) ;
#20945=DIRECTION('center_axis',(1.,0.,0.)) ;
#20946=DIRECTION('ref_axis',(0.,0.587785252292474,0.809016994374947)) ;
#20947=DIRECTION('center_axis',(1.,0.,0.)) ;
#20948=DIRECTION('ref_axis',(0.,0.587785252292474,0.809016994374947)) ;
#20949=DIRECTION('center_axis',(1.,0.,0.)) ;
#20950=DIRECTION('ref_axis',(0.,0.587785252292474,0.809016994374947)) ;
#20951=DIRECTION('center_axis',(1.,0.,0.)) ;
#20952=DIRECTION('ref_axis',(0.,0.587785252292474,0.809016994374947)) ;
#20953=DIRECTION('center_axis',(1.,0.,0.)) ;
#20954=DIRECTION('ref_axis',(0.,0.587785252292474,0.809016994374947)) ;
#20955=DIRECTION('center_axis',(1.,0.,0.)) ;
#20956=DIRECTION('ref_axis',(0.,0.587785252292474,0.809016994374947)) ;
#20957=DIRECTION('center_axis',(1.,0.,0.)) ;
#20958=DIRECTION('ref_axis',(0.,0.587785252292474,0.809016994374947)) ;
#20959=DIRECTION('center_axis',(1.,0.,0.)) ;
#20960=DIRECTION('ref_axis',(0.,0.587785252292474,0.809016994374947)) ;
#20961=DIRECTION('center_axis',(-1.,0.,0.)) ;
#20962=DIRECTION('ref_axis',(0.,-0.587785252292474,-0.809016994374947)) ;
#20963=DIRECTION('',(-1.,0.,0.)) ;
#20964=DIRECTION('center_axis',(-1.,0.,0.)) ;
#20965=DIRECTION('ref_axis',(0.,-0.587785252292474,-0.809016994374947)) ;
#20966=DIRECTION('',(-1.,0.,0.)) ;
#20967=DIRECTION('center_axis',(-1.,0.,0.)) ;
#20968=DIRECTION('ref_axis',(0.,-0.587785252292474,-0.809016994374947)) ;
#20969=DIRECTION('center_axis',(1.,0.,0.)) ;
#20970=DIRECTION('ref_axis',(0.,0.743144825477395,0.669130606358858)) ;
#20971=DIRECTION('center_axis',(1.,0.,0.)) ;
#20972=DIRECTION('ref_axis',(0.,0.743144825477395,0.669130606358858)) ;
#20973=DIRECTION('center_axis',(1.,0.,0.)) ;
#20974=DIRECTION('ref_axis',(0.,0.743144825477395,0.669130606358858)) ;
#20975=DIRECTION('center_axis',(1.,0.,0.)) ;
#20976=DIRECTION('ref_axis',(0.,0.743144825477395,0.669130606358858)) ;
#20977=DIRECTION('center_axis',(1.,0.,0.)) ;
#20978=DIRECTION('ref_axis',(0.,0.743144825477395,0.669130606358858)) ;
#20979=DIRECTION('center_axis',(1.,0.,0.)) ;
#20980=DIRECTION('ref_axis',(0.,0.743144825477395,0.669130606358858)) ;
#20981=DIRECTION('center_axis',(1.,0.,0.)) ;
#20982=DIRECTION('ref_axis',(0.,0.743144825477395,0.669130606358858)) ;
#20983=DIRECTION('center_axis',(1.,0.,0.)) ;
#20984=DIRECTION('ref_axis',(0.,0.743144825477395,0.669130606358858)) ;
#20985=DIRECTION('center_axis',(-1.,0.,0.)) ;
#20986=DIRECTION('ref_axis',(0.,-0.743144825477395,-0.669130606358858)) ;
#20987=DIRECTION('',(-1.,0.,0.)) ;
#20988=DIRECTION('center_axis',(-1.,0.,0.)) ;
#20989=DIRECTION('ref_axis',(0.,-0.743144825477395,-0.669130606358858)) ;
#20990=DIRECTION('',(-1.,0.,0.)) ;
#20991=DIRECTION('center_axis',(-1.,0.,0.)) ;
#20992=DIRECTION('ref_axis',(0.,-0.743144825477395,-0.669130606358858)) ;
#20993=DIRECTION('center_axis',(1.,0.,0.)) ;
#20994=DIRECTION('ref_axis',(0.,0.669130606358858,0.743144825477394)) ;
#20995=DIRECTION('center_axis',(1.,0.,0.)) ;
#20996=DIRECTION('ref_axis',(0.,0.669130606358858,0.743144825477394)) ;
#20997=DIRECTION('center_axis',(1.,0.,0.)) ;
#20998=DIRECTION('ref_axis',(0.,0.669130606358858,0.743144825477394)) ;
#20999=DIRECTION('center_axis',(1.,0.,0.)) ;
#21000=DIRECTION('ref_axis',(0.,0.669130606358858,0.743144825477394)) ;
#21001=DIRECTION('center_axis',(1.,0.,0.)) ;
#21002=DIRECTION('ref_axis',(0.,0.669130606358858,0.743144825477394)) ;
#21003=DIRECTION('center_axis',(1.,0.,0.)) ;
#21004=DIRECTION('ref_axis',(0.,0.669130606358858,0.743144825477394)) ;
#21005=DIRECTION('center_axis',(1.,0.,0.)) ;
#21006=DIRECTION('ref_axis',(0.,0.669130606358858,0.743144825477394)) ;
#21007=DIRECTION('center_axis',(1.,0.,0.)) ;
#21008=DIRECTION('ref_axis',(0.,0.669130606358858,0.743144825477394)) ;
#21009=DIRECTION('center_axis',(-1.,0.,0.)) ;
#21010=DIRECTION('ref_axis',(0.,-0.669130606358858,-0.743144825477394)) ;
#21011=DIRECTION('',(-1.,0.,0.)) ;
#21012=DIRECTION('center_axis',(-1.,0.,0.)) ;
#21013=DIRECTION('ref_axis',(0.,-0.669130606358858,-0.743144825477394)) ;
#21014=DIRECTION('',(-1.,0.,0.)) ;
#21015=DIRECTION('center_axis',(-1.,0.,0.)) ;
#21016=DIRECTION('ref_axis',(0.,-0.669130606358858,-0.743144825477394)) ;
#21017=DIRECTION('center_axis',(1.,0.,0.)) ;
#21018=DIRECTION('ref_axis',(0.,0.809016994374948,0.587785252292473)) ;
#21019=DIRECTION('center_axis',(1.,0.,0.)) ;
#21020=DIRECTION('ref_axis',(0.,0.809016994374948,0.587785252292473)) ;
#21021=DIRECTION('center_axis',(1.,0.,0.)) ;
#21022=DIRECTION('ref_axis',(0.,0.809016994374948,0.587785252292473)) ;
#21023=DIRECTION('center_axis',(1.,0.,0.)) ;
#21024=DIRECTION('ref_axis',(0.,0.809016994374948,0.587785252292473)) ;
#21025=DIRECTION('center_axis',(1.,0.,0.)) ;
#21026=DIRECTION('ref_axis',(0.,0.809016994374948,0.587785252292473)) ;
#21027=DIRECTION('center_axis',(1.,0.,0.)) ;
#21028=DIRECTION('ref_axis',(0.,0.809016994374948,0.587785252292473)) ;
#21029=DIRECTION('center_axis',(1.,0.,0.)) ;
#21030=DIRECTION('ref_axis',(0.,0.809016994374948,0.587785252292473)) ;
#21031=DIRECTION('center_axis',(1.,0.,0.)) ;
#21032=DIRECTION('ref_axis',(0.,0.809016994374948,0.587785252292473)) ;
#21033=DIRECTION('center_axis',(-1.,0.,0.)) ;
#21034=DIRECTION('ref_axis',(0.,-0.809016994374948,-0.587785252292473)) ;
#21035=DIRECTION('',(-1.,0.,0.)) ;
#21036=DIRECTION('center_axis',(-1.,0.,0.)) ;
#21037=DIRECTION('ref_axis',(0.,-0.809016994374948,-0.587785252292473)) ;
#21038=DIRECTION('',(-1.,0.,0.)) ;
#21039=DIRECTION('center_axis',(-1.,0.,0.)) ;
#21040=DIRECTION('ref_axis',(0.,-0.809016994374948,-0.587785252292473)) ;
#21041=DIRECTION('center_axis',(1.,0.,0.)) ;
#21042=DIRECTION('ref_axis',(0.,0.866025403784439,0.499999999999999)) ;
#21043=DIRECTION('center_axis',(1.,0.,0.)) ;
#21044=DIRECTION('ref_axis',(0.,0.866025403784439,0.499999999999999)) ;
#21045=DIRECTION('center_axis',(1.,0.,0.)) ;
#21046=DIRECTION('ref_axis',(0.,0.866025403784439,0.499999999999999)) ;
#21047=DIRECTION('center_axis',(1.,0.,0.)) ;
#21048=DIRECTION('ref_axis',(0.,0.866025403784439,0.499999999999999)) ;
#21049=DIRECTION('center_axis',(1.,0.,0.)) ;
#21050=DIRECTION('ref_axis',(0.,0.866025403784439,0.499999999999999)) ;
#21051=DIRECTION('center_axis',(1.,0.,0.)) ;
#21052=DIRECTION('ref_axis',(0.,0.866025403784439,0.499999999999999)) ;
#21053=DIRECTION('center_axis',(1.,0.,0.)) ;
#21054=DIRECTION('ref_axis',(0.,0.866025403784439,0.499999999999999)) ;
#21055=DIRECTION('center_axis',(1.,0.,0.)) ;
#21056=DIRECTION('ref_axis',(0.,0.866025403784439,0.499999999999999)) ;
#21057=DIRECTION('center_axis',(-1.,0.,0.)) ;
#21058=DIRECTION('ref_axis',(0.,-0.866025403784439,-0.499999999999999)) ;
#21059=DIRECTION('',(-1.,0.,0.)) ;
#21060=DIRECTION('center_axis',(-1.,0.,0.)) ;
#21061=DIRECTION('ref_axis',(0.,-0.866025403784439,-0.499999999999999)) ;
#21062=DIRECTION('',(-1.,0.,0.)) ;
#21063=DIRECTION('center_axis',(-1.,0.,0.)) ;
#21064=DIRECTION('ref_axis',(0.,-0.866025403784439,-0.499999999999999)) ;
#21065=DIRECTION('center_axis',(1.,0.,0.)) ;
#21066=DIRECTION('ref_axis',(0.,0.913545457642601,0.4067366430758)) ;
#21067=DIRECTION('center_axis',(1.,0.,0.)) ;
#21068=DIRECTION('ref_axis',(0.,0.913545457642601,0.4067366430758)) ;
#21069=DIRECTION('center_axis',(1.,0.,0.)) ;
#21070=DIRECTION('ref_axis',(0.,0.913545457642601,0.4067366430758)) ;
#21071=DIRECTION('center_axis',(1.,0.,0.)) ;
#21072=DIRECTION('ref_axis',(0.,0.913545457642601,0.4067366430758)) ;
#21073=DIRECTION('center_axis',(1.,0.,0.)) ;
#21074=DIRECTION('ref_axis',(0.,0.913545457642601,0.4067366430758)) ;
#21075=DIRECTION('center_axis',(1.,0.,0.)) ;
#21076=DIRECTION('ref_axis',(0.,0.913545457642601,0.4067366430758)) ;
#21077=DIRECTION('center_axis',(1.,0.,0.)) ;
#21078=DIRECTION('ref_axis',(0.,0.913545457642601,0.4067366430758)) ;
#21079=DIRECTION('center_axis',(1.,0.,0.)) ;
#21080=DIRECTION('ref_axis',(0.,0.913545457642601,0.4067366430758)) ;
#21081=DIRECTION('center_axis',(-1.,0.,0.)) ;
#21082=DIRECTION('ref_axis',(0.,-0.913545457642601,-0.4067366430758)) ;
#21083=DIRECTION('',(-1.,0.,0.)) ;
#21084=DIRECTION('center_axis',(-1.,0.,0.)) ;
#21085=DIRECTION('ref_axis',(0.,-0.913545457642601,-0.4067366430758)) ;
#21086=DIRECTION('',(-1.,0.,0.)) ;
#21087=DIRECTION('center_axis',(-1.,0.,0.)) ;
#21088=DIRECTION('ref_axis',(0.,-0.913545457642601,-0.4067366430758)) ;
#21089=DIRECTION('center_axis',(1.,0.,0.)) ;
#21090=DIRECTION('ref_axis',(0.,0.951056516295154,0.309016994374947)) ;
#21091=DIRECTION('center_axis',(1.,0.,0.)) ;
#21092=DIRECTION('ref_axis',(0.,0.951056516295154,0.309016994374947)) ;
#21093=DIRECTION('center_axis',(1.,0.,0.)) ;
#21094=DIRECTION('ref_axis',(0.,0.951056516295154,0.309016994374947)) ;
#21095=DIRECTION('center_axis',(1.,0.,0.)) ;
#21096=DIRECTION('ref_axis',(0.,0.951056516295154,0.309016994374947)) ;
#21097=DIRECTION('center_axis',(1.,0.,0.)) ;
#21098=DIRECTION('ref_axis',(0.,0.951056516295154,0.309016994374947)) ;
#21099=DIRECTION('center_axis',(1.,0.,0.)) ;
#21100=DIRECTION('ref_axis',(0.,0.951056516295154,0.309016994374947)) ;
#21101=DIRECTION('center_axis',(1.,0.,0.)) ;
#21102=DIRECTION('ref_axis',(0.,0.951056516295154,0.309016994374947)) ;
#21103=DIRECTION('center_axis',(1.,0.,0.)) ;
#21104=DIRECTION('ref_axis',(0.,0.951056516295154,0.309016994374947)) ;
#21105=DIRECTION('center_axis',(-1.,0.,0.)) ;
#21106=DIRECTION('ref_axis',(0.,-0.951056516295154,-0.309016994374947)) ;
#21107=DIRECTION('',(-1.,0.,0.)) ;
#21108=DIRECTION('center_axis',(-1.,0.,0.)) ;
#21109=DIRECTION('ref_axis',(0.,-0.951056516295154,-0.309016994374947)) ;
#21110=DIRECTION('',(-1.,0.,0.)) ;
#21111=DIRECTION('center_axis',(-1.,0.,0.)) ;
#21112=DIRECTION('ref_axis',(0.,-0.951056516295154,-0.309016994374947)) ;
#21113=DIRECTION('center_axis',(1.,0.,0.)) ;
#21114=DIRECTION('ref_axis',(0.,0.978147600733806,0.207911690817759)) ;
#21115=DIRECTION('center_axis',(1.,0.,0.)) ;
#21116=DIRECTION('ref_axis',(0.,0.978147600733806,0.207911690817759)) ;
#21117=DIRECTION('center_axis',(1.,0.,0.)) ;
#21118=DIRECTION('ref_axis',(0.,0.978147600733806,0.207911690817759)) ;
#21119=DIRECTION('center_axis',(1.,0.,0.)) ;
#21120=DIRECTION('ref_axis',(0.,0.978147600733806,0.207911690817759)) ;
#21121=DIRECTION('center_axis',(1.,0.,0.)) ;
#21122=DIRECTION('ref_axis',(0.,0.978147600733806,0.207911690817759)) ;
#21123=DIRECTION('center_axis',(1.,0.,0.)) ;
#21124=DIRECTION('ref_axis',(0.,0.978147600733806,0.207911690817759)) ;
#21125=DIRECTION('center_axis',(1.,0.,0.)) ;
#21126=DIRECTION('ref_axis',(0.,0.978147600733806,0.207911690817759)) ;
#21127=DIRECTION('center_axis',(1.,0.,0.)) ;
#21128=DIRECTION('ref_axis',(0.,0.978147600733806,0.207911690817759)) ;
#21129=DIRECTION('center_axis',(-1.,0.,0.)) ;
#21130=DIRECTION('ref_axis',(0.,-0.978147600733806,-0.207911690817759)) ;
#21131=DIRECTION('',(-1.,0.,0.)) ;
#21132=DIRECTION('center_axis',(-1.,0.,0.)) ;
#21133=DIRECTION('ref_axis',(0.,-0.978147600733806,-0.207911690817759)) ;
#21134=DIRECTION('',(-1.,0.,0.)) ;
#21135=DIRECTION('center_axis',(-1.,0.,0.)) ;
#21136=DIRECTION('ref_axis',(0.,-0.978147600733806,-0.207911690817759)) ;
#21137=DIRECTION('center_axis',(1.,0.,0.)) ;
#21138=DIRECTION('ref_axis',(0.,0.994521895368273,0.104528463267653)) ;
#21139=DIRECTION('center_axis',(1.,0.,0.)) ;
#21140=DIRECTION('ref_axis',(0.,0.994521895368273,0.104528463267653)) ;
#21141=DIRECTION('center_axis',(1.,0.,0.)) ;
#21142=DIRECTION('ref_axis',(0.,0.994521895368273,0.104528463267653)) ;
#21143=DIRECTION('center_axis',(1.,0.,0.)) ;
#21144=DIRECTION('ref_axis',(0.,0.994521895368273,0.104528463267653)) ;
#21145=DIRECTION('center_axis',(1.,0.,0.)) ;
#21146=DIRECTION('ref_axis',(0.,0.994521895368273,0.104528463267653)) ;
#21147=DIRECTION('center_axis',(1.,0.,0.)) ;
#21148=DIRECTION('ref_axis',(0.,0.994521895368273,0.104528463267653)) ;
#21149=DIRECTION('center_axis',(1.,0.,0.)) ;
#21150=DIRECTION('ref_axis',(0.,0.994521895368273,0.104528463267653)) ;
#21151=DIRECTION('center_axis',(1.,0.,0.)) ;
#21152=DIRECTION('ref_axis',(0.,0.994521895368273,0.104528463267653)) ;
#21153=DIRECTION('center_axis',(-1.,0.,0.)) ;
#21154=DIRECTION('ref_axis',(0.,-0.994521895368273,-0.104528463267653)) ;
#21155=DIRECTION('',(-1.,0.,0.)) ;
#21156=DIRECTION('center_axis',(-1.,0.,0.)) ;
#21157=DIRECTION('ref_axis',(0.,-0.994521895368273,-0.104528463267653)) ;
#21158=DIRECTION('',(-1.,0.,0.)) ;
#21159=DIRECTION('center_axis',(-1.,0.,0.)) ;
#21160=DIRECTION('ref_axis',(0.,-0.994521895368273,-0.104528463267653)) ;
#21161=DIRECTION('center_axis',(1.,0.,0.)) ;
#21162=DIRECTION('ref_axis',(0.,1.,-6.12323399573677E-17)) ;
#21163=DIRECTION('center_axis',(1.,0.,0.)) ;
#21164=DIRECTION('ref_axis',(0.,1.,-6.12323399573677E-17)) ;
#21165=DIRECTION('center_axis',(1.,0.,0.)) ;
#21166=DIRECTION('ref_axis',(0.,1.,-6.12323399573677E-17)) ;
#21167=DIRECTION('center_axis',(1.,0.,0.)) ;
#21168=DIRECTION('ref_axis',(0.,1.,-6.12323399573677E-17)) ;
#21169=DIRECTION('center_axis',(1.,0.,0.)) ;
#21170=DIRECTION('ref_axis',(0.,1.,-6.12323399573677E-17)) ;
#21171=DIRECTION('center_axis',(1.,0.,0.)) ;
#21172=DIRECTION('ref_axis',(0.,1.,-6.12323399573677E-17)) ;
#21173=DIRECTION('center_axis',(1.,0.,0.)) ;
#21174=DIRECTION('ref_axis',(0.,1.,-6.12323399573677E-17)) ;
#21175=DIRECTION('center_axis',(1.,0.,0.)) ;
#21176=DIRECTION('ref_axis',(0.,1.,-6.12323399573677E-17)) ;
#21177=DIRECTION('center_axis',(-1.,0.,0.)) ;
#21178=DIRECTION('ref_axis',(0.,-1.,6.12323399573677E-17)) ;
#21179=DIRECTION('',(-1.,0.,0.)) ;
#21180=DIRECTION('center_axis',(-1.,0.,0.)) ;
#21181=DIRECTION('ref_axis',(0.,-1.,6.12323399573677E-17)) ;
#21182=DIRECTION('',(-1.,0.,0.)) ;
#21183=DIRECTION('center_axis',(-1.,0.,0.)) ;
#21184=DIRECTION('ref_axis',(0.,-1.,6.12323399573677E-17)) ;
#21185=DIRECTION('center_axis',(1.,0.,0.)) ;
#21186=DIRECTION('ref_axis',(0.,0.994521895368273,-0.104528463267653)) ;
#21187=DIRECTION('center_axis',(1.,0.,0.)) ;
#21188=DIRECTION('ref_axis',(0.,0.994521895368273,-0.104528463267653)) ;
#21189=DIRECTION('center_axis',(1.,0.,0.)) ;
#21190=DIRECTION('ref_axis',(0.,0.994521895368273,-0.104528463267653)) ;
#21191=DIRECTION('center_axis',(1.,0.,0.)) ;
#21192=DIRECTION('ref_axis',(0.,0.994521895368273,-0.104528463267653)) ;
#21193=DIRECTION('center_axis',(1.,0.,0.)) ;
#21194=DIRECTION('ref_axis',(0.,0.994521895368273,-0.104528463267653)) ;
#21195=DIRECTION('center_axis',(1.,0.,0.)) ;
#21196=DIRECTION('ref_axis',(0.,0.994521895368273,-0.104528463267653)) ;
#21197=DIRECTION('center_axis',(1.,0.,0.)) ;
#21198=DIRECTION('ref_axis',(0.,0.994521895368273,-0.104528463267653)) ;
#21199=DIRECTION('center_axis',(1.,0.,0.)) ;
#21200=DIRECTION('ref_axis',(0.,0.994521895368273,-0.104528463267653)) ;
#21201=DIRECTION('center_axis',(-1.,0.,0.)) ;
#21202=DIRECTION('ref_axis',(0.,-0.994521895368273,0.104528463267653)) ;
#21203=DIRECTION('',(-1.,0.,0.)) ;
#21204=DIRECTION('center_axis',(-1.,0.,0.)) ;
#21205=DIRECTION('ref_axis',(0.,-0.994521895368273,0.104528463267653)) ;
#21206=DIRECTION('',(-1.,0.,0.)) ;
#21207=DIRECTION('center_axis',(-1.,0.,0.)) ;
#21208=DIRECTION('ref_axis',(0.,-0.994521895368273,0.104528463267653)) ;
#21209=DIRECTION('center_axis',(1.,0.,0.)) ;
#21210=DIRECTION('ref_axis',(0.,0.978147600733806,-0.207911690817759)) ;
#21211=DIRECTION('center_axis',(1.,0.,0.)) ;
#21212=DIRECTION('ref_axis',(0.,0.978147600733806,-0.207911690817759)) ;
#21213=DIRECTION('center_axis',(1.,0.,0.)) ;
#21214=DIRECTION('ref_axis',(0.,0.978147600733806,-0.207911690817759)) ;
#21215=DIRECTION('center_axis',(1.,0.,0.)) ;
#21216=DIRECTION('ref_axis',(0.,0.978147600733806,-0.207911690817759)) ;
#21217=DIRECTION('center_axis',(1.,0.,0.)) ;
#21218=DIRECTION('ref_axis',(0.,0.978147600733806,-0.207911690817759)) ;
#21219=DIRECTION('center_axis',(1.,0.,0.)) ;
#21220=DIRECTION('ref_axis',(0.,0.978147600733806,-0.207911690817759)) ;
#21221=DIRECTION('center_axis',(1.,0.,0.)) ;
#21222=DIRECTION('ref_axis',(0.,0.978147600733806,-0.207911690817759)) ;
#21223=DIRECTION('center_axis',(1.,0.,0.)) ;
#21224=DIRECTION('ref_axis',(0.,0.978147600733806,-0.207911690817759)) ;
#21225=DIRECTION('center_axis',(-1.,0.,0.)) ;
#21226=DIRECTION('ref_axis',(0.,-0.978147600733806,0.207911690817759)) ;
#21227=DIRECTION('',(-1.,0.,0.)) ;
#21228=DIRECTION('center_axis',(-1.,0.,0.)) ;
#21229=DIRECTION('ref_axis',(0.,-0.978147600733806,0.207911690817759)) ;
#21230=DIRECTION('',(-1.,0.,0.)) ;
#21231=DIRECTION('center_axis',(-1.,0.,0.)) ;
#21232=DIRECTION('ref_axis',(0.,-0.978147600733806,0.207911690817759)) ;
#21233=DIRECTION('center_axis',(1.,0.,0.)) ;
#21234=DIRECTION('ref_axis',(0.,0.951056516295154,-0.309016994374947)) ;
#21235=DIRECTION('center_axis',(1.,0.,0.)) ;
#21236=DIRECTION('ref_axis',(0.,0.951056516295154,-0.309016994374947)) ;
#21237=DIRECTION('center_axis',(1.,0.,0.)) ;
#21238=DIRECTION('ref_axis',(0.,0.951056516295154,-0.309016994374947)) ;
#21239=DIRECTION('center_axis',(1.,0.,0.)) ;
#21240=DIRECTION('ref_axis',(0.,0.951056516295154,-0.309016994374947)) ;
#21241=DIRECTION('center_axis',(1.,0.,0.)) ;
#21242=DIRECTION('ref_axis',(0.,0.951056516295154,-0.309016994374947)) ;
#21243=DIRECTION('center_axis',(1.,0.,0.)) ;
#21244=DIRECTION('ref_axis',(0.,0.951056516295154,-0.309016994374947)) ;
#21245=DIRECTION('center_axis',(1.,0.,0.)) ;
#21246=DIRECTION('ref_axis',(0.,0.951056516295154,-0.309016994374947)) ;
#21247=DIRECTION('center_axis',(1.,0.,0.)) ;
#21248=DIRECTION('ref_axis',(0.,0.951056516295154,-0.309016994374947)) ;
#21249=DIRECTION('center_axis',(-1.,0.,0.)) ;
#21250=DIRECTION('ref_axis',(0.,-0.951056516295154,0.309016994374947)) ;
#21251=DIRECTION('',(-1.,0.,0.)) ;
#21252=DIRECTION('center_axis',(-1.,0.,0.)) ;
#21253=DIRECTION('ref_axis',(0.,-0.951056516295154,0.309016994374947)) ;
#21254=DIRECTION('',(-1.,0.,0.)) ;
#21255=DIRECTION('center_axis',(-1.,0.,0.)) ;
#21256=DIRECTION('ref_axis',(0.,-0.951056516295154,0.309016994374947)) ;
#21257=DIRECTION('center_axis',(1.,0.,0.)) ;
#21258=DIRECTION('ref_axis',(0.,0.913545457642601,-0.4067366430758)) ;
#21259=DIRECTION('center_axis',(1.,0.,0.)) ;
#21260=DIRECTION('ref_axis',(0.,0.913545457642601,-0.4067366430758)) ;
#21261=DIRECTION('center_axis',(1.,0.,0.)) ;
#21262=DIRECTION('ref_axis',(0.,0.913545457642601,-0.4067366430758)) ;
#21263=DIRECTION('center_axis',(1.,0.,0.)) ;
#21264=DIRECTION('ref_axis',(0.,0.913545457642601,-0.4067366430758)) ;
#21265=DIRECTION('center_axis',(1.,0.,0.)) ;
#21266=DIRECTION('ref_axis',(0.,0.913545457642601,-0.4067366430758)) ;
#21267=DIRECTION('center_axis',(1.,0.,0.)) ;
#21268=DIRECTION('ref_axis',(0.,0.913545457642601,-0.4067366430758)) ;
#21269=DIRECTION('center_axis',(1.,0.,0.)) ;
#21270=DIRECTION('ref_axis',(0.,0.913545457642601,-0.4067366430758)) ;
#21271=DIRECTION('center_axis',(1.,0.,0.)) ;
#21272=DIRECTION('ref_axis',(0.,0.913545457642601,-0.4067366430758)) ;
#21273=DIRECTION('center_axis',(-1.,0.,0.)) ;
#21274=DIRECTION('ref_axis',(0.,-0.913545457642601,0.4067366430758)) ;
#21275=DIRECTION('',(-1.,0.,0.)) ;
#21276=DIRECTION('center_axis',(-1.,0.,0.)) ;
#21277=DIRECTION('ref_axis',(0.,-0.913545457642601,0.4067366430758)) ;
#21278=DIRECTION('',(-1.,0.,0.)) ;
#21279=DIRECTION('center_axis',(-1.,0.,0.)) ;
#21280=DIRECTION('ref_axis',(0.,-0.913545457642601,0.4067366430758)) ;
#21281=DIRECTION('center_axis',(1.,0.,0.)) ;
#21282=DIRECTION('ref_axis',(0.,0.866025403784439,-0.5)) ;
#21283=DIRECTION('center_axis',(1.,0.,0.)) ;
#21284=DIRECTION('ref_axis',(0.,0.866025403784439,-0.5)) ;
#21285=DIRECTION('center_axis',(1.,0.,0.)) ;
#21286=DIRECTION('ref_axis',(0.,0.866025403784439,-0.5)) ;
#21287=DIRECTION('center_axis',(1.,0.,0.)) ;
#21288=DIRECTION('ref_axis',(0.,0.866025403784439,-0.5)) ;
#21289=DIRECTION('center_axis',(1.,0.,0.)) ;
#21290=DIRECTION('ref_axis',(0.,0.866025403784439,-0.5)) ;
#21291=DIRECTION('center_axis',(1.,0.,0.)) ;
#21292=DIRECTION('ref_axis',(0.,0.866025403784439,-0.5)) ;
#21293=DIRECTION('center_axis',(1.,0.,0.)) ;
#21294=DIRECTION('ref_axis',(0.,0.866025403784439,-0.5)) ;
#21295=DIRECTION('center_axis',(1.,0.,0.)) ;
#21296=DIRECTION('ref_axis',(0.,0.866025403784439,-0.5)) ;
#21297=DIRECTION('center_axis',(-1.,0.,0.)) ;
#21298=DIRECTION('ref_axis',(0.,-0.866025403784439,0.5)) ;
#21299=DIRECTION('',(-1.,0.,0.)) ;
#21300=DIRECTION('center_axis',(-1.,0.,0.)) ;
#21301=DIRECTION('ref_axis',(0.,-0.866025403784439,0.5)) ;
#21302=DIRECTION('',(-1.,0.,0.)) ;
#21303=DIRECTION('center_axis',(-1.,0.,0.)) ;
#21304=DIRECTION('ref_axis',(0.,-0.866025403784439,0.5)) ;
#21305=DIRECTION('center_axis',(1.,0.,0.)) ;
#21306=DIRECTION('ref_axis',(0.,0.587785252292473,-0.809016994374947)) ;
#21307=DIRECTION('center_axis',(1.,0.,0.)) ;
#21308=DIRECTION('ref_axis',(0.,0.587785252292473,-0.809016994374947)) ;
#21309=DIRECTION('center_axis',(1.,0.,0.)) ;
#21310=DIRECTION('ref_axis',(0.,0.587785252292473,-0.809016994374947)) ;
#21311=DIRECTION('center_axis',(1.,0.,0.)) ;
#21312=DIRECTION('ref_axis',(0.,0.587785252292473,-0.809016994374947)) ;
#21313=DIRECTION('center_axis',(1.,0.,0.)) ;
#21314=DIRECTION('ref_axis',(0.,0.587785252292473,-0.809016994374947)) ;
#21315=DIRECTION('center_axis',(1.,0.,0.)) ;
#21316=DIRECTION('ref_axis',(0.,0.587785252292473,-0.809016994374947)) ;
#21317=DIRECTION('center_axis',(1.,0.,0.)) ;
#21318=DIRECTION('ref_axis',(0.,0.587785252292473,-0.809016994374947)) ;
#21319=DIRECTION('center_axis',(1.,0.,0.)) ;
#21320=DIRECTION('ref_axis',(0.,0.587785252292473,-0.809016994374947)) ;
#21321=DIRECTION('center_axis',(-1.,0.,0.)) ;
#21322=DIRECTION('ref_axis',(0.,-0.587785252292473,0.809016994374947)) ;
#21323=DIRECTION('',(-1.,0.,0.)) ;
#21324=DIRECTION('center_axis',(-1.,0.,0.)) ;
#21325=DIRECTION('ref_axis',(0.,-0.587785252292473,0.809016994374947)) ;
#21326=DIRECTION('',(-1.,0.,0.)) ;
#21327=DIRECTION('center_axis',(-1.,0.,0.)) ;
#21328=DIRECTION('ref_axis',(0.,-0.587785252292473,0.809016994374947)) ;
#21329=DIRECTION('center_axis',(1.,0.,0.)) ;
#21330=DIRECTION('ref_axis',(0.,0.669130606358858,-0.743144825477394)) ;
#21331=DIRECTION('center_axis',(1.,0.,0.)) ;
#21332=DIRECTION('ref_axis',(0.,0.669130606358858,-0.743144825477394)) ;
#21333=DIRECTION('center_axis',(1.,0.,0.)) ;
#21334=DIRECTION('ref_axis',(0.,0.669130606358858,-0.743144825477394)) ;
#21335=DIRECTION('center_axis',(1.,0.,0.)) ;
#21336=DIRECTION('ref_axis',(0.,0.669130606358858,-0.743144825477394)) ;
#21337=DIRECTION('center_axis',(1.,0.,0.)) ;
#21338=DIRECTION('ref_axis',(0.,0.669130606358858,-0.743144825477394)) ;
#21339=DIRECTION('center_axis',(1.,0.,0.)) ;
#21340=DIRECTION('ref_axis',(0.,0.669130606358858,-0.743144825477394)) ;
#21341=DIRECTION('center_axis',(1.,0.,0.)) ;
#21342=DIRECTION('ref_axis',(0.,0.669130606358858,-0.743144825477394)) ;
#21343=DIRECTION('center_axis',(1.,0.,0.)) ;
#21344=DIRECTION('ref_axis',(0.,0.669130606358858,-0.743144825477394)) ;
#21345=DIRECTION('center_axis',(-1.,0.,0.)) ;
#21346=DIRECTION('ref_axis',(0.,-0.669130606358858,0.743144825477394)) ;
#21347=DIRECTION('',(-1.,0.,0.)) ;
#21348=DIRECTION('center_axis',(-1.,0.,0.)) ;
#21349=DIRECTION('ref_axis',(0.,-0.669130606358858,0.743144825477394)) ;
#21350=DIRECTION('',(-1.,0.,0.)) ;
#21351=DIRECTION('center_axis',(-1.,0.,0.)) ;
#21352=DIRECTION('ref_axis',(0.,-0.669130606358858,0.743144825477394)) ;
#21353=DIRECTION('center_axis',(1.,0.,0.)) ;
#21354=DIRECTION('ref_axis',(0.,0.743144825477394,-0.669130606358859)) ;
#21355=DIRECTION('center_axis',(1.,0.,0.)) ;
#21356=DIRECTION('ref_axis',(0.,0.743144825477394,-0.669130606358859)) ;
#21357=DIRECTION('center_axis',(1.,0.,0.)) ;
#21358=DIRECTION('ref_axis',(0.,0.743144825477394,-0.669130606358859)) ;
#21359=DIRECTION('center_axis',(1.,0.,0.)) ;
#21360=DIRECTION('ref_axis',(0.,0.743144825477394,-0.669130606358859)) ;
#21361=DIRECTION('center_axis',(1.,0.,0.)) ;
#21362=DIRECTION('ref_axis',(0.,0.743144825477394,-0.669130606358859)) ;
#21363=DIRECTION('center_axis',(1.,0.,0.)) ;
#21364=DIRECTION('ref_axis',(0.,0.743144825477394,-0.669130606358859)) ;
#21365=DIRECTION('center_axis',(1.,0.,0.)) ;
#21366=DIRECTION('ref_axis',(0.,0.743144825477394,-0.669130606358859)) ;
#21367=DIRECTION('center_axis',(1.,0.,0.)) ;
#21368=DIRECTION('ref_axis',(0.,0.743144825477394,-0.669130606358859)) ;
#21369=DIRECTION('center_axis',(-1.,0.,0.)) ;
#21370=DIRECTION('ref_axis',(0.,-0.743144825477394,0.669130606358859)) ;
#21371=DIRECTION('',(-1.,0.,0.)) ;
#21372=DIRECTION('center_axis',(-1.,0.,0.)) ;
#21373=DIRECTION('ref_axis',(0.,-0.743144825477394,0.669130606358859)) ;
#21374=DIRECTION('',(-1.,0.,0.)) ;
#21375=DIRECTION('center_axis',(-1.,0.,0.)) ;
#21376=DIRECTION('ref_axis',(0.,-0.743144825477394,0.669130606358859)) ;
#21377=DIRECTION('center_axis',(1.,0.,0.)) ;
#21378=DIRECTION('ref_axis',(0.,0.809016994374947,-0.587785252292473)) ;
#21379=DIRECTION('center_axis',(1.,0.,0.)) ;
#21380=DIRECTION('ref_axis',(0.,0.809016994374947,-0.587785252292473)) ;
#21381=DIRECTION('center_axis',(1.,0.,0.)) ;
#21382=DIRECTION('ref_axis',(0.,0.809016994374947,-0.587785252292473)) ;
#21383=DIRECTION('center_axis',(1.,0.,0.)) ;
#21384=DIRECTION('ref_axis',(0.,0.809016994374947,-0.587785252292473)) ;
#21385=DIRECTION('center_axis',(1.,0.,0.)) ;
#21386=DIRECTION('ref_axis',(0.,0.809016994374947,-0.587785252292473)) ;
#21387=DIRECTION('center_axis',(1.,0.,0.)) ;
#21388=DIRECTION('ref_axis',(0.,0.809016994374947,-0.587785252292473)) ;
#21389=DIRECTION('center_axis',(1.,0.,0.)) ;
#21390=DIRECTION('ref_axis',(0.,0.809016994374947,-0.587785252292473)) ;
#21391=DIRECTION('center_axis',(1.,0.,0.)) ;
#21392=DIRECTION('ref_axis',(0.,0.809016994374947,-0.587785252292473)) ;
#21393=DIRECTION('center_axis',(-1.,0.,0.)) ;
#21394=DIRECTION('ref_axis',(0.,-0.809016994374947,0.587785252292473)) ;
#21395=DIRECTION('',(-1.,0.,0.)) ;
#21396=DIRECTION('center_axis',(-1.,0.,0.)) ;
#21397=DIRECTION('ref_axis',(0.,-0.809016994374947,0.587785252292473)) ;
#21398=DIRECTION('',(-1.,0.,0.)) ;
#21399=DIRECTION('center_axis',(-1.,0.,0.)) ;
#21400=DIRECTION('ref_axis',(0.,-0.809016994374947,0.587785252292473)) ;
#21401=DIRECTION('center_axis',(1.,0.,0.)) ;
#21402=DIRECTION('ref_axis',(0.,0.5,-0.866025403784439)) ;
#21403=DIRECTION('center_axis',(1.,0.,0.)) ;
#21404=DIRECTION('ref_axis',(0.,0.5,-0.866025403784439)) ;
#21405=DIRECTION('center_axis',(1.,0.,0.)) ;
#21406=DIRECTION('ref_axis',(0.,0.5,-0.866025403784439)) ;
#21407=DIRECTION('center_axis',(1.,0.,0.)) ;
#21408=DIRECTION('ref_axis',(0.,0.5,-0.866025403784439)) ;
#21409=DIRECTION('center_axis',(1.,0.,0.)) ;
#21410=DIRECTION('ref_axis',(0.,0.5,-0.866025403784439)) ;
#21411=DIRECTION('center_axis',(1.,0.,0.)) ;
#21412=DIRECTION('ref_axis',(0.,0.5,-0.866025403784439)) ;
#21413=DIRECTION('center_axis',(1.,0.,0.)) ;
#21414=DIRECTION('ref_axis',(0.,0.5,-0.866025403784439)) ;
#21415=DIRECTION('center_axis',(1.,0.,0.)) ;
#21416=DIRECTION('ref_axis',(0.,0.5,-0.866025403784439)) ;
#21417=DIRECTION('center_axis',(-1.,0.,0.)) ;
#21418=DIRECTION('ref_axis',(0.,-0.5,0.866025403784439)) ;
#21419=DIRECTION('',(-1.,0.,0.)) ;
#21420=DIRECTION('center_axis',(-1.,0.,0.)) ;
#21421=DIRECTION('ref_axis',(0.,-0.5,0.866025403784439)) ;
#21422=DIRECTION('',(-1.,0.,0.)) ;
#21423=DIRECTION('center_axis',(-1.,0.,0.)) ;
#21424=DIRECTION('ref_axis',(0.,-0.5,0.866025403784439)) ;
#21425=DIRECTION('center_axis',(1.,0.,0.)) ;
#21426=DIRECTION('ref_axis',(0.,0.4067366430758,-0.913545457642601)) ;
#21427=DIRECTION('center_axis',(1.,0.,0.)) ;
#21428=DIRECTION('ref_axis',(0.,0.4067366430758,-0.913545457642601)) ;
#21429=DIRECTION('center_axis',(1.,0.,0.)) ;
#21430=DIRECTION('ref_axis',(0.,0.4067366430758,-0.913545457642601)) ;
#21431=DIRECTION('center_axis',(1.,0.,0.)) ;
#21432=DIRECTION('ref_axis',(0.,0.4067366430758,-0.913545457642601)) ;
#21433=DIRECTION('center_axis',(1.,0.,0.)) ;
#21434=DIRECTION('ref_axis',(0.,0.4067366430758,-0.913545457642601)) ;
#21435=DIRECTION('center_axis',(1.,0.,0.)) ;
#21436=DIRECTION('ref_axis',(0.,0.4067366430758,-0.913545457642601)) ;
#21437=DIRECTION('center_axis',(1.,0.,0.)) ;
#21438=DIRECTION('ref_axis',(0.,0.4067366430758,-0.913545457642601)) ;
#21439=DIRECTION('center_axis',(1.,0.,0.)) ;
#21440=DIRECTION('ref_axis',(0.,0.4067366430758,-0.913545457642601)) ;
#21441=DIRECTION('center_axis',(-1.,0.,0.)) ;
#21442=DIRECTION('ref_axis',(0.,-0.4067366430758,0.913545457642601)) ;
#21443=DIRECTION('',(-1.,0.,0.)) ;
#21444=DIRECTION('center_axis',(-1.,0.,0.)) ;
#21445=DIRECTION('ref_axis',(0.,-0.4067366430758,0.913545457642601)) ;
#21446=DIRECTION('',(-1.,0.,0.)) ;
#21447=DIRECTION('center_axis',(-1.,0.,0.)) ;
#21448=DIRECTION('ref_axis',(0.,-0.4067366430758,0.913545457642601)) ;
#21449=DIRECTION('center_axis',(1.,0.,0.)) ;
#21450=DIRECTION('ref_axis',(0.,0.309016994374947,-0.951056516295154)) ;
#21451=DIRECTION('center_axis',(1.,0.,0.)) ;
#21452=DIRECTION('ref_axis',(0.,0.309016994374947,-0.951056516295154)) ;
#21453=DIRECTION('center_axis',(1.,0.,0.)) ;
#21454=DIRECTION('ref_axis',(0.,0.309016994374947,-0.951056516295154)) ;
#21455=DIRECTION('center_axis',(1.,0.,0.)) ;
#21456=DIRECTION('ref_axis',(0.,0.309016994374947,-0.951056516295154)) ;
#21457=DIRECTION('center_axis',(1.,0.,0.)) ;
#21458=DIRECTION('ref_axis',(0.,0.309016994374947,-0.951056516295154)) ;
#21459=DIRECTION('center_axis',(1.,0.,0.)) ;
#21460=DIRECTION('ref_axis',(0.,0.309016994374947,-0.951056516295154)) ;
#21461=DIRECTION('center_axis',(1.,0.,0.)) ;
#21462=DIRECTION('ref_axis',(0.,0.309016994374947,-0.951056516295154)) ;
#21463=DIRECTION('center_axis',(1.,0.,0.)) ;
#21464=DIRECTION('ref_axis',(0.,0.309016994374947,-0.951056516295154)) ;
#21465=DIRECTION('center_axis',(-1.,0.,0.)) ;
#21466=DIRECTION('ref_axis',(0.,-0.309016994374947,0.951056516295154)) ;
#21467=DIRECTION('',(-1.,0.,0.)) ;
#21468=DIRECTION('center_axis',(-1.,0.,0.)) ;
#21469=DIRECTION('ref_axis',(0.,-0.309016994374947,0.951056516295154)) ;
#21470=DIRECTION('',(-1.,0.,0.)) ;
#21471=DIRECTION('center_axis',(-1.,0.,0.)) ;
#21472=DIRECTION('ref_axis',(0.,-0.309016994374947,0.951056516295154)) ;
#21473=DIRECTION('center_axis',(1.,0.,0.)) ;
#21474=DIRECTION('ref_axis',(0.,0.207911690817759,-0.978147600733806)) ;
#21475=DIRECTION('center_axis',(1.,0.,0.)) ;
#21476=DIRECTION('ref_axis',(0.,0.207911690817759,-0.978147600733806)) ;
#21477=DIRECTION('center_axis',(1.,0.,0.)) ;
#21478=DIRECTION('ref_axis',(0.,0.207911690817759,-0.978147600733806)) ;
#21479=DIRECTION('center_axis',(1.,0.,0.)) ;
#21480=DIRECTION('ref_axis',(0.,0.207911690817759,-0.978147600733806)) ;
#21481=DIRECTION('center_axis',(1.,0.,0.)) ;
#21482=DIRECTION('ref_axis',(0.,0.207911690817759,-0.978147600733806)) ;
#21483=DIRECTION('center_axis',(1.,0.,0.)) ;
#21484=DIRECTION('ref_axis',(0.,0.207911690817759,-0.978147600733806)) ;
#21485=DIRECTION('center_axis',(1.,0.,0.)) ;
#21486=DIRECTION('ref_axis',(0.,0.207911690817759,-0.978147600733806)) ;
#21487=DIRECTION('center_axis',(1.,0.,0.)) ;
#21488=DIRECTION('ref_axis',(0.,0.207911690817759,-0.978147600733806)) ;
#21489=DIRECTION('center_axis',(-1.,0.,0.)) ;
#21490=DIRECTION('ref_axis',(0.,-0.207911690817759,0.978147600733806)) ;
#21491=DIRECTION('',(-1.,0.,0.)) ;
#21492=DIRECTION('center_axis',(-1.,0.,0.)) ;
#21493=DIRECTION('ref_axis',(0.,-0.207911690817759,0.978147600733806)) ;
#21494=DIRECTION('',(-1.,0.,0.)) ;
#21495=DIRECTION('center_axis',(-1.,0.,0.)) ;
#21496=DIRECTION('ref_axis',(0.,-0.207911690817759,0.978147600733806)) ;
#21497=DIRECTION('center_axis',(1.,0.,0.)) ;
#21498=DIRECTION('ref_axis',(0.,-1.,-6.12323399573677E-17)) ;
#51949=CARTESIAN_POINT('',(0.,0.,0.)) ;
#51950=CARTESIAN_POINT('Origin',(0.,24.5,5.)) ;
#51951=CARTESIAN_POINT('',(0.,19.3649167310371,5.)) ;
#51952=CARTESIAN_POINT('',(45.,19.3649167310371,5.)) ;
#51953=CARTESIAN_POINT('',(45.,19.3649167310371,5.)) ;
#51954=CARTESIAN_POINT('',(0.,24.5,5.)) ;
#51955=CARTESIAN_POINT('',(0.,12.25,5.)) ;
#51956=CARTESIAN_POINT('',(45.,24.5,5.)) ;
#51957=CARTESIAN_POINT('',(0.,24.5,5.)) ;
#51958=CARTESIAN_POINT('',(45.,31.,5.)) ;
#51959=CARTESIAN_POINT('Origin',(0.,24.5,-5.)) ;
#51960=CARTESIAN_POINT('',(0.,24.5,-5.)) ;
#51961=CARTESIAN_POINT('',(0.,24.5,-2.5)) ;
#51962=CARTESIAN_POINT('',(45.,24.5,-5.)) ;
#51963=CARTESIAN_POINT('',(0.,24.5,-5.)) ;
#51964=CARTESIAN_POINT('',(45.,24.5,-2.5)) ;
#51965=CARTESIAN_POINT('Origin',(0.,14.5,-5.)) ;
#51966=CARTESIAN_POINT('',(45.,19.3649167310371,-5.)) ;
#51967=CARTESIAN_POINT('',(0.,19.3649167310371,-5.)) ;
#51968=CARTESIAN_POINT('',(45.,19.3649167310371,-5.)) ;
#51969=CARTESIAN_POINT('',(45.,26.,-5.)) ;
#51970=CARTESIAN_POINT('',(0.,7.25,-5.)) ;
#51971=CARTESIAN_POINT('Origin',(0.,0.,0.)) ;
#51972=CARTESIAN_POINT('',(0.,-4.89858719658941E-15,40.)) ;
#51973=CARTESIAN_POINT('Origin',(0.,0.,0.)) ;
#51974=CARTESIAN_POINT('Origin',(0.,0.,0.)) ;
#51975=CARTESIAN_POINT('Origin',(45.,0.,0.)) ;
#51976=CARTESIAN_POINT('',(30.5,46.5121833407376,7.8801919949714)) ;
#51977=CARTESIAN_POINT('',(2.5,46.5121833407376,7.8801919949714)) ;
#51978=CARTESIAN_POINT('',(30.5,46.5121833407376,7.8801919949714)) ;
#51979=CARTESIAN_POINT('',(30.5,46.670828298707,6.87854715129665)) ;
#51980=CARTESIAN_POINT('Origin',(30.5,0.,0.)) ;
#51981=CARTESIAN_POINT('',(2.5,46.6708282987069,6.87854715129677)) ;
#51982=CARTESIAN_POINT('',(30.5,46.6708282987069,6.87854715129677)) ;
#51983=CARTESIAN_POINT('Origin',(2.49999999999999,0.,0.)) ;
#51984=CARTESIAN_POINT('Origin',(45.,0.,0.)) ;
#51985=CARTESIAN_POINT('',(30.5,45.6961566547982,11.7192957117799)) ;
#51986=CARTESIAN_POINT('',(30.5,45.4336803742586,12.6988705265355)) ;
#51987=CARTESIAN_POINT('Origin',(30.5,0.,0.)) ;
#51988=CARTESIAN_POINT('',(2.5,45.6961566547981,11.71929571178)) ;
#51989=CARTESIAN_POINT('',(30.5,45.6961566547981,11.71929571178)) ;
#51990=CARTESIAN_POINT('',(2.5,45.4336803742586,12.6988705265355)) ;
#51991=CARTESIAN_POINT('Origin',(2.49999999999999,0.,0.)) ;
#51992=CARTESIAN_POINT('',(30.5,45.4336803742586,12.6988705265355)) ;
#51993=CARTESIAN_POINT('Origin',(45.,0.,0.)) ;
#51994=CARTESIAN_POINT('',(30.5,44.2208283560439,16.4316452160247)) ;
#51995=CARTESIAN_POINT('',(30.5,43.8573964979903,17.3784175752014)) ;
#51996=CARTESIAN_POINT('Origin',(30.5,0.,0.)) ;
#51997=CARTESIAN_POINT('',(2.5,44.2208283560438,16.4316452160248)) ;
#51998=CARTESIAN_POINT('',(30.5,44.2208283560438,16.4316452160248)) ;
#51999=CARTESIAN_POINT('',(2.5,43.8573964979903,17.3784175752014)) ;
#52000=CARTESIAN_POINT('Origin',(2.49999999999999,0.,0.)) ;
#52001=CARTESIAN_POINT('',(30.5,43.8573964979903,17.3784175752014)) ;
#52002=CARTESIAN_POINT('Origin',(45.,0.,0.)) ;
#52003=CARTESIAN_POINT('',(30.5,42.2610074080175,20.9639661767398)) ;
#52004=CARTESIAN_POINT('',(30.5,41.8006018079398,21.8675630442457)) ;
#52005=CARTESIAN_POINT('Origin',(30.5,0.,0.)) ;
#52006=CARTESIAN_POINT('',(2.5,42.2610074080174,20.9639661767399)) ;
#52007=CARTESIAN_POINT('',(30.5,42.2610074080174,20.9639661767399)) ;
#52008=CARTESIAN_POINT('',(2.5,41.8006018079398,21.8675630442457)) ;
#52009=CARTESIAN_POINT('Origin',(2.49999999999999,0.,0.)) ;
#52010=CARTESIAN_POINT('',(30.5,41.8006018079398,21.8675630442457)) ;
#52011=CARTESIAN_POINT('Origin',(45.,0.,0.)) ;
#52012=CARTESIAN_POINT('',(30.5,29.2924107235056,36.9788493466935)) ;
#52013=CARTESIAN_POINT('',(2.5,29.2924107235056,36.9788493466935)) ;
#52014=CARTESIAN_POINT('',(30.5,29.2924107235056,36.9788493466935)) ;
#52015=CARTESIAN_POINT('',(30.5,30.0805381247129,36.3406363610723)) ;
#52016=CARTESIAN_POINT('Origin',(30.5,0.,0.)) ;
#52017=CARTESIAN_POINT('',(2.5,30.0805381247128,36.3406363610724)) ;
#52018=CARTESIAN_POINT('',(30.5,30.0805381247128,36.3406363610724)) ;
#52019=CARTESIAN_POINT('Origin',(2.49999999999999,0.,0.)) ;
#52020=CARTESIAN_POINT('Origin',(45.,0.,0.)) ;
#52021=CARTESIAN_POINT('',(30.5,32.9972861282627,33.7143846624785)) ;
#52022=CARTESIAN_POINT('',(2.5,32.9972861282627,33.7143846624785)) ;
#52023=CARTESIAN_POINT('',(30.5,32.9972861282627,33.7143846624785)) ;
#52024=CARTESIAN_POINT('',(30.5,33.7143846624786,32.9972861282625)) ;
#52025=CARTESIAN_POINT('Origin',(30.5,0.,0.)) ;
#52026=CARTESIAN_POINT('',(2.5,33.7143846624785,32.9972861282626)) ;
#52027=CARTESIAN_POINT('',(30.5,33.7143846624785,32.9972861282626)) ;
#52028=CARTESIAN_POINT('Origin',(2.49999999999999,0.,0.)) ;
#52029=CARTESIAN_POINT('Origin',(45.,0.,0.)) ;
#52030=CARTESIAN_POINT('',(30.5,36.3406363610724,30.0805381247128)) ;
#52031=CARTESIAN_POINT('',(2.5,36.3406363610724,30.0805381247128)) ;
#52032=CARTESIAN_POINT('',(30.5,36.3406363610724,30.0805381247128)) ;
#52033=CARTESIAN_POINT('',(30.5,36.9788493466936,29.2924107235055)) ;
#52034=CARTESIAN_POINT('Origin',(30.5,0.,0.)) ;
#52035=CARTESIAN_POINT('',(2.5,36.9788493466935,29.2924107235055)) ;
#52036=CARTESIAN_POINT('',(30.5,36.9788493466935,29.2924107235055)) ;
#52037=CARTESIAN_POINT('Origin',(2.49999999999999,0.,0.)) ;
#52038=CARTESIAN_POINT('Origin',(45.,0.,0.)) ;
#52039=CARTESIAN_POINT('',(30.5,39.8381660191445,25.2666015370306)) ;
#52040=CARTESIAN_POINT('',(30.5,39.2858309771432,26.1171229164955)) ;
#52041=CARTESIAN_POINT('Origin',(30.5,0.,0.)) ;
#52042=CARTESIAN_POINT('',(2.5,39.8381660191444,25.2666015370307)) ;
#52043=CARTESIAN_POINT('',(30.5,39.8381660191444,25.2666015370307)) ;
#52044=CARTESIAN_POINT('',(2.5,39.2858309771432,26.1171229164955)) ;
#52045=CARTESIAN_POINT('Origin',(2.49999999999999,0.,0.)) ;
#52046=CARTESIAN_POINT('',(30.5,39.2858309771432,26.1171229164955)) ;
#52047=CARTESIAN_POINT('Origin',(45.,0.,0.)) ;
#52048=CARTESIAN_POINT('',(30.5,26.1171229164956,39.2858309771432)) ;
#52049=CARTESIAN_POINT('',(30.5,25.2666015370307,39.8381660191445)) ;
#52050=CARTESIAN_POINT('Origin',(30.5,0.,0.)) ;
#52051=CARTESIAN_POINT('',(2.5,26.1171229164954,39.2858309771432)) ;
#52052=CARTESIAN_POINT('',(30.5,26.1171229164954,39.2858309771432)) ;
#52053=CARTESIAN_POINT('',(2.5,25.2666015370307,39.8381660191445)) ;
#52054=CARTESIAN_POINT('Origin',(2.49999999999999,0.,0.)) ;
#52055=CARTESIAN_POINT('',(30.5,25.2666015370307,39.8381660191445)) ;
#52056=CARTESIAN_POINT('Origin',(45.,0.,0.)) ;
#52057=CARTESIAN_POINT('',(30.5,21.8675630442458,41.8006018079397)) ;
#52058=CARTESIAN_POINT('',(30.5,20.9639661767399,42.2610074080174)) ;
#52059=CARTESIAN_POINT('Origin',(30.5,0.,0.)) ;
#52060=CARTESIAN_POINT('',(2.5,21.8675630442456,41.8006018079398)) ;
#52061=CARTESIAN_POINT('',(30.5,21.8675630442456,41.8006018079398)) ;
#52062=CARTESIAN_POINT('',(2.5,20.9639661767399,42.2610074080174)) ;
#52063=CARTESIAN_POINT('Origin',(2.49999999999999,0.,0.)) ;
#52064=CARTESIAN_POINT('',(30.5,20.9639661767399,42.2610074080174)) ;
#52065=CARTESIAN_POINT('Origin',(45.,0.,0.)) ;
#52066=CARTESIAN_POINT('',(30.5,17.3784175752015,43.8573964979902)) ;
#52067=CARTESIAN_POINT('',(30.5,16.4316452160248,44.2208283560438)) ;
#52068=CARTESIAN_POINT('Origin',(30.5,0.,0.)) ;
#52069=CARTESIAN_POINT('',(2.5,17.3784175752014,43.8573964979902)) ;
#52070=CARTESIAN_POINT('',(30.5,17.3784175752014,43.8573964979902)) ;
#52071=CARTESIAN_POINT('',(2.5,16.4316452160248,44.2208283560438)) ;
#52072=CARTESIAN_POINT('Origin',(2.49999999999999,0.,0.)) ;
#52073=CARTESIAN_POINT('',(30.5,16.4316452160248,44.2208283560438)) ;
#52074=CARTESIAN_POINT('Origin',(45.,0.,0.)) ;
#52075=CARTESIAN_POINT('',(30.5,12.6988705265356,45.4336803742585)) ;
#52076=CARTESIAN_POINT('',(30.5,11.7192957117801,45.6961566547981)) ;
#52077=CARTESIAN_POINT('Origin',(30.5,0.,0.)) ;
#52078=CARTESIAN_POINT('',(2.5,12.6988705265355,45.4336803742585)) ;
#52079=CARTESIAN_POINT('',(30.5,12.6988705265355,45.4336803742585)) ;
#52080=CARTESIAN_POINT('',(2.5,11.7192957117801,45.6961566547981)) ;
#52081=CARTESIAN_POINT('Origin',(2.49999999999999,0.,0.)) ;
#52082=CARTESIAN_POINT('',(30.5,11.7192957117801,45.6961566547981)) ;
#52083=CARTESIAN_POINT('Origin',(45.,0.,0.)) ;
#52084=CARTESIAN_POINT('',(30.5,7.88019199497154,46.5121833407376)) ;
#52085=CARTESIAN_POINT('',(30.5,6.87854715129677,46.670828298707)) ;
#52086=CARTESIAN_POINT('Origin',(30.5,0.,0.)) ;
#52087=CARTESIAN_POINT('',(2.5,7.8801919949714,46.5121833407375)) ;
#52088=CARTESIAN_POINT('',(30.5,7.8801919949714,46.5121833407375)) ;
#52089=CARTESIAN_POINT('',(2.5,6.87854715129677,46.670828298707)) ;
#52090=CARTESIAN_POINT('Origin',(2.49999999999999,0.,0.)) ;
#52091=CARTESIAN_POINT('',(30.5,6.87854715129677,46.670828298707)) ;
#52092=CARTESIAN_POINT('Origin',(45.,0.,0.)) ;
#52093=CARTESIAN_POINT('',(30.5,2.97517643087433,47.0810890932354)) ;
#52094=CARTESIAN_POINT('',(30.5,1.96243578879535,47.1341645812764)) ;
#52095=CARTESIAN_POINT('Origin',(30.5,0.,0.)) ;
#52096=CARTESIAN_POINT('',(2.5,2.9751764308742,47.0810890932354)) ;
#52097=CARTESIAN_POINT('',(30.5,2.9751764308742,47.0810890932354)) ;
#52098=CARTESIAN_POINT('',(2.5,1.96243578879535,47.1341645812764)) ;
#52099=CARTESIAN_POINT('Origin',(2.49999999999999,0.,0.)) ;
#52100=CARTESIAN_POINT('',(30.5,1.96243578879535,47.1341645812764)) ;
#52101=CARTESIAN_POINT('Origin',(45.,0.,0.)) ;
#52102=CARTESIAN_POINT('',(30.5,-1.96243578879522,47.1341645812764)) ;
#52103=CARTESIAN_POINT('',(30.5,-2.97517643087417,47.0810890932354)) ;
#52104=CARTESIAN_POINT('Origin',(30.5,0.,0.)) ;
#52105=CARTESIAN_POINT('',(2.5,-1.96243578879535,47.1341645812764)) ;
#52106=CARTESIAN_POINT('',(30.5,-1.96243578879535,47.1341645812764)) ;
#52107=CARTESIAN_POINT('',(2.5,-2.97517643087417,47.0810890932354)) ;
#52108=CARTESIAN_POINT('Origin',(2.49999999999999,0.,0.)) ;
#52109=CARTESIAN_POINT('',(30.5,-2.97517643087417,47.0810890932354)) ;
#52110=CARTESIAN_POINT('Origin',(45.,0.,0.)) ;
#52111=CARTESIAN_POINT('',(30.5,-6.87854715129661,46.670828298707)) ;
#52112=CARTESIAN_POINT('',(30.5,-7.88019199497139,46.5121833407376)) ;
#52113=CARTESIAN_POINT('Origin',(30.5,0.,0.)) ;
#52114=CARTESIAN_POINT('',(2.5,-6.87854715129673,46.6708282987069)) ;
#52115=CARTESIAN_POINT('',(30.5,-6.87854715129673,46.6708282987069)) ;
#52116=CARTESIAN_POINT('',(2.5,-7.88019199497139,46.5121833407376)) ;
#52117=CARTESIAN_POINT('Origin',(2.49999999999999,0.,0.)) ;
#52118=CARTESIAN_POINT('',(30.5,-7.88019199497139,46.5121833407376)) ;
#52119=CARTESIAN_POINT('Origin',(45.,0.,0.)) ;
#52120=CARTESIAN_POINT('',(30.5,-11.7192957117799,45.6961566547982)) ;
#52121=CARTESIAN_POINT('',(30.5,-12.6988705265355,45.4336803742586)) ;
#52122=CARTESIAN_POINT('Origin',(30.5,0.,0.)) ;
#52123=CARTESIAN_POINT('',(2.5,-11.71929571178,45.6961566547981)) ;
#52124=CARTESIAN_POINT('',(30.5,-11.71929571178,45.6961566547981)) ;
#52125=CARTESIAN_POINT('',(2.5,-12.6988705265355,45.4336803742586)) ;
#52126=CARTESIAN_POINT('Origin',(2.49999999999999,0.,0.)) ;
#52127=CARTESIAN_POINT('',(30.5,-12.6988705265355,45.4336803742586)) ;
#52128=CARTESIAN_POINT('Origin',(45.,0.,0.)) ;
#52129=CARTESIAN_POINT('',(30.5,-16.4316452160246,44.2208283560439)) ;
#52130=CARTESIAN_POINT('',(30.5,-17.3784175752014,43.8573964979903)) ;
#52131=CARTESIAN_POINT('Origin',(30.5,0.,0.)) ;
#52132=CARTESIAN_POINT('',(2.5,-16.4316452160247,44.2208283560438)) ;
#52133=CARTESIAN_POINT('',(30.5,-16.4316452160247,44.2208283560438)) ;
#52134=CARTESIAN_POINT('',(2.5,-17.3784175752014,43.8573964979903)) ;
#52135=CARTESIAN_POINT('Origin',(2.49999999999999,0.,0.)) ;
#52136=CARTESIAN_POINT('',(30.5,-17.3784175752014,43.8573964979903)) ;
#52137=CARTESIAN_POINT('Origin',(45.,0.,0.)) ;
#52138=CARTESIAN_POINT('',(30.5,-20.9639661767398,42.2610074080175)) ;
#52139=CARTESIAN_POINT('',(30.5,-21.8675630442457,41.8006018079398)) ;
#52140=CARTESIAN_POINT('Origin',(30.5,0.,0.)) ;
#52141=CARTESIAN_POINT('',(2.5,-20.9639661767399,42.2610074080174)) ;
#52142=CARTESIAN_POINT('',(30.5,-20.9639661767399,42.2610074080174)) ;
#52143=CARTESIAN_POINT('',(2.5,-21.8675630442457,41.8006018079398)) ;
#52144=CARTESIAN_POINT('Origin',(2.49999999999999,0.,0.)) ;
#52145=CARTESIAN_POINT('',(30.5,-21.8675630442457,41.8006018079398)) ;
#52146=CARTESIAN_POINT('Origin',(45.,0.,0.)) ;
#52147=CARTESIAN_POINT('',(30.5,-25.2666015370306,39.8381660191445)) ;
#52148=CARTESIAN_POINT('',(30.5,-26.1171229164955,39.2858309771432)) ;
#52149=CARTESIAN_POINT('Origin',(30.5,0.,0.)) ;
#52150=CARTESIAN_POINT('',(2.5,-25.2666015370307,39.8381660191444)) ;
#52151=CARTESIAN_POINT('',(30.5,-25.2666015370307,39.8381660191444)) ;
#52152=CARTESIAN_POINT('',(2.5,-26.1171229164955,39.2858309771432)) ;
#52153=CARTESIAN_POINT('Origin',(2.49999999999999,0.,0.)) ;
#52154=CARTESIAN_POINT('',(30.5,-26.1171229164955,39.2858309771432)) ;
#52155=CARTESIAN_POINT('Origin',(45.,0.,0.)) ;
#52156=CARTESIAN_POINT('',(30.5,-33.7143846624785,32.9972861282626)) ;
#52157=CARTESIAN_POINT('',(2.5,-33.7143846624785,32.9972861282626)) ;
#52158=CARTESIAN_POINT('',(30.5,-33.7143846624785,32.9972861282626)) ;
#52159=CARTESIAN_POINT('',(30.5,-32.9972861282625,33.7143846624786)) ;
#52160=CARTESIAN_POINT('Origin',(30.5,0.,0.)) ;
#52161=CARTESIAN_POINT('',(2.5,-32.9972861282626,33.7143846624785)) ;
#52162=CARTESIAN_POINT('',(30.5,-32.9972861282626,33.7143846624785)) ;
#52163=CARTESIAN_POINT('Origin',(2.49999999999999,0.,0.)) ;
#52164=CARTESIAN_POINT('Origin',(45.,0.,0.)) ;
#52165=CARTESIAN_POINT('',(30.5,-29.2924107235054,36.9788493466936)) ;
#52166=CARTESIAN_POINT('',(30.5,-30.0805381247128,36.3406363610724)) ;
#52167=CARTESIAN_POINT('Origin',(30.5,0.,0.)) ;
#52168=CARTESIAN_POINT('',(2.5,-29.2924107235055,36.9788493466935)) ;
#52169=CARTESIAN_POINT('',(30.5,-29.2924107235055,36.9788493466935)) ;
#52170=CARTESIAN_POINT('',(2.5,-30.0805381247128,36.3406363610724)) ;
#52171=CARTESIAN_POINT('Origin',(2.49999999999999,0.,0.)) ;
#52172=CARTESIAN_POINT('',(30.5,-30.0805381247128,36.3406363610724)) ;
#52173=CARTESIAN_POINT('Origin',(45.,0.,0.)) ;
#52174=CARTESIAN_POINT('',(30.5,-36.3406363610723,30.0805381247129)) ;
#52175=CARTESIAN_POINT('',(30.5,-36.9788493466935,29.2924107235056)) ;
#52176=CARTESIAN_POINT('Origin',(30.5,0.,0.)) ;
#52177=CARTESIAN_POINT('',(2.5,-36.3406363610724,30.0805381247128)) ;
#52178=CARTESIAN_POINT('',(30.5,-36.3406363610724,30.0805381247128)) ;
#52179=CARTESIAN_POINT('',(2.5,-36.9788493466935,29.2924107235056)) ;
#52180=CARTESIAN_POINT('Origin',(2.49999999999999,0.,0.)) ;
#52181=CARTESIAN_POINT('',(30.5,-36.9788493466935,29.2924107235056)) ;
#52182=CARTESIAN_POINT('Origin',(45.,0.,0.)) ;
#52183=CARTESIAN_POINT('',(30.5,-39.2858309771431,26.1171229164956)) ;
#52184=CARTESIAN_POINT('',(30.5,-39.8381660191444,25.2666015370307)) ;
#52185=CARTESIAN_POINT('Origin',(30.5,0.,0.)) ;
#52186=CARTESIAN_POINT('',(2.5,-39.2858309771432,26.1171229164955)) ;
#52187=CARTESIAN_POINT('',(30.5,-39.2858309771432,26.1171229164955)) ;
#52188=CARTESIAN_POINT('',(2.5,-39.8381660191444,25.2666015370307)) ;
#52189=CARTESIAN_POINT('Origin',(2.49999999999999,0.,0.)) ;
#52190=CARTESIAN_POINT('',(30.5,-39.8381660191444,25.2666015370307)) ;
#52191=CARTESIAN_POINT('Origin',(45.,0.,0.)) ;
#52192=CARTESIAN_POINT('',(30.5,-41.8006018079397,21.8675630442458)) ;
#52193=CARTESIAN_POINT('',(30.5,-42.2610074080174,20.9639661767399)) ;
#52194=CARTESIAN_POINT('Origin',(30.5,0.,0.)) ;
#52195=CARTESIAN_POINT('',(2.5,-41.8006018079397,21.8675630442457)) ;
#52196=CARTESIAN_POINT('',(30.5,-41.8006018079397,21.8675630442457)) ;
#52197=CARTESIAN_POINT('',(2.5,-42.2610074080174,20.9639661767399)) ;
#52198=CARTESIAN_POINT('Origin',(2.49999999999999,0.,0.)) ;
#52199=CARTESIAN_POINT('',(30.5,-42.2610074080174,20.9639661767399)) ;
#52200=CARTESIAN_POINT('Origin',(45.,0.,0.)) ;
#52201=CARTESIAN_POINT('',(30.5,-43.8573964979902,17.3784175752015)) ;
#52202=CARTESIAN_POINT('',(30.5,-44.2208283560438,16.4316452160248)) ;
#52203=CARTESIAN_POINT('Origin',(30.5,0.,0.)) ;
#52204=CARTESIAN_POINT('',(2.5,-43.8573964979902,17.3784175752014)) ;
#52205=CARTESIAN_POINT('',(30.5,-43.8573964979902,17.3784175752014)) ;
#52206=CARTESIAN_POINT('',(2.5,-44.2208283560438,16.4316452160248)) ;
#52207=CARTESIAN_POINT('Origin',(2.49999999999999,0.,0.)) ;
#52208=CARTESIAN_POINT('',(30.5,-44.2208283560438,16.4316452160248)) ;
#52209=CARTESIAN_POINT('Origin',(45.,0.,0.)) ;
#52210=CARTESIAN_POINT('',(30.5,-45.4336803742585,12.6988705265356)) ;
#52211=CARTESIAN_POINT('',(30.5,-45.6961566547981,11.7192957117801)) ;
#52212=CARTESIAN_POINT('Origin',(30.5,0.,0.)) ;
#52213=CARTESIAN_POINT('',(2.5,-45.4336803742585,12.6988705265355)) ;
#52214=CARTESIAN_POINT('',(30.5,-45.4336803742585,12.6988705265355)) ;
#52215=CARTESIAN_POINT('',(2.5,-45.6961566547981,11.7192957117801)) ;
#52216=CARTESIAN_POINT('Origin',(2.49999999999999,0.,0.)) ;
#52217=CARTESIAN_POINT('',(30.5,-45.6961566547981,11.7192957117801)) ;
#52218=CARTESIAN_POINT('Origin',(45.,0.,0.)) ;
#52219=CARTESIAN_POINT('',(30.5,-46.5121833407376,7.88019199497153)) ;
#52220=CARTESIAN_POINT('',(30.5,-46.670828298707,6.87854715129678)) ;
#52221=CARTESIAN_POINT('Origin',(30.5,0.,0.)) ;
#52222=CARTESIAN_POINT('',(2.5,-46.5121833407376,7.88019199497139)) ;
#52223=CARTESIAN_POINT('',(30.5,-46.5121833407376,7.88019199497139)) ;
#52224=CARTESIAN_POINT('',(2.5,-46.670828298707,6.87854715129678)) ;
#52225=CARTESIAN_POINT('Origin',(2.49999999999999,0.,0.)) ;
#52226=CARTESIAN_POINT('',(30.5,-46.670828298707,6.87854715129678)) ;
#52227=CARTESIAN_POINT('Origin',(45.,0.,0.)) ;
#52228=CARTESIAN_POINT('',(30.5,-47.0810890932354,2.97517643087434)) ;
#52229=CARTESIAN_POINT('',(30.5,-47.1341645812764,1.96243578879536)) ;
#52230=CARTESIAN_POINT('Origin',(30.5,0.,0.)) ;
#52231=CARTESIAN_POINT('',(2.5,-47.0810890932354,2.97517643087421)) ;
#52232=CARTESIAN_POINT('',(30.5,-47.0810890932354,2.97517643087421)) ;
#52233=CARTESIAN_POINT('',(2.5,-47.1341645812764,1.96243578879536)) ;
#52234=CARTESIAN_POINT('Origin',(2.49999999999999,0.,0.)) ;
#52235=CARTESIAN_POINT('',(30.5,-47.1341645812764,1.96243578879536)) ;
#52236=CARTESIAN_POINT('Origin',(45.,0.,0.)) ;
#52237=CARTESIAN_POINT('',(30.5,-47.1341645812764,-1.96243578879522)) ;
#52238=CARTESIAN_POINT('',(30.5,-47.0810890932354,-2.97517643087418)) ;
#52239=CARTESIAN_POINT('Origin',(30.5,0.,0.)) ;
#52240=CARTESIAN_POINT('',(2.5,-47.1341645812764,-1.96243578879534)) ;
#52241=CARTESIAN_POINT('',(30.5,-47.1341645812764,-1.96243578879534)) ;
#52242=CARTESIAN_POINT('',(2.5,-47.0810890932354,-2.97517643087418)) ;
#52243=CARTESIAN_POINT('Origin',(2.49999999999999,0.,0.)) ;
#52244=CARTESIAN_POINT('',(30.5,-47.0810890932354,-2.97517643087418)) ;
#52245=CARTESIAN_POINT('Origin',(45.,0.,0.)) ;
#52246=CARTESIAN_POINT('',(30.5,-46.670828298707,-6.87854715129663)) ;
#52247=CARTESIAN_POINT('',(30.5,-46.5121833407376,-7.88019199497139)) ;
#52248=CARTESIAN_POINT('Origin',(30.5,0.,0.)) ;
#52249=CARTESIAN_POINT('',(2.5,-46.6708282987069,-6.87854715129675)) ;
#52250=CARTESIAN_POINT('',(30.5,-46.6708282987069,-6.87854715129675)) ;
#52251=CARTESIAN_POINT('',(2.5,-46.5121833407376,-7.88019199497139)) ;
#52252=CARTESIAN_POINT('Origin',(2.49999999999999,0.,0.)) ;
#52253=CARTESIAN_POINT('',(30.5,-46.5121833407376,-7.88019199497139)) ;
#52254=CARTESIAN_POINT('Origin',(45.,0.,0.)) ;
#52255=CARTESIAN_POINT('',(30.5,-45.6961566547982,-11.7192957117799)) ;
#52256=CARTESIAN_POINT('',(30.5,-45.4336803742586,-12.6988705265355)) ;
#52257=CARTESIAN_POINT('Origin',(30.5,0.,0.)) ;
#52258=CARTESIAN_POINT('',(2.5,-45.6961566547981,-11.71929571178)) ;
#52259=CARTESIAN_POINT('',(30.5,-45.6961566547981,-11.71929571178)) ;
#52260=CARTESIAN_POINT('',(2.5,-45.4336803742586,-12.6988705265355)) ;
#52261=CARTESIAN_POINT('Origin',(2.49999999999999,0.,0.)) ;
#52262=CARTESIAN_POINT('',(30.5,-45.4336803742586,-12.6988705265355)) ;
#52263=CARTESIAN_POINT('Origin',(45.,0.,0.)) ;
#52264=CARTESIAN_POINT('',(30.5,-20.9639661767399,-42.2610074080174)) ;
#52265=CARTESIAN_POINT('',(2.5,-20.9639661767399,-42.2610074080174)) ;
#52266=CARTESIAN_POINT('',(30.5,-20.9639661767399,-42.2610074080174)) ;
#52267=CARTESIAN_POINT('',(30.5,-21.8675630442458,-41.8006018079397)) ;
#52268=CARTESIAN_POINT('Origin',(30.5,0.,0.)) ;
#52269=CARTESIAN_POINT('',(2.5,-21.8675630442457,-41.8006018079397)) ;
#52270=CARTESIAN_POINT('',(30.5,-21.8675630442457,-41.8006018079397)) ;
#52271=CARTESIAN_POINT('Origin',(2.49999999999999,0.,0.)) ;
#52272=CARTESIAN_POINT('Origin',(45.,0.,0.)) ;
#52273=CARTESIAN_POINT('',(30.5,-25.2666015370308,-39.8381660191444)) ;
#52274=CARTESIAN_POINT('',(2.5,-25.2666015370308,-39.8381660191444)) ;
#52275=CARTESIAN_POINT('',(30.5,-25.2666015370308,-39.8381660191444)) ;
#52276=CARTESIAN_POINT('',(30.5,-26.1171229164956,-39.2858309771431)) ;
#52277=CARTESIAN_POINT('Origin',(30.5,0.,0.)) ;
#52278=CARTESIAN_POINT('',(2.5,-26.1171229164955,-39.2858309771432)) ;
#52279=CARTESIAN_POINT('',(30.5,-26.1171229164955,-39.2858309771432)) ;
#52280=CARTESIAN_POINT('Origin',(2.49999999999999,0.,0.)) ;
#52281=CARTESIAN_POINT('Origin',(45.,0.,0.)) ;
#52282=CARTESIAN_POINT('',(30.5,-29.2924107235056,-36.9788493466935)) ;
#52283=CARTESIAN_POINT('',(2.5,-29.2924107235056,-36.9788493466935)) ;
#52284=CARTESIAN_POINT('',(30.5,-29.2924107235056,-36.9788493466935)) ;
#52285=CARTESIAN_POINT('',(30.5,-30.0805381247129,-36.3406363610723)) ;
#52286=CARTESIAN_POINT('Origin',(30.5,0.,0.)) ;
#52287=CARTESIAN_POINT('',(2.5,-30.0805381247128,-36.3406363610724)) ;
#52288=CARTESIAN_POINT('',(30.5,-30.0805381247128,-36.3406363610724)) ;
#52289=CARTESIAN_POINT('Origin',(2.49999999999999,0.,0.)) ;
#52290=CARTESIAN_POINT('Origin',(45.,0.,0.)) ;
#52291=CARTESIAN_POINT('',(30.5,-32.9972861282627,-33.7143846624785)) ;
#52292=CARTESIAN_POINT('',(2.5,-32.9972861282627,-33.7143846624785)) ;
#52293=CARTESIAN_POINT('',(30.5,-32.9972861282627,-33.7143846624785)) ;
#52294=CARTESIAN_POINT('',(30.5,-33.7143846624786,-32.9972861282625)) ;
#52295=CARTESIAN_POINT('Origin',(30.5,0.,0.)) ;
#52296=CARTESIAN_POINT('',(2.5,-33.7143846624785,-32.9972861282626)) ;
#52297=CARTESIAN_POINT('',(30.5,-33.7143846624785,-32.9972861282626)) ;
#52298=CARTESIAN_POINT('Origin',(2.49999999999999,0.,0.)) ;
#52299=CARTESIAN_POINT('Origin',(45.,0.,0.)) ;
#52300=CARTESIAN_POINT('',(30.5,-36.3406363610724,-30.0805381247128)) ;
#52301=CARTESIAN_POINT('',(2.5,-36.3406363610724,-30.0805381247128)) ;
#52302=CARTESIAN_POINT('',(30.5,-36.3406363610724,-30.0805381247128)) ;
#52303=CARTESIAN_POINT('',(30.5,-36.9788493466936,-29.2924107235055)) ;
#52304=CARTESIAN_POINT('Origin',(30.5,0.,0.)) ;
#52305=CARTESIAN_POINT('',(2.5,-36.9788493466935,-29.2924107235055)) ;
#52306=CARTESIAN_POINT('',(30.5,-36.9788493466935,-29.2924107235055)) ;
#52307=CARTESIAN_POINT('Origin',(2.49999999999999,0.,0.)) ;
#52308=CARTESIAN_POINT('Origin',(45.,0.,0.)) ;
#52309=CARTESIAN_POINT('',(30.5,-39.2858309771432,-26.1171229164955)) ;
#52310=CARTESIAN_POINT('',(2.5,-39.2858309771432,-26.1171229164955)) ;
#52311=CARTESIAN_POINT('',(30.5,-39.2858309771432,-26.1171229164955)) ;
#52312=CARTESIAN_POINT('',(30.5,-39.8381660191445,-25.2666015370306)) ;
#52313=CARTESIAN_POINT('Origin',(30.5,0.,0.)) ;
#52314=CARTESIAN_POINT('',(2.5,-39.8381660191444,-25.2666015370307)) ;
#52315=CARTESIAN_POINT('',(30.5,-39.8381660191444,-25.2666015370307)) ;
#52316=CARTESIAN_POINT('Origin',(2.49999999999999,0.,0.)) ;
#52317=CARTESIAN_POINT('Origin',(45.,0.,0.)) ;
#52318=CARTESIAN_POINT('',(30.5,-41.8006018079398,-21.8675630442457)) ;
#52319=CARTESIAN_POINT('',(2.5,-41.8006018079398,-21.8675630442457)) ;
#52320=CARTESIAN_POINT('',(30.5,-41.8006018079398,-21.8675630442457)) ;
#52321=CARTESIAN_POINT('',(30.5,-42.2610074080175,-20.9639661767398)) ;
#52322=CARTESIAN_POINT('Origin',(30.5,0.,0.)) ;
#52323=CARTESIAN_POINT('',(2.5,-42.2610074080174,-20.9639661767399)) ;
#52324=CARTESIAN_POINT('',(30.5,-42.2610074080174,-20.9639661767399)) ;
#52325=CARTESIAN_POINT('Origin',(2.49999999999999,0.,0.)) ;
#52326=CARTESIAN_POINT('Origin',(45.,0.,0.)) ;
#52327=CARTESIAN_POINT('',(30.5,-44.2208283560439,-16.4316452160247)) ;
#52328=CARTESIAN_POINT('',(30.5,-43.8573964979903,-17.3784175752014)) ;
#52329=CARTESIAN_POINT('Origin',(30.5,0.,0.)) ;
#52330=CARTESIAN_POINT('',(2.5,-44.2208283560438,-16.4316452160248)) ;
#52331=CARTESIAN_POINT('',(30.5,-44.2208283560438,-16.4316452160248)) ;
#52332=CARTESIAN_POINT('',(2.5,-43.8573964979903,-17.3784175752014)) ;
#52333=CARTESIAN_POINT('Origin',(2.49999999999999,0.,0.)) ;
#52334=CARTESIAN_POINT('',(30.5,-43.8573964979903,-17.3784175752014)) ;
#52335=CARTESIAN_POINT('Origin',(45.,0.,0.)) ;
#52336=CARTESIAN_POINT('',(30.5,-17.3784175752015,-43.8573964979902)) ;
#52337=CARTESIAN_POINT('',(30.5,-16.4316452160248,-44.2208283560438)) ;
#52338=CARTESIAN_POINT('Origin',(30.5,0.,0.)) ;
#52339=CARTESIAN_POINT('',(2.5,-17.3784175752014,-43.8573964979902)) ;
#52340=CARTESIAN_POINT('',(30.5,-17.3784175752014,-43.8573964979902)) ;
#52341=CARTESIAN_POINT('',(2.5,-16.4316452160248,-44.2208283560438)) ;
#52342=CARTESIAN_POINT('Origin',(2.49999999999999,0.,0.)) ;
#52343=CARTESIAN_POINT('',(30.5,-16.4316452160248,-44.2208283560438)) ;
#52344=CARTESIAN_POINT('Origin',(45.,0.,0.)) ;
#52345=CARTESIAN_POINT('',(30.5,-12.6988705265356,-45.4336803742585)) ;
#52346=CARTESIAN_POINT('',(30.5,-11.7192957117801,-45.6961566547981)) ;
#52347=CARTESIAN_POINT('Origin',(30.5,0.,0.)) ;
#52348=CARTESIAN_POINT('',(2.5,-12.6988705265355,-45.4336803742585)) ;
#52349=CARTESIAN_POINT('',(30.5,-12.6988705265355,-45.4336803742585)) ;
#52350=CARTESIAN_POINT('',(2.5,-11.7192957117801,-45.6961566547981)) ;
#52351=CARTESIAN_POINT('Origin',(2.49999999999999,0.,0.)) ;
#52352=CARTESIAN_POINT('',(30.5,-11.7192957117801,-45.6961566547981)) ;
#52353=CARTESIAN_POINT('Origin',(45.,0.,0.)) ;
#52354=CARTESIAN_POINT('',(30.5,-7.88019199497155,-46.5121833407376)) ;
#52355=CARTESIAN_POINT('',(30.5,-6.87854715129677,-46.670828298707)) ;
#52356=CARTESIAN_POINT('Origin',(30.5,0.,0.)) ;
#52357=CARTESIAN_POINT('',(2.5,-7.88019199497142,-46.5121833407375)) ;
#52358=CARTESIAN_POINT('',(30.5,-7.88019199497142,-46.5121833407375)) ;
#52359=CARTESIAN_POINT('',(2.5,-6.87854715129677,-46.670828298707)) ;
#52360=CARTESIAN_POINT('Origin',(2.49999999999999,0.,0.)) ;
#52361=CARTESIAN_POINT('',(30.5,-6.87854715129677,-46.670828298707)) ;
#52362=CARTESIAN_POINT('Origin',(45.,0.,0.)) ;
#52363=CARTESIAN_POINT('',(30.5,-2.97517643087433,-47.0810890932354)) ;
#52364=CARTESIAN_POINT('',(30.5,-1.96243578879536,-47.1341645812764)) ;
#52365=CARTESIAN_POINT('Origin',(30.5,0.,0.)) ;
#52366=CARTESIAN_POINT('',(2.5,-2.97517643087419,-47.0810890932354)) ;
#52367=CARTESIAN_POINT('',(30.5,-2.97517643087419,-47.0810890932354)) ;
#52368=CARTESIAN_POINT('',(2.5,-1.96243578879536,-47.1341645812764)) ;
#52369=CARTESIAN_POINT('Origin',(2.49999999999999,0.,0.)) ;
#52370=CARTESIAN_POINT('',(30.5,-1.96243578879536,-47.1341645812764)) ;
#52371=CARTESIAN_POINT('Origin',(45.,0.,0.)) ;
#52372=CARTESIAN_POINT('',(30.5,1.96243578879521,-47.1341645812764)) ;
#52373=CARTESIAN_POINT('',(30.5,2.9751764308742,-47.0810890932354)) ;
#52374=CARTESIAN_POINT('Origin',(30.5,0.,0.)) ;
#52375=CARTESIAN_POINT('',(2.5,1.96243578879534,-47.1341645812764)) ;
#52376=CARTESIAN_POINT('',(30.5,1.96243578879534,-47.1341645812764)) ;
#52377=CARTESIAN_POINT('',(2.5,2.9751764308742,-47.0810890932354)) ;
#52378=CARTESIAN_POINT('Origin',(2.49999999999999,0.,0.)) ;
#52379=CARTESIAN_POINT('',(30.5,2.9751764308742,-47.0810890932354)) ;
#52380=CARTESIAN_POINT('Origin',(45.,0.,0.)) ;
#52381=CARTESIAN_POINT('',(30.5,6.87854715129665,-46.670828298707)) ;
#52382=CARTESIAN_POINT('',(30.5,7.88019199497141,-46.5121833407376)) ;
#52383=CARTESIAN_POINT('Origin',(30.5,0.,0.)) ;
#52384=CARTESIAN_POINT('',(2.5,6.87854715129677,-46.6708282987069)) ;
#52385=CARTESIAN_POINT('',(30.5,6.87854715129677,-46.6708282987069)) ;
#52386=CARTESIAN_POINT('',(2.5,7.88019199497141,-46.5121833407376)) ;
#52387=CARTESIAN_POINT('Origin',(2.49999999999999,0.,0.)) ;
#52388=CARTESIAN_POINT('',(30.5,7.88019199497141,-46.5121833407376)) ;
#52389=CARTESIAN_POINT('Origin',(45.,0.,0.)) ;
#52390=CARTESIAN_POINT('',(30.5,11.7192957117799,-45.6961566547982)) ;
#52391=CARTESIAN_POINT('',(30.5,12.6988705265355,-45.4336803742586)) ;
#52392=CARTESIAN_POINT('Origin',(30.5,0.,0.)) ;
#52393=CARTESIAN_POINT('',(2.5,11.71929571178,-45.6961566547981)) ;
#52394=CARTESIAN_POINT('',(30.5,11.71929571178,-45.6961566547981)) ;
#52395=CARTESIAN_POINT('',(2.5,12.6988705265355,-45.4336803742586)) ;
#52396=CARTESIAN_POINT('Origin',(2.49999999999999,0.,0.)) ;
#52397=CARTESIAN_POINT('',(30.5,12.6988705265355,-45.4336803742586)) ;
#52398=CARTESIAN_POINT('Origin',(45.,0.,0.)) ;
#52399=CARTESIAN_POINT('',(30.5,16.4316452160247,-44.2208283560439)) ;
#52400=CARTESIAN_POINT('',(30.5,17.3784175752014,-43.8573964979903)) ;
#52401=CARTESIAN_POINT('Origin',(30.5,0.,0.)) ;
#52402=CARTESIAN_POINT('',(2.5,16.4316452160248,-44.2208283560438)) ;
#52403=CARTESIAN_POINT('',(30.5,16.4316452160248,-44.2208283560438)) ;
#52404=CARTESIAN_POINT('',(2.5,17.3784175752014,-43.8573964979903)) ;
#52405=CARTESIAN_POINT('Origin',(2.49999999999999,0.,0.)) ;
#52406=CARTESIAN_POINT('',(30.5,17.3784175752014,-43.8573964979903)) ;
#52407=CARTESIAN_POINT('Origin',(45.,0.,0.)) ;
#52408=CARTESIAN_POINT('',(30.5,20.9639661767398,-42.2610074080175)) ;
#52409=CARTESIAN_POINT('',(30.5,21.8675630442457,-41.8006018079398)) ;
#52410=CARTESIAN_POINT('Origin',(30.5,0.,0.)) ;
#52411=CARTESIAN_POINT('',(2.5,20.9639661767399,-42.2610074080174)) ;
#52412=CARTESIAN_POINT('',(30.5,20.9639661767399,-42.2610074080174)) ;
#52413=CARTESIAN_POINT('',(2.5,21.8675630442457,-41.8006018079398)) ;
#52414=CARTESIAN_POINT('Origin',(2.49999999999999,0.,0.)) ;
#52415=CARTESIAN_POINT('',(30.5,21.8675630442457,-41.8006018079398)) ;
#52416=CARTESIAN_POINT('Origin',(45.,0.,0.)) ;
#52417=CARTESIAN_POINT('',(30.5,25.2666015370306,-39.8381660191445)) ;
#52418=CARTESIAN_POINT('',(30.5,26.1171229164955,-39.2858309771432)) ;
#52419=CARTESIAN_POINT('Origin',(30.5,0.,0.)) ;
#52420=CARTESIAN_POINT('',(2.5,25.2666015370307,-39.8381660191444)) ;
#52421=CARTESIAN_POINT('',(30.5,25.2666015370307,-39.8381660191444)) ;
#52422=CARTESIAN_POINT('',(2.5,26.1171229164955,-39.2858309771432)) ;
#52423=CARTESIAN_POINT('Origin',(2.49999999999999,0.,0.)) ;
#52424=CARTESIAN_POINT('',(30.5,26.1171229164955,-39.2858309771432)) ;
#52425=CARTESIAN_POINT('Origin',(45.,0.,0.)) ;
#52426=CARTESIAN_POINT('',(30.5,33.7143846624785,-32.9972861282626)) ;
#52427=CARTESIAN_POINT('',(2.5,33.7143846624785,-32.9972861282626)) ;
#52428=CARTESIAN_POINT('',(30.5,33.7143846624785,-32.9972861282626)) ;
#52429=CARTESIAN_POINT('',(30.5,32.9972861282625,-33.7143846624786)) ;
#52430=CARTESIAN_POINT('Origin',(30.5,0.,0.)) ;
#52431=CARTESIAN_POINT('',(2.5,32.9972861282626,-33.7143846624785)) ;
#52432=CARTESIAN_POINT('',(30.5,32.9972861282626,-33.7143846624785)) ;
#52433=CARTESIAN_POINT('Origin',(2.49999999999999,0.,0.)) ;
#52434=CARTESIAN_POINT('Origin',(45.,0.,0.)) ;
#52435=CARTESIAN_POINT('',(30.5,29.2924107235055,-36.9788493466936)) ;
#52436=CARTESIAN_POINT('',(30.5,30.0805381247128,-36.3406363610724)) ;
#52437=CARTESIAN_POINT('Origin',(30.5,0.,0.)) ;
#52438=CARTESIAN_POINT('',(2.5,29.2924107235055,-36.9788493466935)) ;
#52439=CARTESIAN_POINT('',(30.5,29.2924107235055,-36.9788493466935)) ;
#52440=CARTESIAN_POINT('',(2.5,30.0805381247128,-36.3406363610724)) ;
#52441=CARTESIAN_POINT('Origin',(2.49999999999999,0.,0.)) ;
#52442=CARTESIAN_POINT('',(30.5,30.0805381247128,-36.3406363610724)) ;
#52443=CARTESIAN_POINT('Origin',(45.,0.,0.)) ;
#52444=CARTESIAN_POINT('',(30.5,36.3406363610723,-30.0805381247129)) ;
#52445=CARTESIAN_POINT('',(30.5,36.9788493466935,-29.2924107235056)) ;
#52446=CARTESIAN_POINT('Origin',(30.5,0.,0.)) ;
#52447=CARTESIAN_POINT('',(2.5,36.3406363610724,-30.0805381247128)) ;
#52448=CARTESIAN_POINT('',(30.5,36.3406363610724,-30.0805381247128)) ;
#52449=CARTESIAN_POINT('',(2.5,36.9788493466935,-29.2924107235056)) ;
#52450=CARTESIAN_POINT('Origin',(2.49999999999999,0.,0.)) ;
#52451=CARTESIAN_POINT('',(30.5,36.9788493466935,-29.2924107235056)) ;
#52452=CARTESIAN_POINT('Origin',(45.,0.,0.)) ;
#52453=CARTESIAN_POINT('',(30.5,39.2858309771432,-26.1171229164956)) ;
#52454=CARTESIAN_POINT('',(30.5,39.8381660191444,-25.2666015370307)) ;
#52455=CARTESIAN_POINT('Origin',(30.5,0.,0.)) ;
#52456=CARTESIAN_POINT('',(2.5,39.2858309771432,-26.1171229164954)) ;
#52457=CARTESIAN_POINT('',(30.5,39.2858309771432,-26.1171229164954)) ;
#52458=CARTESIAN_POINT('',(2.5,39.8381660191444,-25.2666015370307)) ;
#52459=CARTESIAN_POINT('Origin',(2.49999999999999,0.,0.)) ;
#52460=CARTESIAN_POINT('',(30.5,39.8381660191444,-25.2666015370307)) ;
#52461=CARTESIAN_POINT('Origin',(45.,0.,0.)) ;
#52462=CARTESIAN_POINT('',(30.5,41.8006018079397,-21.8675630442458)) ;
#52463=CARTESIAN_POINT('',(30.5,42.2610074080174,-20.9639661767399)) ;
#52464=CARTESIAN_POINT('Origin',(30.5,0.,0.)) ;
#52465=CARTESIAN_POINT('',(2.5,41.8006018079397,-21.8675630442457)) ;
#52466=CARTESIAN_POINT('',(30.5,41.8006018079397,-21.8675630442457)) ;
#52467=CARTESIAN_POINT('',(2.5,42.2610074080174,-20.9639661767399)) ;
#52468=CARTESIAN_POINT('Origin',(2.49999999999999,0.,0.)) ;
#52469=CARTESIAN_POINT('',(30.5,42.2610074080174,-20.9639661767399)) ;
#52470=CARTESIAN_POINT('Origin',(45.,0.,0.)) ;
#52471=CARTESIAN_POINT('',(30.5,43.8573964979902,-17.3784175752015)) ;
#52472=CARTESIAN_POINT('',(30.5,44.2208283560438,-16.4316452160248)) ;
#52473=CARTESIAN_POINT('Origin',(30.5,0.,0.)) ;
#52474=CARTESIAN_POINT('',(2.5,43.8573964979902,-17.3784175752014)) ;
#52475=CARTESIAN_POINT('',(30.5,43.8573964979902,-17.3784175752014)) ;
#52476=CARTESIAN_POINT('',(2.5,44.2208283560438,-16.4316452160248)) ;
#52477=CARTESIAN_POINT('Origin',(2.49999999999999,0.,0.)) ;
#52478=CARTESIAN_POINT('',(30.5,44.2208283560438,-16.4316452160248)) ;
#52479=CARTESIAN_POINT('Origin',(45.,0.,0.)) ;
#52480=CARTESIAN_POINT('',(30.5,45.4336803742585,-12.6988705265356)) ;
#52481=CARTESIAN_POINT('',(30.5,45.6961566547981,-11.7192957117801)) ;
#52482=CARTESIAN_POINT('Origin',(30.5,0.,0.)) ;
#52483=CARTESIAN_POINT('',(2.5,45.4336803742585,-12.6988705265355)) ;
#52484=CARTESIAN_POINT('',(30.5,45.4336803742585,-12.6988705265355)) ;
#52485=CARTESIAN_POINT('',(2.5,45.6961566547981,-11.7192957117801)) ;
#52486=CARTESIAN_POINT('Origin',(2.49999999999999,0.,0.)) ;
#52487=CARTESIAN_POINT('',(30.5,45.6961566547981,-11.7192957117801)) ;
#52488=CARTESIAN_POINT('Origin',(45.,0.,0.)) ;
#52489=CARTESIAN_POINT('',(30.5,46.5121833407376,-7.88019199497153)) ;
#52490=CARTESIAN_POINT('',(30.5,46.670828298707,-6.87854715129677)) ;
#52491=CARTESIAN_POINT('Origin',(30.5,0.,0.)) ;
#52492=CARTESIAN_POINT('',(2.5,46.5121833407376,-7.88019199497139)) ;
#52493=CARTESIAN_POINT('',(30.5,46.5121833407376,-7.88019199497139)) ;
#52494=CARTESIAN_POINT('',(2.5,46.670828298707,-6.87854715129677)) ;
#52495=CARTESIAN_POINT('Origin',(2.49999999999999,0.,0.)) ;
#52496=CARTESIAN_POINT('',(30.5,46.670828298707,-6.87854715129677)) ;
#52497=CARTESIAN_POINT('Origin',(45.,0.,0.)) ;
#52498=CARTESIAN_POINT('',(30.5,47.0810890932354,2.9751764308742)) ;
#52499=CARTESIAN_POINT('',(2.5,47.0810890932354,2.9751764308742)) ;
#52500=CARTESIAN_POINT('',(30.5,47.0810890932354,2.9751764308742)) ;
#52501=CARTESIAN_POINT('',(30.5,47.1341645812764,1.96243578879522)) ;
#52502=CARTESIAN_POINT('Origin',(30.5,0.,0.)) ;
#52503=CARTESIAN_POINT('',(2.5,47.1341645812764,1.96243578879535)) ;
#52504=CARTESIAN_POINT('',(30.5,47.1341645812764,1.96243578879535)) ;
#52505=CARTESIAN_POINT('Origin',(2.49999999999999,0.,0.)) ;
#52506=CARTESIAN_POINT('Origin',(45.,0.,0.)) ;
#52507=CARTESIAN_POINT('',(30.5,47.0810890932354,-2.97517643087433)) ;
#52508=CARTESIAN_POINT('',(30.5,47.1341645812764,-1.96243578879535)) ;
#52509=CARTESIAN_POINT('Origin',(30.5,0.,0.)) ;
#52510=CARTESIAN_POINT('',(2.5,47.0810890932354,-2.9751764308742)) ;
#52511=CARTESIAN_POINT('',(30.5,47.0810890932354,-2.9751764308742)) ;
#52512=CARTESIAN_POINT('',(2.5,47.1341645812764,-1.96243578879535)) ;
#52513=CARTESIAN_POINT('Origin',(2.49999999999999,0.,0.)) ;
#52514=CARTESIAN_POINT('',(30.5,47.1341645812764,-1.96243578879535)) ;
#52515=CARTESIAN_POINT('Origin',(45.,0.,0.)) ;
#52516=CARTESIAN_POINT('',(1.5,-4.89858719658941E-15,40.)) ;
#52517=CARTESIAN_POINT('Origin',(1.5,0.,0.)) ;
#52518=CARTESIAN_POINT('',(45.,-4.89858719658941E-15,40.)) ;
#52519=CARTESIAN_POINT('Origin',(1.5,40.,0.)) ;
#52520=CARTESIAN_POINT('',(1.5,0.,-47.0433475024125)) ;
#52521=CARTESIAN_POINT('Origin',(1.5,0.,0.)) ;
#52522=CARTESIAN_POINT('Origin',(1.5,0.,0.)) ;
#52523=CARTESIAN_POINT('',(0.91109230130857,-6.03030546426507E-15,-49.2411809548974)) ;
#52524=CARTESIAN_POINT('',(1.5,-5.76114849400061E-15,-47.0433475024125)) ;
#52525=CARTESIAN_POINT('',(0.911092301308557,-6.03030546426507E-15,49.2411809548974)) ;
#52526=CARTESIAN_POINT('Origin',(0.911092301308557,0.,0.)) ;
#52527=CARTESIAN_POINT('Origin',(0.911092301308557,0.,0.)) ;
#52528=CARTESIAN_POINT('Origin',(0.911092301308557,0.,0.)) ;
#52529=CARTESIAN_POINT('',(1.87701812759763,0.,-49.5)) ;
#52530=CARTESIAN_POINT('',(1.87701812759764,-6.06200165577939E-15,49.5)) ;
#52531=CARTESIAN_POINT('Origin',(1.87701812759763,0.,0.)) ;
#52532=CARTESIAN_POINT('Origin',(1.87701812759763,0.,0.)) ;
#52533=CARTESIAN_POINT('',(0.911092301308557,-6.03030546426507E-15,49.2411809548974)) ;
#52534=CARTESIAN_POINT('Origin',(1.87701812759763,0.,0.)) ;
#52535=CARTESIAN_POINT('',(2.49999999999999,-5.77727127497764E-15,-47.175)) ;
#52536=CARTESIAN_POINT('',(1.87701812759763,-6.0620016557794E-15,-49.5)) ;
#52537=CARTESIAN_POINT('Origin',(2.49999999999999,0.,0.)) ;
#52538=CARTESIAN_POINT('Origin',(2.49999999999999,0.,0.)) ;
#52539=CARTESIAN_POINT('Origin',(2.49999999999999,0.,0.)) ;
#52540=CARTESIAN_POINT('Origin',(2.49999999999999,0.,0.)) ;
#52541=CARTESIAN_POINT('Origin',(2.49999999999999,0.,0.)) ;
#52542=CARTESIAN_POINT('Origin',(2.49999999999999,0.,0.)) ;
#52543=CARTESIAN_POINT('Origin',(2.49999999999999,0.,0.)) ;
#52544=CARTESIAN_POINT('Origin',(2.49999999999999,0.,0.)) ;
#52545=CARTESIAN_POINT('Origin',(2.49999999999999,0.,0.)) ;
#52546=CARTESIAN_POINT('Origin',(2.49999999999999,0.,0.)) ;
#52547=CARTESIAN_POINT('Origin',(2.49999999999999,0.,0.)) ;
#52548=CARTESIAN_POINT('Origin',(2.49999999999999,0.,0.)) ;
#52549=CARTESIAN_POINT('Origin',(2.49999999999999,0.,0.)) ;
#52550=CARTESIAN_POINT('Origin',(2.49999999999999,0.,0.)) ;
#52551=CARTESIAN_POINT('Origin',(2.49999999999999,0.,0.)) ;
#52552=CARTESIAN_POINT('Origin',(2.49999999999999,0.,0.)) ;
#52553=CARTESIAN_POINT('Origin',(2.49999999999999,0.,0.)) ;
#52554=CARTESIAN_POINT('Origin',(2.49999999999999,0.,0.)) ;
#52555=CARTESIAN_POINT('Origin',(2.49999999999999,0.,0.)) ;
#52556=CARTESIAN_POINT('Origin',(2.49999999999999,0.,0.)) ;
#52557=CARTESIAN_POINT('Origin',(2.49999999999999,0.,0.)) ;
#52558=CARTESIAN_POINT('Origin',(2.49999999999999,0.,0.)) ;
#52559=CARTESIAN_POINT('Origin',(2.49999999999999,0.,0.)) ;
#52560=CARTESIAN_POINT('Origin',(2.49999999999999,0.,0.)) ;
#52561=CARTESIAN_POINT('Origin',(2.49999999999999,0.,0.)) ;
#52562=CARTESIAN_POINT('Origin',(2.49999999999999,0.,0.)) ;
#52563=CARTESIAN_POINT('Origin',(2.49999999999999,0.,0.)) ;
#52564=CARTESIAN_POINT('Origin',(2.49999999999999,0.,0.)) ;
#52565=CARTESIAN_POINT('Origin',(2.49999999999999,0.,0.)) ;
#52566=CARTESIAN_POINT('Origin',(2.49999999999999,0.,0.)) ;
#52567=CARTESIAN_POINT('Origin',(2.49999999999999,0.,0.)) ;
#52568=CARTESIAN_POINT('Origin',(2.49999999999999,0.,0.)) ;
#52569=CARTESIAN_POINT('Origin',(2.49999999999999,0.,0.)) ;
#52570=CARTESIAN_POINT('Origin',(2.49999999999999,0.,0.)) ;
#52571=CARTESIAN_POINT('Origin',(2.49999999999999,0.,0.)) ;
#52572=CARTESIAN_POINT('Origin',(2.49999999999999,0.,0.)) ;
#52573=CARTESIAN_POINT('Origin',(2.49999999999999,0.,0.)) ;
#52574=CARTESIAN_POINT('Origin',(2.49999999999999,0.,0.)) ;
#52575=CARTESIAN_POINT('Origin',(2.49999999999999,0.,0.)) ;
#52576=CARTESIAN_POINT('Origin',(2.49999999999999,0.,0.)) ;
#52577=CARTESIAN_POINT('Origin',(2.49999999999999,0.,0.)) ;
#52578=CARTESIAN_POINT('Origin',(2.49999999999999,0.,0.)) ;
#52579=CARTESIAN_POINT('Origin',(2.49999999999999,0.,0.)) ;
#52580=CARTESIAN_POINT('Origin',(2.49999999999999,0.,0.)) ;
#52581=CARTESIAN_POINT('Origin',(2.49999999999999,0.,0.)) ;
#52582=CARTESIAN_POINT('Origin',(2.49999999999999,0.,0.)) ;
#52583=CARTESIAN_POINT('Origin',(2.49999999999999,0.,0.)) ;
#52584=CARTESIAN_POINT('Origin',(2.49999999999999,0.,0.)) ;
#52585=CARTESIAN_POINT('Origin',(2.49999999999999,0.,0.)) ;
#52586=CARTESIAN_POINT('Origin',(2.49999999999999,0.,0.)) ;
#52587=CARTESIAN_POINT('Origin',(2.49999999999999,0.,0.)) ;
#52588=CARTESIAN_POINT('Origin',(2.49999999999999,0.,0.)) ;
#52589=CARTESIAN_POINT('Origin',(2.49999999999999,0.,0.)) ;
#52590=CARTESIAN_POINT('Origin',(2.49999999999999,0.,0.)) ;
#52591=CARTESIAN_POINT('Origin',(2.49999999999999,0.,0.)) ;
#52592=CARTESIAN_POINT('Origin',(2.49999999999999,0.,0.)) ;
#52593=CARTESIAN_POINT('Origin',(2.49999999999999,0.,0.)) ;
#52594=CARTESIAN_POINT('Origin',(2.49999999999999,0.,0.)) ;
#52595=CARTESIAN_POINT('Origin',(2.49999999999999,0.,0.)) ;
#52596=CARTESIAN_POINT('Origin',(2.49999999999999,0.,0.)) ;
#52597=CARTESIAN_POINT('Origin',(2.49999999999999,0.,0.)) ;
#52598=CARTESIAN_POINT('Origin',(30.5,0.,0.)) ;
#52599=CARTESIAN_POINT('',(31.1229818724024,0.,-49.5)) ;
#52600=CARTESIAN_POINT('',(31.1229818724024,-6.0620016557794E-15,49.5)) ;
#52601=CARTESIAN_POINT('Origin',(31.1229818724024,0.,0.)) ;
#52602=CARTESIAN_POINT('Origin',(31.1229818724024,0.,0.)) ;
#52603=CARTESIAN_POINT('',(30.5,-5.77727127497764E-15,47.175)) ;
#52604=CARTESIAN_POINT('',(30.5,-5.77727127497764E-15,47.175)) ;
#52605=CARTESIAN_POINT('Origin',(30.5,0.,0.)) ;
#52606=CARTESIAN_POINT('Origin',(30.5,0.,0.)) ;
#52607=CARTESIAN_POINT('Origin',(30.5,0.,0.)) ;
#52608=CARTESIAN_POINT('Origin',(30.5,0.,0.)) ;
#52609=CARTESIAN_POINT('Origin',(30.5,0.,0.)) ;
#52610=CARTESIAN_POINT('Origin',(30.5,0.,0.)) ;
#52611=CARTESIAN_POINT('Origin',(30.5,0.,0.)) ;
#52612=CARTESIAN_POINT('Origin',(30.5,0.,0.)) ;
#52613=CARTESIAN_POINT('Origin',(30.5,0.,0.)) ;
#52614=CARTESIAN_POINT('Origin',(30.5,0.,0.)) ;
#52615=CARTESIAN_POINT('Origin',(30.5,0.,0.)) ;
#52616=CARTESIAN_POINT('Origin',(30.5,0.,0.)) ;
#52617=CARTESIAN_POINT('Origin',(30.5,0.,0.)) ;
#52618=CARTESIAN_POINT('Origin',(30.5,0.,0.)) ;
#52619=CARTESIAN_POINT('Origin',(30.5,0.,0.)) ;
#52620=CARTESIAN_POINT('Origin',(30.5,0.,0.)) ;
#52621=CARTESIAN_POINT('Origin',(30.5,0.,0.)) ;
#52622=CARTESIAN_POINT('Origin',(30.5,0.,0.)) ;
#52623=CARTESIAN_POINT('Origin',(30.5,0.,0.)) ;
#52624=CARTESIAN_POINT('Origin',(30.5,0.,0.)) ;
#52625=CARTESIAN_POINT('Origin',(30.5,0.,0.)) ;
#52626=CARTESIAN_POINT('Origin',(30.5,0.,0.)) ;
#52627=CARTESIAN_POINT('Origin',(30.5,0.,0.)) ;
#52628=CARTESIAN_POINT('Origin',(30.5,0.,0.)) ;
#52629=CARTESIAN_POINT('Origin',(30.5,0.,0.)) ;
#52630=CARTESIAN_POINT('Origin',(30.5,0.,0.)) ;
#52631=CARTESIAN_POINT('Origin',(30.5,0.,0.)) ;
#52632=CARTESIAN_POINT('Origin',(30.5,0.,0.)) ;
#52633=CARTESIAN_POINT('Origin',(30.5,0.,0.)) ;
#52634=CARTESIAN_POINT('Origin',(30.5,0.,0.)) ;
#52635=CARTESIAN_POINT('Origin',(30.5,0.,0.)) ;
#52636=CARTESIAN_POINT('Origin',(30.5,0.,0.)) ;
#52637=CARTESIAN_POINT('Origin',(30.5,0.,0.)) ;
#52638=CARTESIAN_POINT('Origin',(30.5,0.,0.)) ;
#52639=CARTESIAN_POINT('Origin',(30.5,0.,0.)) ;
#52640=CARTESIAN_POINT('Origin',(30.5,0.,0.)) ;
#52641=CARTESIAN_POINT('Origin',(30.5,0.,0.)) ;
#52642=CARTESIAN_POINT('Origin',(30.5,0.,0.)) ;
#52643=CARTESIAN_POINT('Origin',(30.5,0.,0.)) ;
#52644=CARTESIAN_POINT('Origin',(30.5,0.,0.)) ;
#52645=CARTESIAN_POINT('Origin',(30.5,0.,0.)) ;
#52646=CARTESIAN_POINT('Origin',(30.5,0.,0.)) ;
#52647=CARTESIAN_POINT('Origin',(30.5,0.,0.)) ;
#52648=CARTESIAN_POINT('Origin',(30.5,0.,0.)) ;
#52649=CARTESIAN_POINT('Origin',(30.5,0.,0.)) ;
#52650=CARTESIAN_POINT('Origin',(30.5,0.,0.)) ;
#52651=CARTESIAN_POINT('Origin',(30.5,0.,0.)) ;
#52652=CARTESIAN_POINT('Origin',(30.5,0.,0.)) ;
#52653=CARTESIAN_POINT('Origin',(30.5,0.,0.)) ;
#52654=CARTESIAN_POINT('Origin',(30.5,0.,0.)) ;
#52655=CARTESIAN_POINT('Origin',(30.5,0.,0.)) ;
#52656=CARTESIAN_POINT('Origin',(30.5,0.,0.)) ;
#52657=CARTESIAN_POINT('Origin',(30.5,0.,0.)) ;
#52658=CARTESIAN_POINT('Origin',(30.5,0.,0.)) ;
#52659=CARTESIAN_POINT('Origin',(30.5,0.,0.)) ;
#52660=CARTESIAN_POINT('Origin',(30.5,0.,0.)) ;
#52661=CARTESIAN_POINT('Origin',(30.5,0.,0.)) ;
#52662=CARTESIAN_POINT('Origin',(30.5,0.,0.)) ;
#52663=CARTESIAN_POINT('Origin',(30.5,0.,0.)) ;
#52664=CARTESIAN_POINT('Origin',(30.5,0.,0.)) ;
#52665=CARTESIAN_POINT('Origin',(30.5,0.,0.)) ;
#52666=CARTESIAN_POINT('Origin',(31.1229818724024,0.,0.)) ;
#52667=CARTESIAN_POINT('',(32.0889076986914,-6.03030546426508E-15,-49.2411809548975)) ;
#52668=CARTESIAN_POINT('',(31.1229818724024,-6.0620016557794E-15,-49.5)) ;
#52669=CARTESIAN_POINT('',(32.0889076986914,-6.03030546426508E-15,49.2411809548975)) ;
#52670=CARTESIAN_POINT('Origin',(32.0889076986914,0.,0.)) ;
#52671=CARTESIAN_POINT('Origin',(32.0889076986914,0.,0.)) ;
#52672=CARTESIAN_POINT('Origin',(32.0889076986914,0.,0.)) ;
#52673=CARTESIAN_POINT('',(31.5,-5.76114849400062E-15,47.0433475024126)) ;
#52674=CARTESIAN_POINT('Origin',(31.5,0.,0.)) ;
#52675=CARTESIAN_POINT('',(32.0889076986914,-6.03030546426508E-15,49.2411809548975)) ;
#52676=CARTESIAN_POINT('Origin',(31.5,47.0433475024126,0.)) ;
#52677=CARTESIAN_POINT('',(31.5,-4.89858719658941E-15,40.)) ;
#52678=CARTESIAN_POINT('Origin',(31.5,0.,0.)) ;
#52679=CARTESIAN_POINT('Origin',(45.,0.,0.)) ;
#52680=CARTESIAN_POINT('',(33.,-4.89858719658941E-15,40.)) ;
#52681=CARTESIAN_POINT('Origin',(33.,0.,0.)) ;
#52682=CARTESIAN_POINT('',(45.,-4.89858719658941E-15,40.)) ;
#52683=CARTESIAN_POINT('Origin',(33.,40.,0.)) ;
#52684=CARTESIAN_POINT('',(33.,-4.59242549680258E-15,37.5)) ;
#52685=CARTESIAN_POINT('Origin',(33.,0.,0.)) ;
#52686=CARTESIAN_POINT('Origin',(45.,0.,0.)) ;
#52687=CARTESIAN_POINT('',(45.,-4.59242549680258E-15,37.5)) ;
#52688=CARTESIAN_POINT('Origin',(45.,0.,0.)) ;
#52689=CARTESIAN_POINT('',(45.,-4.59242549680258E-15,37.5)) ;
#52690=CARTESIAN_POINT('Origin',(45.,37.5,0.)) ;
#52691=CARTESIAN_POINT('Origin',(45.,0.,0.)) ;
#52692=CARTESIAN_POINT('Origin',(2.5,-2.84494650060196E-12,-7.9580439460436E-14)) ;
#52693=CARTESIAN_POINT('',(2.5,46.5975179480543,-1.39998000660682)) ;
#52694=CARTESIAN_POINT('Origin',(2.5,46.5946320137324,-1.93997229486941)) ;
#52695=CARTESIAN_POINT('',(2.5,46.5975179480543,1.39998000660682)) ;
#52696=CARTESIAN_POINT('Origin',(2.5,46.5946320137324,1.93997229486942)) ;
#52697=CARTESIAN_POINT('Origin',(2.5,46.6049999999905,0.)) ;
#52698=CARTESIAN_POINT('Origin',(30.5,-2.84494650060196E-12,-7.9580439460436E-14)) ;
#52699=CARTESIAN_POINT('',(30.5,46.5975179480543,-1.39998000660682)) ;
#52700=CARTESIAN_POINT('Origin',(30.5,46.5946320137324,-1.93997229486941)) ;
#52701=CARTESIAN_POINT('',(30.5,46.5975179480543,1.39998000660682)) ;
#52702=CARTESIAN_POINT('Origin',(30.5,46.6049999999905,0.)) ;
#52703=CARTESIAN_POINT('Origin',(30.5,46.5946320137324,1.93997229486942)) ;
#52704=CARTESIAN_POINT('Origin',(30.5,46.5946320137324,1.93997229486942)) ;
#52705=CARTESIAN_POINT('',(30.5,46.5975179480543,1.39998000660682)) ;
#52706=CARTESIAN_POINT('Origin',(30.5,46.6049999999905,0.)) ;
#52707=CARTESIAN_POINT('',(30.5,46.5975179480543,-1.39998000660682)) ;
#52708=CARTESIAN_POINT('Origin',(30.5,46.5946320137324,-1.93997229486941)) ;
#52709=CARTESIAN_POINT('Origin',(2.5,-2.82104316495704E-12,-3.76522375273045E-13)) ;
#52710=CARTESIAN_POINT('',(2.5,46.19591411046,6.26307771284532)) ;
#52711=CARTESIAN_POINT('Origin',(2.5,46.1365994215198,6.79981020457273)) ;
#52712=CARTESIAN_POINT('',(2.5,46.4885896278522,3.47845617354872)) ;
#52713=CARTESIAN_POINT('Origin',(2.5,46.3496929336289,4.871549030588)) ;
#52714=CARTESIAN_POINT('Origin',(2.5,46.5421640670489,2.94112035726179)) ;
#52715=CARTESIAN_POINT('Origin',(30.5,-2.82104316495704E-12,-3.76522375273045E-13)) ;
#52716=CARTESIAN_POINT('',(30.5,46.4885896278522,3.47845617354872)) ;
#52717=CARTESIAN_POINT('Origin',(30.5,46.5421640670489,2.94112035726179)) ;
#52718=CARTESIAN_POINT('',(30.5,46.19591411046,6.26307771284532)) ;
#52719=CARTESIAN_POINT('Origin',(30.5,46.3496929336289,4.871549030588)) ;
#52720=CARTESIAN_POINT('Origin',(30.5,46.1365994215198,6.79981020457273)) ;
#52721=CARTESIAN_POINT('Origin',(30.5,46.1365994215198,6.79981020457273)) ;
#52722=CARTESIAN_POINT('',(30.5,46.19591411046,6.26307771284532)) ;
#52723=CARTESIAN_POINT('Origin',(30.5,46.3496929336289,4.871549030588)) ;
#52724=CARTESIAN_POINT('',(30.5,46.4885896278522,3.47845617354872)) ;
#52725=CARTESIAN_POINT('Origin',(30.5,46.5421640670489,2.94112035726179)) ;
#52726=CARTESIAN_POINT('Origin',(2.5,-2.83768000704297E-12,2.18233396300179E-13)) ;
#52727=CARTESIAN_POINT('',(2.5,46.4885896278521,-3.47845617354871)) ;
#52728=CARTESIAN_POINT('Origin',(2.5,46.5421640670489,-2.94112035726178)) ;
#52729=CARTESIAN_POINT('',(2.5,46.1959141104601,-6.26307771284532)) ;
#52730=CARTESIAN_POINT('Origin',(2.5,46.3496929336289,-4.871549030588)) ;
#52731=CARTESIAN_POINT('Origin',(2.5,46.1365994215199,-6.79981020457273)) ;
#52732=CARTESIAN_POINT('Origin',(30.5,-2.83768000704297E-12,2.18233396300179E-13)) ;
#52733=CARTESIAN_POINT('',(30.5,46.1959141104601,-6.26307771284532)) ;
#52734=CARTESIAN_POINT('Origin',(30.5,46.1365994215199,-6.79981020457273)) ;
#52735=CARTESIAN_POINT('',(30.5,46.4885896278521,-3.47845617354871)) ;
#52736=CARTESIAN_POINT('Origin',(30.5,46.3496929336289,-4.871549030588)) ;
#52737=CARTESIAN_POINT('Origin',(30.5,46.5421640670489,-2.94112035726178)) ;
#52738=CARTESIAN_POINT('Origin',(30.5,46.5421640670489,-2.94112035726178)) ;
#52739=CARTESIAN_POINT('',(30.5,46.4885896278521,-3.47845617354871)) ;
#52740=CARTESIAN_POINT('Origin',(30.5,46.3496929336289,-4.871549030588)) ;
#52741=CARTESIAN_POINT('',(30.5,46.1959141104601,-6.26307771284532)) ;
#52742=CARTESIAN_POINT('Origin',(30.5,46.1365994215199,-6.79981020457273)) ;
#52743=CARTESIAN_POINT('Origin',(2.5,-2.79932329750409E-12,5.13656221302654E-13)) ;
#52744=CARTESIAN_POINT('',(2.5,45.8703225913244,-8.3187816599531)) ;
#52745=CARTESIAN_POINT('Origin',(2.5,45.9797704312728,-7.78998947928981)) ;
#52746=CARTESIAN_POINT('',(2.5,45.2881781707551,-11.0575558290286)) ;
#52747=CARTESIAN_POINT('Origin',(2.5,45.5865689321897,-9.6897243505597)) ;
#52748=CARTESIAN_POINT('Origin',(2.5,45.1730845913411,-11.585147970723)) ;
#52749=CARTESIAN_POINT('Origin',(30.5,-2.79932329750409E-12,5.13656221302654E-13)) ;
#52750=CARTESIAN_POINT('',(30.5,45.2881781707551,-11.0575558290286)) ;
#52751=CARTESIAN_POINT('Origin',(30.5,45.1730845913411,-11.585147970723)) ;
#52752=CARTESIAN_POINT('',(30.5,45.8703225913244,-8.3187816599531)) ;
#52753=CARTESIAN_POINT('Origin',(30.5,45.5865689321897,-9.6897243505597)) ;
#52754=CARTESIAN_POINT('Origin',(30.5,45.9797704312728,-7.78998947928981)) ;
#52755=CARTESIAN_POINT('Origin',(30.5,45.9797704312728,-7.78998947928981)) ;
#52756=CARTESIAN_POINT('',(30.5,45.8703225913244,-8.3187816599531)) ;
#52757=CARTESIAN_POINT('Origin',(30.5,45.5865689321897,-9.6897243505597)) ;
#52758=CARTESIAN_POINT('',(30.5,45.2881781707551,-11.0575558290286)) ;
#52759=CARTESIAN_POINT('Origin',(30.5,45.1730845913411,-11.585147970723)) ;
#52760=CARTESIAN_POINT('Origin',(2.5,-2.73029661612169E-12,8.03451321255064E-13)) ;
#52761=CARTESIAN_POINT('',(2.5,44.7494907015041,-13.0679648336741)) ;
#52762=CARTESIAN_POINT('Origin',(2.5,44.9136128087662,-12.5535098464227)) ;
#52763=CARTESIAN_POINT('',(2.5,43.8842554738508,-15.7308850496068)) ;
#52764=CARTESIAN_POINT('Origin',(2.5,44.3239889419266,-14.4017370228415)) ;
#52765=CARTESIAN_POINT('Origin',(2.5,43.7146439933038,-16.2435564313579)) ;
#52766=CARTESIAN_POINT('Origin',(30.5,-2.73029661612169E-12,8.03451321255064E-13)) ;
#52767=CARTESIAN_POINT('',(30.5,43.8842554738508,-15.7308850496068)) ;
#52768=CARTESIAN_POINT('Origin',(30.5,43.7146439933038,-16.2435564313579)) ;
#52769=CARTESIAN_POINT('',(30.5,44.7494907015041,-13.0679648336741)) ;
#52770=CARTESIAN_POINT('Origin',(30.5,44.3239889419266,-14.4017370228415)) ;
#52771=CARTESIAN_POINT('Origin',(30.5,44.9136128087662,-12.5535098464227)) ;
#52772=CARTESIAN_POINT('Origin',(30.5,44.9136128087662,-12.5535098464227)) ;
#52773=CARTESIAN_POINT('',(30.5,44.7494907015041,-13.0679648336741)) ;
#52774=CARTESIAN_POINT('Origin',(30.5,44.3239889419266,-14.4017370228415)) ;
#52775=CARTESIAN_POINT('',(30.5,43.8842554738508,-15.7308850496068)) ;
#52776=CARTESIAN_POINT('Origin',(30.5,43.7146439933038,-16.2435564313579)) ;
#52777=CARTESIAN_POINT('Origin',(2.5,-2.63135623366177E-12,1.0844436403988E-12)) ;
#52778=CARTESIAN_POINT('',(2.5,43.1383740271251,-17.6739726500298)) ;
#52779=CARTESIAN_POINT('Origin',(2.5,43.355372245549,-17.1794913326873)) ;
#52780=CARTESIAN_POINT('',(2.5,41.9995276906041,-20.2318634016821)) ;
#52781=CARTESIAN_POINT('Origin',(2.5,42.5757860534247,-18.9559612505438)) ;
#52782=CARTESIAN_POINT('Origin',(2.5,41.7772566077985,-20.7239970885482)) ;
#52783=CARTESIAN_POINT('Origin',(30.5,-2.63135623366177E-12,1.0844436403988E-12)) ;
#52784=CARTESIAN_POINT('',(30.5,41.9995276906041,-20.2318634016821)) ;
#52785=CARTESIAN_POINT('Origin',(30.5,41.7772566077985,-20.7239970885482)) ;
#52786=CARTESIAN_POINT('',(30.5,43.1383740271251,-17.6739726500298)) ;
#52787=CARTESIAN_POINT('Origin',(30.5,42.5757860534247,-18.9559612505438)) ;
#52788=CARTESIAN_POINT('Origin',(30.5,43.355372245549,-17.1794913326873)) ;
#52789=CARTESIAN_POINT('Origin',(30.5,43.355372245549,-17.1794913326873)) ;
#52790=CARTESIAN_POINT('',(30.5,43.1383740271251,-17.6739726500298)) ;
#52791=CARTESIAN_POINT('Origin',(30.5,42.5757860534247,-18.9559612505438)) ;
#52792=CARTESIAN_POINT('',(30.5,41.9995276906041,-20.2318634016821)) ;
#52793=CARTESIAN_POINT('Origin',(30.5,41.7772566077985,-20.7239970885482)) ;
#52794=CARTESIAN_POINT('Origin',(2.5,-2.50358616165916E-12,1.35355456808391E-12)) ;
#52795=CARTESIAN_POINT('',(2.5,41.0546242996198,-22.0863407235153)) ;
#52796=CARTESIAN_POINT('Origin',(2.5,41.3221211513146,-21.6172507168713)) ;
#52797=CARTESIAN_POINT('',(2.5,39.654644293013,-24.511177224539)) ;
#52798=CARTESIAN_POINT('Origin',(2.5,40.3611139433656,-23.3024999999953)) ;
#52799=CARTESIAN_POINT('Origin',(2.5,39.3821488564453,-24.9773812968611)) ;
#52800=CARTESIAN_POINT('Origin',(30.5,-2.50358616165916E-12,1.35355456808391E-12)) ;
#52801=CARTESIAN_POINT('',(30.5,39.654644293013,-24.511177224539)) ;
#52802=CARTESIAN_POINT('Origin',(30.5,39.3821488564453,-24.9773812968611)) ;
#52803=CARTESIAN_POINT('',(30.5,41.0546242996198,-22.0863407235153)) ;
#52804=CARTESIAN_POINT('Origin',(30.5,40.3611139433656,-23.3024999999953)) ;
#52805=CARTESIAN_POINT('Origin',(30.5,41.3221211513146,-21.6172507168713)) ;
#52806=CARTESIAN_POINT('Origin',(30.5,41.3221211513146,-21.6172507168713)) ;
#52807=CARTESIAN_POINT('',(30.5,41.0546242996198,-22.0863407235153)) ;
#52808=CARTESIAN_POINT('Origin',(30.5,40.3611139433656,-23.3024999999953)) ;
#52809=CARTESIAN_POINT('',(30.5,39.654644293013,-24.511177224539)) ;
#52810=CARTESIAN_POINT('Origin',(30.5,39.3821488564453,-24.9773812968611)) ;
#52811=CARTESIAN_POINT('Origin',(2.5,-2.34838627576032E-12,1.60783566867159E-12)) ;
#52812=CARTESIAN_POINT('',(2.5,38.5210715170554,-26.2567262261701)) ;
#52813=CARTESIAN_POINT('Origin',(2.5,38.8361362505367,-25.8181669785007)) ;
#52814=CARTESIAN_POINT('',(2.5,36.8752963142798,-28.5219414604302)) ;
#52815=CARTESIAN_POINT('Origin',(2.5,37.7042370228368,-27.3937316830851)) ;
#52816=CARTESIAN_POINT('Origin',(2.5,36.5555620409763,-28.9571080888326)) ;
#52817=CARTESIAN_POINT('Origin',(30.5,-2.34838627576032E-12,1.60783566867159E-12)) ;
#52818=CARTESIAN_POINT('',(30.5,36.8752963142798,-28.5219414604302)) ;
#52819=CARTESIAN_POINT('Origin',(30.5,36.5555620409763,-28.9571080888326)) ;
#52820=CARTESIAN_POINT('',(30.5,38.5210715170554,-26.2567262261701)) ;
#52821=CARTESIAN_POINT('Origin',(30.5,37.7042370228368,-27.3937316830851)) ;
#52822=CARTESIAN_POINT('Origin',(30.5,38.8361362505367,-25.8181669785007)) ;
#52823=CARTESIAN_POINT('Origin',(30.5,38.8361362505367,-25.8181669785007)) ;
#52824=CARTESIAN_POINT('',(30.5,38.5210715170554,-26.2567262261701)) ;
#52825=CARTESIAN_POINT('Origin',(30.5,37.7042370228368,-27.3937316830851)) ;
#52826=CARTESIAN_POINT('',(30.5,36.8752963142798,-28.5219414604302)) ;
#52827=CARTESIAN_POINT('Origin',(30.5,36.5555620409763,-28.9571080888326)) ;
#52828=CARTESIAN_POINT('Origin',(2.5,-1.96278056880054E-12,2.0609575629719E-12)) ;
#52829=CARTESIAN_POINT('',(2.5,32.220213337081,-33.6919348724754)) ;
#52830=CARTESIAN_POINT('Origin',(2.5,32.6195747449183,-33.3284648380432)) ;
#52831=CARTESIAN_POINT('',(2.5,30.1394375417177,-35.5654738138977)) ;
#52832=CARTESIAN_POINT('Origin',(2.5,31.1848319093482,-34.6342645913669)) ;
#52833=CARTESIAN_POINT('Origin',(2.5,29.736213999915,-35.924654514014)) ;
#52834=CARTESIAN_POINT('Origin',(30.5,-1.96278056880054E-12,2.0609575629719E-12)) ;
#52835=CARTESIAN_POINT('',(30.5,30.1394375417177,-35.5654738138977)) ;
#52836=CARTESIAN_POINT('Origin',(30.5,29.736213999915,-35.924654514014)) ;
#52837=CARTESIAN_POINT('',(30.5,32.220213337081,-33.6919348724754)) ;
#52838=CARTESIAN_POINT('Origin',(30.5,31.1848319093482,-34.6342645913669)) ;
#52839=CARTESIAN_POINT('Origin',(30.5,32.6195747449183,-33.3284648380432)) ;
#52840=CARTESIAN_POINT('Origin',(30.5,32.6195747449183,-33.3284648380432)) ;
#52841=CARTESIAN_POINT('',(30.5,32.220213337081,-33.6919348724754)) ;
#52842=CARTESIAN_POINT('Origin',(30.5,31.1848319093482,-34.6342645913669)) ;
#52843=CARTESIAN_POINT('',(30.5,30.1394375417177,-35.5654738138977)) ;
#52844=CARTESIAN_POINT('Origin',(30.5,29.736213999915,-35.924654514014)) ;
#52845=CARTESIAN_POINT('Origin',(2.5,-2.16745697839284E-12,1.84450098521206E-12)) ;
#52846=CARTESIAN_POINT('',(2.5,35.5654738138977,-30.1394375417177)) ;
#52847=CARTESIAN_POINT('Origin',(2.5,35.9246545140139,-29.7362139999149)) ;
#52848=CARTESIAN_POINT('',(2.5,33.6919348724755,-32.220213337081)) ;
#52849=CARTESIAN_POINT('Origin',(2.5,34.6342645913669,-31.1848319093482)) ;
#52850=CARTESIAN_POINT('Origin',(2.5,33.3284648380432,-32.6195747449184)) ;
#52851=CARTESIAN_POINT('Origin',(30.5,-2.16745697839284E-12,1.84450098521206E-12)) ;
#52852=CARTESIAN_POINT('',(30.5,33.6919348724755,-32.220213337081)) ;
#52853=CARTESIAN_POINT('Origin',(30.5,33.3284648380432,-32.6195747449184)) ;
#52854=CARTESIAN_POINT('',(30.5,35.5654738138977,-30.1394375417177)) ;
#52855=CARTESIAN_POINT('Origin',(30.5,34.6342645913669,-31.1848319093482)) ;
#52856=CARTESIAN_POINT('Origin',(30.5,35.9246545140139,-29.7362139999149)) ;
#52857=CARTESIAN_POINT('Origin',(30.5,35.9246545140139,-29.7362139999149)) ;
#52858=CARTESIAN_POINT('',(30.5,35.5654738138977,-30.1394375417177)) ;
#52859=CARTESIAN_POINT('Origin',(30.5,34.6342645913669,-31.1848319093482)) ;
#52860=CARTESIAN_POINT('',(30.5,33.6919348724755,-32.220213337081)) ;
#52861=CARTESIAN_POINT('Origin',(30.5,33.3284648380432,-32.6195747449184)) ;
#52862=CARTESIAN_POINT('Origin',(2.5,-1.73659952455823E-12,2.25483385838873E-12)) ;
#52863=CARTESIAN_POINT('',(2.5,28.5219414604302,-36.8752963142797)) ;
#52864=CARTESIAN_POINT('Origin',(2.5,28.9571080888326,-36.5555620409762)) ;
#52865=CARTESIAN_POINT('',(2.5,26.2567262261701,-38.5210715170554)) ;
#52866=CARTESIAN_POINT('Origin',(2.5,27.3937316830851,-37.7042370228368)) ;
#52867=CARTESIAN_POINT('Origin',(2.5,25.8181669785007,-38.8361362505368)) ;
#52868=CARTESIAN_POINT('Origin',(30.5,-1.73659952455823E-12,2.25483385838873E-12)) ;
#52869=CARTESIAN_POINT('',(30.5,26.2567262261701,-38.5210715170554)) ;
#52870=CARTESIAN_POINT('Origin',(30.5,25.8181669785007,-38.8361362505368)) ;
#52871=CARTESIAN_POINT('',(30.5,28.5219414604302,-36.8752963142797)) ;
#52872=CARTESIAN_POINT('Origin',(30.5,27.3937316830851,-37.7042370228368)) ;
#52873=CARTESIAN_POINT('Origin',(30.5,28.9571080888326,-36.5555620409762)) ;
#52874=CARTESIAN_POINT('Origin',(30.5,28.9571080888326,-36.5555620409762)) ;
#52875=CARTESIAN_POINT('',(30.5,28.5219414604302,-36.8752963142797)) ;
#52876=CARTESIAN_POINT('Origin',(30.5,27.3937316830851,-37.7042370228368)) ;
#52877=CARTESIAN_POINT('',(30.5,26.2567262261701,-38.5210715170554)) ;
#52878=CARTESIAN_POINT('Origin',(30.5,25.8181669785007,-38.8361362505368)) ;
#52879=CARTESIAN_POINT('Origin',(2.5,-1.49139193251805E-12,2.42400572219872E-12)) ;
#52880=CARTESIAN_POINT('',(2.5,24.511177224539,-39.6546442930129)) ;
#52881=CARTESIAN_POINT('Origin',(2.5,24.9773812968611,-39.3821488564452)) ;
#52882=CARTESIAN_POINT('',(2.5,22.0863407235154,-41.0546242996198)) ;
#52883=CARTESIAN_POINT('Origin',(2.5,23.3024999999953,-40.3611139433656)) ;
#52884=CARTESIAN_POINT('Origin',(2.5,21.6172507168713,-41.3221211513147)) ;
#52885=CARTESIAN_POINT('Origin',(30.5,-1.49139193251805E-12,2.42400572219872E-12)) ;
#52886=CARTESIAN_POINT('',(30.5,22.0863407235154,-41.0546242996198)) ;
#52887=CARTESIAN_POINT('Origin',(30.5,21.6172507168713,-41.3221211513147)) ;
#52888=CARTESIAN_POINT('',(30.5,24.511177224539,-39.6546442930129)) ;
#52889=CARTESIAN_POINT('Origin',(30.5,23.3024999999953,-40.3611139433656)) ;
#52890=CARTESIAN_POINT('Origin',(30.5,24.9773812968611,-39.3821488564452)) ;
#52891=CARTESIAN_POINT('Origin',(30.5,24.9773812968611,-39.3821488564452)) ;
#52892=CARTESIAN_POINT('',(30.5,24.511177224539,-39.6546442930129)) ;
#52893=CARTESIAN_POINT('Origin',(30.5,23.3024999999953,-40.3611139433656)) ;
#52894=CARTESIAN_POINT('',(30.5,22.0863407235154,-41.0546242996198)) ;
#52895=CARTESIAN_POINT('Origin',(30.5,21.6172507168713,-41.3221211513147)) ;
#52896=CARTESIAN_POINT('Origin',(2.5,-1.22984433837137E-12,2.5666196720605E-12)) ;
#52897=CARTESIAN_POINT('',(2.5,20.2318634016821,-41.9995276906041)) ;
#52898=CARTESIAN_POINT('Origin',(2.5,20.7239970885482,-41.7772566077985)) ;
#52899=CARTESIAN_POINT('',(2.5,17.6739726500299,-43.1383740271251)) ;
#52900=CARTESIAN_POINT('Origin',(2.5,18.9559612505438,-42.5757860534247)) ;
#52901=CARTESIAN_POINT('Origin',(2.5,17.1794913326873,-43.355372245549)) ;
#52902=CARTESIAN_POINT('Origin',(30.5,-1.22984433837137E-12,2.5666196720605E-12)) ;
#52903=CARTESIAN_POINT('',(30.5,17.6739726500299,-43.1383740271251)) ;
#52904=CARTESIAN_POINT('Origin',(30.5,17.1794913326873,-43.355372245549)) ;
#52905=CARTESIAN_POINT('',(30.5,20.2318634016821,-41.9995276906041)) ;
#52906=CARTESIAN_POINT('Origin',(30.5,18.9559612505438,-42.5757860534247)) ;
#52907=CARTESIAN_POINT('Origin',(30.5,20.7239970885482,-41.7772566077985)) ;
#52908=CARTESIAN_POINT('Origin',(30.5,20.7239970885482,-41.7772566077985)) ;
#52909=CARTESIAN_POINT('',(30.5,20.2318634016821,-41.9995276906041)) ;
#52910=CARTESIAN_POINT('Origin',(30.5,18.9559612505438,-42.5757860534247)) ;
#52911=CARTESIAN_POINT('',(30.5,17.6739726500299,-43.1383740271251)) ;
#52912=CARTESIAN_POINT('Origin',(30.5,17.1794913326873,-43.355372245549)) ;
#52913=CARTESIAN_POINT('Origin',(2.5,-9.54822312292023E-13,2.68111319969549E-12)) ;
#52914=CARTESIAN_POINT('',(2.5,15.7308850496068,-43.8842554738508)) ;
#52915=CARTESIAN_POINT('Origin',(2.5,16.2435564313579,-43.7146439933037)) ;
#52916=CARTESIAN_POINT('',(2.5,13.0679648336741,-44.7494907015041)) ;
#52917=CARTESIAN_POINT('Origin',(2.5,14.4017370228415,-44.3239889419266)) ;
#52918=CARTESIAN_POINT('Origin',(2.5,12.5535098464227,-44.9136128087662)) ;
#52919=CARTESIAN_POINT('Origin',(30.5,-9.54822312292023E-13,2.68111319969549E-12)) ;
#52920=CARTESIAN_POINT('',(30.5,13.0679648336741,-44.7494907015041)) ;
#52921=CARTESIAN_POINT('Origin',(30.5,12.5535098464227,-44.9136128087662)) ;
#52922=CARTESIAN_POINT('',(30.5,15.7308850496068,-43.8842554738508)) ;
#52923=CARTESIAN_POINT('Origin',(30.5,14.4017370228415,-44.3239889419266)) ;
#52924=CARTESIAN_POINT('Origin',(30.5,16.2435564313579,-43.7146439933037)) ;
#52925=CARTESIAN_POINT('Origin',(30.5,16.2435564313579,-43.7146439933037)) ;
#52926=CARTESIAN_POINT('',(30.5,15.7308850496068,-43.8842554738508)) ;
#52927=CARTESIAN_POINT('Origin',(30.5,14.4017370228415,-44.3239889419266)) ;
#52928=CARTESIAN_POINT('',(30.5,13.0679648336741,-44.7494907015041)) ;
#52929=CARTESIAN_POINT('Origin',(30.5,12.5535098464227,-44.9136128087662)) ;
#52930=CARTESIAN_POINT('Origin',(2.5,-6.69339053149789E-13,2.76623189005561E-12)) ;
#52931=CARTESIAN_POINT('',(2.5,11.0575558290286,-45.2881781707551)) ;
#52932=CARTESIAN_POINT('Origin',(2.5,11.585147970723,-45.173084591341)) ;
#52933=CARTESIAN_POINT('',(2.5,8.31878165995311,-45.8703225913245)) ;
#52934=CARTESIAN_POINT('Origin',(2.5,9.68972435055971,-45.5865689321897)) ;
#52935=CARTESIAN_POINT('Origin',(2.5,7.78998947928984,-45.9797704312729)) ;
#52936=CARTESIAN_POINT('Origin',(30.5,-6.69339053149789E-13,2.76623189005561E-12)) ;
#52937=CARTESIAN_POINT('',(30.5,8.31878165995311,-45.8703225913245)) ;
#52938=CARTESIAN_POINT('Origin',(30.5,7.78998947928984,-45.9797704312729)) ;
#52939=CARTESIAN_POINT('',(30.5,11.0575558290286,-45.2881781707551)) ;
#52940=CARTESIAN_POINT('Origin',(30.5,9.68972435055971,-45.5865689321897)) ;
#52941=CARTESIAN_POINT('Origin',(30.5,11.585147970723,-45.173084591341)) ;
#52942=CARTESIAN_POINT('Origin',(30.5,11.585147970723,-45.173084591341)) ;
#52943=CARTESIAN_POINT('',(30.5,11.0575558290286,-45.2881781707551)) ;
#52944=CARTESIAN_POINT('Origin',(30.5,9.68972435055971,-45.5865689321897)) ;
#52945=CARTESIAN_POINT('',(30.5,8.31878165995311,-45.8703225913245)) ;
#52946=CARTESIAN_POINT('Origin',(30.5,7.78998947928984,-45.9797704312729)) ;
#52947=CARTESIAN_POINT('Origin',(2.5,-3.76522375273045E-13,2.82104316495704E-12)) ;
#52948=CARTESIAN_POINT('',(2.5,6.26307771284532,-46.19591411046)) ;
#52949=CARTESIAN_POINT('Origin',(2.5,6.79981020457273,-46.1365994215198)) ;
#52950=CARTESIAN_POINT('',(2.5,3.47845617354872,-46.4885896278522)) ;
#52951=CARTESIAN_POINT('Origin',(2.5,4.871549030588,-46.3496929336289)) ;
#52952=CARTESIAN_POINT('Origin',(2.5,2.94112035726179,-46.5421640670489)) ;
#52953=CARTESIAN_POINT('Origin',(30.5,-3.76522375273045E-13,2.82104316495704E-12)) ;
#52954=CARTESIAN_POINT('',(30.5,3.47845617354872,-46.4885896278522)) ;
#52955=CARTESIAN_POINT('Origin',(30.5,2.94112035726179,-46.5421640670489)) ;
#52956=CARTESIAN_POINT('',(30.5,6.26307771284532,-46.19591411046)) ;
#52957=CARTESIAN_POINT('Origin',(30.5,4.871549030588,-46.3496929336289)) ;
#52958=CARTESIAN_POINT('Origin',(30.5,6.79981020457273,-46.1365994215198)) ;
#52959=CARTESIAN_POINT('Origin',(30.5,6.79981020457273,-46.1365994215198)) ;
#52960=CARTESIAN_POINT('',(30.5,6.26307771284532,-46.19591411046)) ;
#52961=CARTESIAN_POINT('Origin',(30.5,4.871549030588,-46.3496929336289)) ;
#52962=CARTESIAN_POINT('',(30.5,3.47845617354872,-46.4885896278522)) ;
#52963=CARTESIAN_POINT('Origin',(30.5,2.94112035726179,-46.5421640670489)) ;
#52964=CARTESIAN_POINT('Origin',(2.5,-7.95804394604355E-14,2.84494650060196E-12)) ;
#52965=CARTESIAN_POINT('',(2.5,1.39998000660681,-46.5975179480543)) ;
#52966=CARTESIAN_POINT('Origin',(2.5,1.93997229486942,-46.5946320137324)) ;
#52967=CARTESIAN_POINT('',(2.5,-1.39998000660683,-46.5975179480543)) ;
#52968=CARTESIAN_POINT('Origin',(2.5,-8.56119961113762E-15,-46.6049999999905)) ;
#52969=CARTESIAN_POINT('Origin',(2.5,-1.93997229486942,-46.5946320137324)) ;
#52970=CARTESIAN_POINT('Origin',(30.5,-7.95804394604355E-14,2.84494650060196E-12)) ;
#52971=CARTESIAN_POINT('',(30.5,-1.39998000660683,-46.5975179480543)) ;
#52972=CARTESIAN_POINT('Origin',(30.5,-1.93997229486942,-46.5946320137324)) ;
#52973=CARTESIAN_POINT('',(30.5,1.39998000660681,-46.5975179480543)) ;
#52974=CARTESIAN_POINT('Origin',(30.5,-8.56119961113762E-15,-46.6049999999905)) ;
#52975=CARTESIAN_POINT('Origin',(30.5,1.93997229486942,-46.5946320137324)) ;
#52976=CARTESIAN_POINT('Origin',(30.5,1.93997229486942,-46.5946320137324)) ;
#52977=CARTESIAN_POINT('',(30.5,1.39998000660681,-46.5975179480543)) ;
#52978=CARTESIAN_POINT('Origin',(30.5,-8.56119961113762E-15,-46.6049999999905)) ;
#52979=CARTESIAN_POINT('',(30.5,-1.39998000660683,-46.5975179480543)) ;
#52980=CARTESIAN_POINT('Origin',(30.5,-1.93997229486942,-46.5946320137324)) ;
#52981=CARTESIAN_POINT('Origin',(2.5,2.18233396300178E-13,2.83768000704297E-12)) ;
#52982=CARTESIAN_POINT('',(2.5,-3.47845617354871,-46.4885896278521)) ;
#52983=CARTESIAN_POINT('Origin',(2.5,-2.94112035726177,-46.5421640670489)) ;
#52984=CARTESIAN_POINT('',(2.5,-6.26307771284532,-46.1959141104601)) ;
#52985=CARTESIAN_POINT('Origin',(2.5,-4.87154903058799,-46.349692933629)) ;
#52986=CARTESIAN_POINT('Origin',(2.5,-6.79981020457272,-46.1365994215199)) ;
#52987=CARTESIAN_POINT('Origin',(30.5,2.18233396300178E-13,2.83768000704297E-12)) ;
#52988=CARTESIAN_POINT('',(30.5,-6.26307771284532,-46.1959141104601)) ;
#52989=CARTESIAN_POINT('Origin',(30.5,-6.79981020457272,-46.1365994215199)) ;
#52990=CARTESIAN_POINT('',(30.5,-3.47845617354871,-46.4885896278521)) ;
#52991=CARTESIAN_POINT('Origin',(30.5,-4.87154903058799,-46.349692933629)) ;
#52992=CARTESIAN_POINT('Origin',(30.5,-2.94112035726177,-46.5421640670489)) ;
#52993=CARTESIAN_POINT('Origin',(30.5,-2.94112035726177,-46.5421640670489)) ;
#52994=CARTESIAN_POINT('',(30.5,-3.47845617354871,-46.4885896278521)) ;
#52995=CARTESIAN_POINT('Origin',(30.5,-4.87154903058799,-46.349692933629)) ;
#52996=CARTESIAN_POINT('',(30.5,-6.26307771284532,-46.1959141104601)) ;
#52997=CARTESIAN_POINT('Origin',(30.5,-6.79981020457272,-46.1365994215199)) ;
#52998=CARTESIAN_POINT('Origin',(2.5,5.13656221302656E-13,2.79932329750409E-12)) ;
#52999=CARTESIAN_POINT('',(2.5,-8.31878165995312,-45.8703225913244)) ;
#53000=CARTESIAN_POINT('Origin',(2.5,-7.78998947928983,-45.9797704312728)) ;
#53001=CARTESIAN_POINT('',(2.5,-11.0575558290286,-45.2881781707551)) ;
#53002=CARTESIAN_POINT('Origin',(2.5,-9.68972435055972,-45.5865689321897)) ;
#53003=CARTESIAN_POINT('Origin',(2.5,-11.585147970723,-45.173084591341)) ;
#53004=CARTESIAN_POINT('Origin',(30.5,5.13656221302656E-13,2.79932329750409E-12)) ;
#53005=CARTESIAN_POINT('',(30.5,-11.0575558290286,-45.2881781707551)) ;
#53006=CARTESIAN_POINT('Origin',(30.5,-11.585147970723,-45.173084591341)) ;
#53007=CARTESIAN_POINT('',(30.5,-8.31878165995312,-45.8703225913244)) ;
#53008=CARTESIAN_POINT('Origin',(30.5,-9.68972435055972,-45.5865689321897)) ;
#53009=CARTESIAN_POINT('Origin',(30.5,-7.78998947928983,-45.9797704312728)) ;
#53010=CARTESIAN_POINT('Origin',(30.5,-7.78998947928983,-45.9797704312728)) ;
#53011=CARTESIAN_POINT('',(30.5,-8.31878165995312,-45.8703225913244)) ;
#53012=CARTESIAN_POINT('Origin',(30.5,-9.68972435055972,-45.5865689321897)) ;
#53013=CARTESIAN_POINT('',(30.5,-11.0575558290286,-45.2881781707551)) ;
#53014=CARTESIAN_POINT('Origin',(30.5,-11.585147970723,-45.173084591341)) ;
#53015=CARTESIAN_POINT('Origin',(2.5,8.03451321255064E-13,2.73029661612169E-12)) ;
#53016=CARTESIAN_POINT('',(2.5,-13.0679648336741,-44.7494907015041)) ;
#53017=CARTESIAN_POINT('Origin',(2.5,-12.5535098464227,-44.9136128087662)) ;
#53018=CARTESIAN_POINT('',(2.5,-15.7308850496068,-43.8842554738508)) ;
#53019=CARTESIAN_POINT('Origin',(2.5,-14.4017370228415,-44.3239889419266)) ;
#53020=CARTESIAN_POINT('Origin',(2.5,-16.2435564313579,-43.7146439933038)) ;
#53021=CARTESIAN_POINT('Origin',(30.5,8.03451321255064E-13,2.73029661612169E-12)) ;
#53022=CARTESIAN_POINT('',(30.5,-15.7308850496068,-43.8842554738508)) ;
#53023=CARTESIAN_POINT('Origin',(30.5,-16.2435564313579,-43.7146439933038)) ;
#53024=CARTESIAN_POINT('',(30.5,-13.0679648336741,-44.7494907015041)) ;
#53025=CARTESIAN_POINT('Origin',(30.5,-14.4017370228415,-44.3239889419266)) ;
#53026=CARTESIAN_POINT('Origin',(30.5,-12.5535098464227,-44.9136128087662)) ;
#53027=CARTESIAN_POINT('Origin',(30.5,-12.5535098464227,-44.9136128087662)) ;
#53028=CARTESIAN_POINT('',(30.5,-13.0679648336741,-44.7494907015041)) ;
#53029=CARTESIAN_POINT('Origin',(30.5,-14.4017370228415,-44.3239889419266)) ;
#53030=CARTESIAN_POINT('',(30.5,-15.7308850496068,-43.8842554738508)) ;
#53031=CARTESIAN_POINT('Origin',(30.5,-16.2435564313579,-43.7146439933038)) ;
#53032=CARTESIAN_POINT('Origin',(2.5,2.5666196720605E-12,1.22984433837137E-12)) ;
#53033=CARTESIAN_POINT('',(2.5,-41.9995276906041,-20.2318634016821)) ;
#53034=CARTESIAN_POINT('Origin',(2.5,-41.7772566077985,-20.7239970885482)) ;
#53035=CARTESIAN_POINT('',(2.5,-43.1383740271251,-17.6739726500298)) ;
#53036=CARTESIAN_POINT('Origin',(2.5,-42.5757860534248,-18.9559612505438)) ;
#53037=CARTESIAN_POINT('Origin',(2.5,-43.355372245549,-17.1794913326873)) ;
#53038=CARTESIAN_POINT('Origin',(30.5,2.5666196720605E-12,1.22984433837137E-12)) ;
#53039=CARTESIAN_POINT('',(30.5,-43.1383740271251,-17.6739726500298)) ;
#53040=CARTESIAN_POINT('Origin',(30.5,-43.355372245549,-17.1794913326873)) ;
#53041=CARTESIAN_POINT('',(30.5,-41.9995276906041,-20.2318634016821)) ;
#53042=CARTESIAN_POINT('Origin',(30.5,-42.5757860534248,-18.9559612505438)) ;
#53043=CARTESIAN_POINT('Origin',(30.5,-41.7772566077985,-20.7239970885482)) ;
#53044=CARTESIAN_POINT('Origin',(30.5,-41.7772566077985,-20.7239970885482)) ;
#53045=CARTESIAN_POINT('',(30.5,-41.9995276906041,-20.2318634016821)) ;
#53046=CARTESIAN_POINT('Origin',(30.5,-42.5757860534248,-18.9559612505438)) ;
#53047=CARTESIAN_POINT('',(30.5,-43.1383740271251,-17.6739726500298)) ;
#53048=CARTESIAN_POINT('Origin',(30.5,-43.355372245549,-17.1794913326873)) ;
#53049=CARTESIAN_POINT('Origin',(2.5,2.42400572219872E-12,1.49139193251805E-12)) ;
#53050=CARTESIAN_POINT('',(2.5,-39.654644293013,-24.5111772245389)) ;
#53051=CARTESIAN_POINT('Origin',(2.5,-39.3821488564452,-24.9773812968611)) ;
#53052=CARTESIAN_POINT('',(2.5,-41.0546242996198,-22.0863407235153)) ;
#53053=CARTESIAN_POINT('Origin',(2.5,-40.3611139433656,-23.3024999999952)) ;
#53054=CARTESIAN_POINT('Origin',(2.5,-41.3221211513147,-21.6172507168713)) ;
#53055=CARTESIAN_POINT('Origin',(30.5,2.42400572219872E-12,1.49139193251805E-12)) ;
#53056=CARTESIAN_POINT('',(30.5,-41.0546242996198,-22.0863407235153)) ;
#53057=CARTESIAN_POINT('Origin',(30.5,-41.3221211513147,-21.6172507168713)) ;
#53058=CARTESIAN_POINT('',(30.5,-39.654644293013,-24.5111772245389)) ;
#53059=CARTESIAN_POINT('Origin',(30.5,-40.3611139433656,-23.3024999999952)) ;
#53060=CARTESIAN_POINT('Origin',(30.5,-39.3821488564452,-24.9773812968611)) ;
#53061=CARTESIAN_POINT('Origin',(30.5,-39.3821488564452,-24.9773812968611)) ;
#53062=CARTESIAN_POINT('',(30.5,-39.654644293013,-24.5111772245389)) ;
#53063=CARTESIAN_POINT('Origin',(30.5,-40.3611139433656,-23.3024999999952)) ;
#53064=CARTESIAN_POINT('',(30.5,-41.0546242996198,-22.0863407235153)) ;
#53065=CARTESIAN_POINT('Origin',(30.5,-41.3221211513147,-21.6172507168713)) ;
#53066=CARTESIAN_POINT('Origin',(2.5,2.25483385838873E-12,1.73659952455823E-12)) ;
#53067=CARTESIAN_POINT('',(2.5,-36.8752963142797,-28.5219414604302)) ;
#53068=CARTESIAN_POINT('Origin',(2.5,-36.5555620409762,-28.9571080888326)) ;
#53069=CARTESIAN_POINT('',(2.5,-38.5210715170554,-26.2567262261701)) ;
#53070=CARTESIAN_POINT('Origin',(2.5,-37.7042370228368,-27.3937316830851)) ;
#53071=CARTESIAN_POINT('Origin',(2.5,-38.8361362505368,-25.8181669785007)) ;
#53072=CARTESIAN_POINT('Origin',(30.5,2.25483385838873E-12,1.73659952455823E-12)) ;
#53073=CARTESIAN_POINT('',(30.5,-38.5210715170554,-26.2567262261701)) ;
#53074=CARTESIAN_POINT('Origin',(30.5,-38.8361362505368,-25.8181669785007)) ;
#53075=CARTESIAN_POINT('',(30.5,-36.8752963142797,-28.5219414604302)) ;
#53076=CARTESIAN_POINT('Origin',(30.5,-37.7042370228368,-27.3937316830851)) ;
#53077=CARTESIAN_POINT('Origin',(30.5,-36.5555620409762,-28.9571080888326)) ;
#53078=CARTESIAN_POINT('Origin',(30.5,-36.5555620409762,-28.9571080888326)) ;
#53079=CARTESIAN_POINT('',(30.5,-36.8752963142797,-28.5219414604302)) ;
#53080=CARTESIAN_POINT('Origin',(30.5,-37.7042370228368,-27.3937316830851)) ;
#53081=CARTESIAN_POINT('',(30.5,-38.5210715170554,-26.2567262261701)) ;
#53082=CARTESIAN_POINT('Origin',(30.5,-38.8361362505368,-25.8181669785007)) ;
#53083=CARTESIAN_POINT('Origin',(2.5,2.0609575629719E-12,1.96278056880054E-12)) ;
#53084=CARTESIAN_POINT('',(2.5,-33.6919348724754,-32.220213337081)) ;
#53085=CARTESIAN_POINT('Origin',(2.5,-33.3284648380432,-32.6195747449183)) ;
#53086=CARTESIAN_POINT('',(2.5,-35.5654738138977,-30.1394375417177)) ;
#53087=CARTESIAN_POINT('Origin',(2.5,-34.6342645913669,-31.1848319093482)) ;
#53088=CARTESIAN_POINT('Origin',(2.5,-35.924654514014,-29.7362139999149)) ;
#53089=CARTESIAN_POINT('Origin',(30.5,2.0609575629719E-12,1.96278056880054E-12)) ;
#53090=CARTESIAN_POINT('',(30.5,-35.5654738138977,-30.1394375417177)) ;
#53091=CARTESIAN_POINT('Origin',(30.5,-35.924654514014,-29.7362139999149)) ;
#53092=CARTESIAN_POINT('',(30.5,-33.6919348724754,-32.220213337081)) ;
#53093=CARTESIAN_POINT('Origin',(30.5,-34.6342645913669,-31.1848319093482)) ;
#53094=CARTESIAN_POINT('Origin',(30.5,-33.3284648380432,-32.6195747449183)) ;
#53095=CARTESIAN_POINT('Origin',(30.5,-33.3284648380432,-32.6195747449183)) ;
#53096=CARTESIAN_POINT('',(30.5,-33.6919348724754,-32.220213337081)) ;
#53097=CARTESIAN_POINT('Origin',(30.5,-34.6342645913669,-31.1848319093482)) ;
#53098=CARTESIAN_POINT('',(30.5,-35.5654738138977,-30.1394375417177)) ;
#53099=CARTESIAN_POINT('Origin',(30.5,-35.924654514014,-29.7362139999149)) ;
#53100=CARTESIAN_POINT('Origin',(2.5,1.84450098521206E-12,2.16745697839284E-12)) ;
#53101=CARTESIAN_POINT('',(2.5,-30.1394375417177,-35.5654738138976)) ;
#53102=CARTESIAN_POINT('Origin',(2.5,-29.7362139999149,-35.9246545140139)) ;
#53103=CARTESIAN_POINT('',(2.5,-32.220213337081,-33.6919348724755)) ;
#53104=CARTESIAN_POINT('Origin',(2.5,-31.1848319093483,-34.6342645913669)) ;
#53105=CARTESIAN_POINT('Origin',(2.5,-32.6195747449184,-33.3284648380432)) ;
#53106=CARTESIAN_POINT('Origin',(30.5,1.84450098521206E-12,2.16745697839284E-12)) ;
#53107=CARTESIAN_POINT('',(30.5,-32.220213337081,-33.6919348724755)) ;
#53108=CARTESIAN_POINT('Origin',(30.5,-32.6195747449184,-33.3284648380432)) ;
#53109=CARTESIAN_POINT('',(30.5,-30.1394375417177,-35.5654738138976)) ;
#53110=CARTESIAN_POINT('Origin',(30.5,-31.1848319093483,-34.6342645913669)) ;
#53111=CARTESIAN_POINT('Origin',(30.5,-29.7362139999149,-35.9246545140139)) ;
#53112=CARTESIAN_POINT('Origin',(30.5,-29.7362139999149,-35.9246545140139)) ;
#53113=CARTESIAN_POINT('',(30.5,-30.1394375417177,-35.5654738138976)) ;
#53114=CARTESIAN_POINT('Origin',(30.5,-31.1848319093483,-34.6342645913669)) ;
#53115=CARTESIAN_POINT('',(30.5,-32.220213337081,-33.6919348724755)) ;
#53116=CARTESIAN_POINT('Origin',(30.5,-32.6195747449184,-33.3284648380432)) ;
#53117=CARTESIAN_POINT('Origin',(2.5,1.60783566867159E-12,2.34838627576032E-12)) ;
#53118=CARTESIAN_POINT('',(2.5,-26.2567262261701,-38.5210715170554)) ;
#53119=CARTESIAN_POINT('Origin',(2.5,-25.8181669785007,-38.8361362505367)) ;
#53120=CARTESIAN_POINT('',(2.5,-28.5219414604302,-36.8752963142798)) ;
#53121=CARTESIAN_POINT('Origin',(2.5,-27.3937316830851,-37.7042370228368)) ;
#53122=CARTESIAN_POINT('Origin',(2.5,-28.9571080888326,-36.5555620409763)) ;
#53123=CARTESIAN_POINT('Origin',(30.5,1.60783566867159E-12,2.34838627576032E-12)) ;
#53124=CARTESIAN_POINT('',(30.5,-28.5219414604302,-36.8752963142798)) ;
#53125=CARTESIAN_POINT('Origin',(30.5,-28.9571080888326,-36.5555620409763)) ;
#53126=CARTESIAN_POINT('',(30.5,-26.2567262261701,-38.5210715170554)) ;
#53127=CARTESIAN_POINT('Origin',(30.5,-27.3937316830851,-37.7042370228368)) ;
#53128=CARTESIAN_POINT('Origin',(30.5,-25.8181669785007,-38.8361362505367)) ;
#53129=CARTESIAN_POINT('Origin',(30.5,-25.8181669785007,-38.8361362505367)) ;
#53130=CARTESIAN_POINT('',(30.5,-26.2567262261701,-38.5210715170554)) ;
#53131=CARTESIAN_POINT('Origin',(30.5,-27.3937316830851,-37.7042370228368)) ;
#53132=CARTESIAN_POINT('',(30.5,-28.5219414604302,-36.8752963142798)) ;
#53133=CARTESIAN_POINT('Origin',(30.5,-28.9571080888326,-36.5555620409763)) ;
#53134=CARTESIAN_POINT('Origin',(2.5,1.35355456808392E-12,2.50358616165916E-12)) ;
#53135=CARTESIAN_POINT('',(2.5,-22.0863407235154,-41.0546242996198)) ;
#53136=CARTESIAN_POINT('Origin',(2.5,-21.6172507168713,-41.3221211513146)) ;
#53137=CARTESIAN_POINT('',(2.5,-24.511177224539,-39.654644293013)) ;
#53138=CARTESIAN_POINT('Origin',(2.5,-23.3024999999953,-40.3611139433655)) ;
#53139=CARTESIAN_POINT('Origin',(2.5,-24.9773812968612,-39.3821488564453)) ;
#53140=CARTESIAN_POINT('Origin',(30.5,1.35355456808392E-12,2.50358616165916E-12)) ;
#53141=CARTESIAN_POINT('',(30.5,-24.511177224539,-39.654644293013)) ;
#53142=CARTESIAN_POINT('Origin',(30.5,-24.9773812968612,-39.3821488564453)) ;
#53143=CARTESIAN_POINT('',(30.5,-22.0863407235154,-41.0546242996198)) ;
#53144=CARTESIAN_POINT('Origin',(30.5,-23.3024999999953,-40.3611139433655)) ;
#53145=CARTESIAN_POINT('Origin',(30.5,-21.6172507168713,-41.3221211513146)) ;
#53146=CARTESIAN_POINT('Origin',(30.5,-21.6172507168713,-41.3221211513146)) ;
#53147=CARTESIAN_POINT('',(30.5,-22.0863407235154,-41.0546242996198)) ;
#53148=CARTESIAN_POINT('Origin',(30.5,-23.3024999999953,-40.3611139433655)) ;
#53149=CARTESIAN_POINT('',(30.5,-24.511177224539,-39.654644293013)) ;
#53150=CARTESIAN_POINT('Origin',(30.5,-24.9773812968612,-39.3821488564453)) ;
#53151=CARTESIAN_POINT('Origin',(2.5,1.0844436403988E-12,2.63135623366177E-12)) ;
#53152=CARTESIAN_POINT('',(2.5,-17.6739726500298,-43.1383740271251)) ;
#53153=CARTESIAN_POINT('Origin',(2.5,-17.1794913326873,-43.355372245549)) ;
#53154=CARTESIAN_POINT('',(2.5,-20.2318634016821,-41.9995276906041)) ;
#53155=CARTESIAN_POINT('Origin',(2.5,-18.9559612505438,-42.5757860534248)) ;
#53156=CARTESIAN_POINT('Origin',(2.5,-20.7239970885482,-41.7772566077985)) ;
#53157=CARTESIAN_POINT('Origin',(30.5,1.0844436403988E-12,2.63135623366177E-12)) ;
#53158=CARTESIAN_POINT('',(30.5,-20.2318634016821,-41.9995276906041)) ;
#53159=CARTESIAN_POINT('Origin',(30.5,-20.7239970885482,-41.7772566077985)) ;
#53160=CARTESIAN_POINT('',(30.5,-17.6739726500298,-43.1383740271251)) ;
#53161=CARTESIAN_POINT('Origin',(30.5,-18.9559612505438,-42.5757860534248)) ;
#53162=CARTESIAN_POINT('Origin',(30.5,-17.1794913326873,-43.355372245549)) ;
#53163=CARTESIAN_POINT('Origin',(30.5,-17.1794913326873,-43.355372245549)) ;
#53164=CARTESIAN_POINT('',(30.5,-17.6739726500298,-43.1383740271251)) ;
#53165=CARTESIAN_POINT('Origin',(30.5,-18.9559612505438,-42.5757860534248)) ;
#53166=CARTESIAN_POINT('',(30.5,-20.2318634016821,-41.9995276906041)) ;
#53167=CARTESIAN_POINT('Origin',(30.5,-20.7239970885482,-41.7772566077985)) ;
#53168=CARTESIAN_POINT('Origin',(2.5,2.68111319969549E-12,9.54822312292024E-13)) ;
#53169=CARTESIAN_POINT('',(2.5,-43.8842554738508,-15.7308850496068)) ;
#53170=CARTESIAN_POINT('Origin',(2.5,-43.7146439933037,-16.2435564313579)) ;
#53171=CARTESIAN_POINT('',(2.5,-44.7494907015041,-13.0679648336741)) ;
#53172=CARTESIAN_POINT('Origin',(2.5,-44.3239889419266,-14.4017370228415)) ;
#53173=CARTESIAN_POINT('Origin',(2.5,-44.9136128087662,-12.5535098464227)) ;
#53174=CARTESIAN_POINT('Origin',(30.5,2.68111319969549E-12,9.54822312292024E-13)) ;
#53175=CARTESIAN_POINT('',(30.5,-44.7494907015041,-13.0679648336741)) ;
#53176=CARTESIAN_POINT('Origin',(30.5,-44.9136128087662,-12.5535098464227)) ;
#53177=CARTESIAN_POINT('',(30.5,-43.8842554738508,-15.7308850496068)) ;
#53178=CARTESIAN_POINT('Origin',(30.5,-44.3239889419266,-14.4017370228415)) ;
#53179=CARTESIAN_POINT('Origin',(30.5,-43.7146439933037,-16.2435564313579)) ;
#53180=CARTESIAN_POINT('Origin',(30.5,-43.7146439933037,-16.2435564313579)) ;
#53181=CARTESIAN_POINT('',(30.5,-43.8842554738508,-15.7308850496068)) ;
#53182=CARTESIAN_POINT('Origin',(30.5,-44.3239889419266,-14.4017370228415)) ;
#53183=CARTESIAN_POINT('',(30.5,-44.7494907015041,-13.0679648336741)) ;
#53184=CARTESIAN_POINT('Origin',(30.5,-44.9136128087662,-12.5535098464227)) ;
#53185=CARTESIAN_POINT('Origin',(2.5,2.76623189005561E-12,6.69339053149788E-13)) ;
#53186=CARTESIAN_POINT('',(2.5,-45.2881781707551,-11.0575558290286)) ;
#53187=CARTESIAN_POINT('Origin',(2.5,-45.173084591341,-11.585147970723)) ;
#53188=CARTESIAN_POINT('',(2.5,-45.8703225913245,-8.31878165995309)) ;
#53189=CARTESIAN_POINT('Origin',(2.5,-45.5865689321897,-9.68972435055969)) ;
#53190=CARTESIAN_POINT('Origin',(2.5,-45.9797704312729,-7.78998947928983)) ;
#53191=CARTESIAN_POINT('Origin',(30.5,2.76623189005561E-12,6.69339053149788E-13)) ;
#53192=CARTESIAN_POINT('',(30.5,-45.8703225913245,-8.31878165995309)) ;
#53193=CARTESIAN_POINT('Origin',(30.5,-45.9797704312729,-7.78998947928983)) ;
#53194=CARTESIAN_POINT('',(30.5,-45.2881781707551,-11.0575558290286)) ;
#53195=CARTESIAN_POINT('Origin',(30.5,-45.5865689321897,-9.68972435055969)) ;
#53196=CARTESIAN_POINT('Origin',(30.5,-45.173084591341,-11.585147970723)) ;
#53197=CARTESIAN_POINT('Origin',(30.5,-45.173084591341,-11.585147970723)) ;
#53198=CARTESIAN_POINT('',(30.5,-45.2881781707551,-11.0575558290286)) ;
#53199=CARTESIAN_POINT('Origin',(30.5,-45.5865689321897,-9.68972435055969)) ;
#53200=CARTESIAN_POINT('',(30.5,-45.8703225913245,-8.31878165995309)) ;
#53201=CARTESIAN_POINT('Origin',(30.5,-45.9797704312729,-7.78998947928983)) ;
#53202=CARTESIAN_POINT('Origin',(2.5,2.82104316495704E-12,3.76522375273043E-13)) ;
#53203=CARTESIAN_POINT('',(2.5,-46.1959141104601,-6.2630777128453)) ;
#53204=CARTESIAN_POINT('Origin',(2.5,-46.1365994215198,-6.79981020457271)) ;
#53205=CARTESIAN_POINT('',(2.5,-46.4885896278522,-3.4784561735487)) ;
#53206=CARTESIAN_POINT('Origin',(2.5,-46.349692933629,-4.87154903058798)) ;
#53207=CARTESIAN_POINT('Origin',(2.5,-46.5421640670489,-2.94112035726177)) ;
#53208=CARTESIAN_POINT('Origin',(30.5,2.82104316495704E-12,3.76522375273043E-13)) ;
#53209=CARTESIAN_POINT('',(30.5,-46.4885896278522,-3.4784561735487)) ;
#53210=CARTESIAN_POINT('Origin',(30.5,-46.5421640670489,-2.94112035726177)) ;
#53211=CARTESIAN_POINT('',(30.5,-46.1959141104601,-6.2630777128453)) ;
#53212=CARTESIAN_POINT('Origin',(30.5,-46.349692933629,-4.87154903058798)) ;
#53213=CARTESIAN_POINT('Origin',(30.5,-46.1365994215198,-6.79981020457271)) ;
#53214=CARTESIAN_POINT('Origin',(30.5,-46.1365994215198,-6.79981020457271)) ;
#53215=CARTESIAN_POINT('',(30.5,-46.1959141104601,-6.2630777128453)) ;
#53216=CARTESIAN_POINT('Origin',(30.5,-46.349692933629,-4.87154903058798)) ;
#53217=CARTESIAN_POINT('',(30.5,-46.4885896278522,-3.4784561735487)) ;
#53218=CARTESIAN_POINT('Origin',(30.5,-46.5421640670489,-2.94112035726177)) ;
#53219=CARTESIAN_POINT('Origin',(2.5,2.84494650060196E-12,7.95804394604357E-14)) ;
#53220=CARTESIAN_POINT('',(2.5,-46.5975179480543,-1.39998000660681)) ;
#53221=CARTESIAN_POINT('Origin',(2.5,-46.5946320137324,-1.93997229486942)) ;
#53222=CARTESIAN_POINT('',(2.5,-46.5975179480543,1.39998000660682)) ;
#53223=CARTESIAN_POINT('Origin',(2.5,-46.6049999999905,5.70746640742508E-15)) ;
#53224=CARTESIAN_POINT('Origin',(2.5,-46.5946320137324,1.93997229486942)) ;
#53225=CARTESIAN_POINT('Origin',(30.5,2.84494650060196E-12,7.95804394604357E-14)) ;
#53226=CARTESIAN_POINT('',(30.5,-46.5975179480543,1.39998000660682)) ;
#53227=CARTESIAN_POINT('Origin',(30.5,-46.5946320137324,1.93997229486942)) ;
#53228=CARTESIAN_POINT('',(30.5,-46.5975179480543,-1.39998000660681)) ;
#53229=CARTESIAN_POINT('Origin',(30.5,-46.6049999999905,5.70746640742508E-15)) ;
#53230=CARTESIAN_POINT('Origin',(30.5,-46.5946320137324,-1.93997229486942)) ;
#53231=CARTESIAN_POINT('Origin',(30.5,-46.5946320137324,-1.93997229486942)) ;
#53232=CARTESIAN_POINT('',(30.5,-46.5975179480543,-1.39998000660681)) ;
#53233=CARTESIAN_POINT('Origin',(30.5,-46.6049999999905,5.70746640742508E-15)) ;
#53234=CARTESIAN_POINT('',(30.5,-46.5975179480543,1.39998000660682)) ;
#53235=CARTESIAN_POINT('Origin',(30.5,-46.5946320137324,1.93997229486942)) ;
#53236=CARTESIAN_POINT('Origin',(2.5,2.83768000704297E-12,-2.18233396300179E-13)) ;
#53237=CARTESIAN_POINT('',(2.5,-46.4885896278521,3.47845617354873)) ;
#53238=CARTESIAN_POINT('Origin',(2.5,-46.5421640670489,2.94112035726179)) ;
#53239=CARTESIAN_POINT('',(2.5,-46.1959141104601,6.26307771284533)) ;
#53240=CARTESIAN_POINT('Origin',(2.5,-46.3496929336289,4.87154903058801)) ;
#53241=CARTESIAN_POINT('Origin',(2.5,-46.1365994215199,6.79981020457274)) ;
#53242=CARTESIAN_POINT('Origin',(30.5,2.83768000704297E-12,-2.18233396300179E-13)) ;
#53243=CARTESIAN_POINT('',(30.5,-46.1959141104601,6.26307771284533)) ;
#53244=CARTESIAN_POINT('Origin',(30.5,-46.1365994215199,6.79981020457274)) ;
#53245=CARTESIAN_POINT('',(30.5,-46.4885896278521,3.47845617354873)) ;
#53246=CARTESIAN_POINT('Origin',(30.5,-46.3496929336289,4.87154903058801)) ;
#53247=CARTESIAN_POINT('Origin',(30.5,-46.5421640670489,2.94112035726179)) ;
#53248=CARTESIAN_POINT('Origin',(30.5,-46.5421640670489,2.94112035726179)) ;
#53249=CARTESIAN_POINT('',(30.5,-46.4885896278521,3.47845617354873)) ;
#53250=CARTESIAN_POINT('Origin',(30.5,-46.3496929336289,4.87154903058801)) ;
#53251=CARTESIAN_POINT('',(30.5,-46.1959141104601,6.26307771284533)) ;
#53252=CARTESIAN_POINT('Origin',(30.5,-46.1365994215199,6.79981020457274)) ;
#53253=CARTESIAN_POINT('Origin',(2.5,2.79932329750409E-12,-5.13656221302654E-13)) ;
#53254=CARTESIAN_POINT('',(2.5,-45.8703225913244,8.3187816599531)) ;
#53255=CARTESIAN_POINT('Origin',(2.5,-45.9797704312728,7.78998947928981)) ;
#53256=CARTESIAN_POINT('',(2.5,-45.2881781707551,11.0575558290286)) ;
#53257=CARTESIAN_POINT('Origin',(2.5,-45.5865689321897,9.6897243505597)) ;
#53258=CARTESIAN_POINT('Origin',(2.5,-45.1730845913411,11.585147970723)) ;
#53259=CARTESIAN_POINT('Origin',(30.5,2.79932329750409E-12,-5.13656221302654E-13)) ;
#53260=CARTESIAN_POINT('',(30.5,-45.2881781707551,11.0575558290286)) ;
#53261=CARTESIAN_POINT('Origin',(30.5,-45.1730845913411,11.585147970723)) ;
#53262=CARTESIAN_POINT('',(30.5,-45.8703225913244,8.3187816599531)) ;
#53263=CARTESIAN_POINT('Origin',(30.5,-45.5865689321897,9.6897243505597)) ;
#53264=CARTESIAN_POINT('Origin',(30.5,-45.9797704312728,7.78998947928981)) ;
#53265=CARTESIAN_POINT('Origin',(30.5,-45.9797704312728,7.78998947928981)) ;
#53266=CARTESIAN_POINT('',(30.5,-45.8703225913244,8.3187816599531)) ;
#53267=CARTESIAN_POINT('Origin',(30.5,-45.5865689321897,9.6897243505597)) ;
#53268=CARTESIAN_POINT('',(30.5,-45.2881781707551,11.0575558290286)) ;
#53269=CARTESIAN_POINT('Origin',(30.5,-45.1730845913411,11.585147970723)) ;
#53270=CARTESIAN_POINT('Origin',(2.5,2.73029661612169E-12,-8.03451321255064E-13)) ;
#53271=CARTESIAN_POINT('',(2.5,-44.7494907015041,13.0679648336741)) ;
#53272=CARTESIAN_POINT('Origin',(2.5,-44.9136128087662,12.5535098464227)) ;
#53273=CARTESIAN_POINT('',(2.5,-43.8842554738508,15.7308850496068)) ;
#53274=CARTESIAN_POINT('Origin',(2.5,-44.3239889419266,14.4017370228415)) ;
#53275=CARTESIAN_POINT('Origin',(2.5,-43.7146439933038,16.2435564313579)) ;
#53276=CARTESIAN_POINT('Origin',(30.5,2.73029661612169E-12,-8.03451321255064E-13)) ;
#53277=CARTESIAN_POINT('',(30.5,-43.8842554738508,15.7308850496068)) ;
#53278=CARTESIAN_POINT('Origin',(30.5,-43.7146439933038,16.2435564313579)) ;
#53279=CARTESIAN_POINT('',(30.5,-44.7494907015041,13.0679648336741)) ;
#53280=CARTESIAN_POINT('Origin',(30.5,-44.3239889419266,14.4017370228415)) ;
#53281=CARTESIAN_POINT('Origin',(30.5,-44.9136128087662,12.5535098464227)) ;
#53282=CARTESIAN_POINT('Origin',(30.5,-44.9136128087662,12.5535098464227)) ;
#53283=CARTESIAN_POINT('',(30.5,-44.7494907015041,13.0679648336741)) ;
#53284=CARTESIAN_POINT('Origin',(30.5,-44.3239889419266,14.4017370228415)) ;
#53285=CARTESIAN_POINT('',(30.5,-43.8842554738508,15.7308850496068)) ;
#53286=CARTESIAN_POINT('Origin',(30.5,-43.7146439933038,16.2435564313579)) ;
#53287=CARTESIAN_POINT('Origin',(2.5,2.63135623366177E-12,-1.08444364039881E-12)) ;
#53288=CARTESIAN_POINT('',(2.5,-43.1383740271251,17.6739726500298)) ;
#53289=CARTESIAN_POINT('Origin',(2.5,-43.355372245549,17.1794913326873)) ;
#53290=CARTESIAN_POINT('',(2.5,-41.9995276906041,20.2318634016821)) ;
#53291=CARTESIAN_POINT('Origin',(2.5,-42.5757860534247,18.9559612505438)) ;
#53292=CARTESIAN_POINT('Origin',(2.5,-41.7772566077985,20.7239970885482)) ;
#53293=CARTESIAN_POINT('Origin',(30.5,2.63135623366177E-12,-1.08444364039881E-12)) ;
#53294=CARTESIAN_POINT('',(30.5,-41.9995276906041,20.2318634016821)) ;
#53295=CARTESIAN_POINT('Origin',(30.5,-41.7772566077985,20.7239970885482)) ;
#53296=CARTESIAN_POINT('',(30.5,-43.1383740271251,17.6739726500298)) ;
#53297=CARTESIAN_POINT('Origin',(30.5,-42.5757860534247,18.9559612505438)) ;
#53298=CARTESIAN_POINT('Origin',(30.5,-43.355372245549,17.1794913326873)) ;
#53299=CARTESIAN_POINT('Origin',(30.5,-43.355372245549,17.1794913326873)) ;
#53300=CARTESIAN_POINT('',(30.5,-43.1383740271251,17.6739726500298)) ;
#53301=CARTESIAN_POINT('Origin',(30.5,-42.5757860534247,18.9559612505438)) ;
#53302=CARTESIAN_POINT('',(30.5,-41.9995276906041,20.2318634016821)) ;
#53303=CARTESIAN_POINT('Origin',(30.5,-41.7772566077985,20.7239970885482)) ;
#53304=CARTESIAN_POINT('Origin',(2.5,2.50358616165916E-12,-1.35355456808391E-12)) ;
#53305=CARTESIAN_POINT('',(2.5,-41.0546242996198,22.0863407235153)) ;
#53306=CARTESIAN_POINT('Origin',(2.5,-41.3221211513146,21.6172507168713)) ;
#53307=CARTESIAN_POINT('',(2.5,-39.654644293013,24.511177224539)) ;
#53308=CARTESIAN_POINT('Origin',(2.5,-40.3611139433656,23.3024999999953)) ;
#53309=CARTESIAN_POINT('Origin',(2.5,-39.3821488564453,24.9773812968611)) ;
#53310=CARTESIAN_POINT('Origin',(30.5,2.50358616165916E-12,-1.35355456808391E-12)) ;
#53311=CARTESIAN_POINT('',(30.5,-39.654644293013,24.511177224539)) ;
#53312=CARTESIAN_POINT('Origin',(30.5,-39.3821488564453,24.9773812968611)) ;
#53313=CARTESIAN_POINT('',(30.5,-41.0546242996198,22.0863407235153)) ;
#53314=CARTESIAN_POINT('Origin',(30.5,-40.3611139433656,23.3024999999953)) ;
#53315=CARTESIAN_POINT('Origin',(30.5,-41.3221211513146,21.6172507168713)) ;
#53316=CARTESIAN_POINT('Origin',(30.5,-41.3221211513146,21.6172507168713)) ;
#53317=CARTESIAN_POINT('',(30.5,-41.0546242996198,22.0863407235153)) ;
#53318=CARTESIAN_POINT('Origin',(30.5,-40.3611139433656,23.3024999999953)) ;
#53319=CARTESIAN_POINT('',(30.5,-39.654644293013,24.511177224539)) ;
#53320=CARTESIAN_POINT('Origin',(30.5,-39.3821488564453,24.9773812968611)) ;
#53321=CARTESIAN_POINT('Origin',(2.5,2.34838627576032E-12,-1.6078356686716E-12)) ;
#53322=CARTESIAN_POINT('',(2.5,-38.5210715170553,26.2567262261701)) ;
#53323=CARTESIAN_POINT('Origin',(2.5,-38.8361362505367,25.8181669785007)) ;
#53324=CARTESIAN_POINT('',(2.5,-36.8752963142798,28.5219414604302)) ;
#53325=CARTESIAN_POINT('Origin',(2.5,-37.7042370228367,27.3937316830852)) ;
#53326=CARTESIAN_POINT('Origin',(2.5,-36.5555620409763,28.9571080888326)) ;
#53327=CARTESIAN_POINT('Origin',(30.5,2.34838627576032E-12,-1.6078356686716E-12)) ;
#53328=CARTESIAN_POINT('',(30.5,-36.8752963142798,28.5219414604302)) ;
#53329=CARTESIAN_POINT('Origin',(30.5,-36.5555620409763,28.9571080888326)) ;
#53330=CARTESIAN_POINT('',(30.5,-38.5210715170553,26.2567262261701)) ;
#53331=CARTESIAN_POINT('Origin',(30.5,-37.7042370228367,27.3937316830852)) ;
#53332=CARTESIAN_POINT('Origin',(30.5,-38.8361362505367,25.8181669785007)) ;
#53333=CARTESIAN_POINT('Origin',(30.5,-38.8361362505367,25.8181669785007)) ;
#53334=CARTESIAN_POINT('',(30.5,-38.5210715170553,26.2567262261701)) ;
#53335=CARTESIAN_POINT('Origin',(30.5,-37.7042370228367,27.3937316830852)) ;
#53336=CARTESIAN_POINT('',(30.5,-36.8752963142798,28.5219414604302)) ;
#53337=CARTESIAN_POINT('Origin',(30.5,-36.5555620409763,28.9571080888326)) ;
#53338=CARTESIAN_POINT('Origin',(2.5,1.96278056880054E-12,-2.06095756297191E-12)) ;
#53339=CARTESIAN_POINT('',(2.5,-32.220213337081,33.6919348724755)) ;
#53340=CARTESIAN_POINT('Origin',(2.5,-32.6195747449183,33.3284648380432)) ;
#53341=CARTESIAN_POINT('',(2.5,-30.1394375417177,35.5654738138977)) ;
#53342=CARTESIAN_POINT('Origin',(2.5,-31.1848319093482,34.6342645913669)) ;
#53343=CARTESIAN_POINT('Origin',(2.5,-29.7362139999149,35.924654514014)) ;
#53344=CARTESIAN_POINT('Origin',(30.5,1.96278056880054E-12,-2.06095756297191E-12)) ;
#53345=CARTESIAN_POINT('',(30.5,-30.1394375417177,35.5654738138977)) ;
#53346=CARTESIAN_POINT('Origin',(30.5,-29.7362139999149,35.924654514014)) ;
#53347=CARTESIAN_POINT('',(30.5,-32.220213337081,33.6919348724755)) ;
#53348=CARTESIAN_POINT('Origin',(30.5,-31.1848319093482,34.6342645913669)) ;
#53349=CARTESIAN_POINT('Origin',(30.5,-32.6195747449183,33.3284648380432)) ;
#53350=CARTESIAN_POINT('Origin',(30.5,-32.6195747449183,33.3284648380432)) ;
#53351=CARTESIAN_POINT('',(30.5,-32.220213337081,33.6919348724755)) ;
#53352=CARTESIAN_POINT('Origin',(30.5,-31.1848319093482,34.6342645913669)) ;
#53353=CARTESIAN_POINT('',(30.5,-30.1394375417177,35.5654738138977)) ;
#53354=CARTESIAN_POINT('Origin',(30.5,-29.7362139999149,35.924654514014)) ;
#53355=CARTESIAN_POINT('Origin',(2.5,2.16745697839284E-12,-1.84450098521206E-12)) ;
#53356=CARTESIAN_POINT('',(2.5,-35.5654738138976,30.1394375417177)) ;
#53357=CARTESIAN_POINT('Origin',(2.5,-35.9246545140139,29.7362139999149)) ;
#53358=CARTESIAN_POINT('',(2.5,-33.6919348724755,32.220213337081)) ;
#53359=CARTESIAN_POINT('Origin',(2.5,-34.6342645913669,31.1848319093482)) ;
#53360=CARTESIAN_POINT('Origin',(2.5,-33.3284648380432,32.6195747449184)) ;
#53361=CARTESIAN_POINT('Origin',(30.5,2.16745697839284E-12,-1.84450098521206E-12)) ;
#53362=CARTESIAN_POINT('',(30.5,-33.6919348724755,32.220213337081)) ;
#53363=CARTESIAN_POINT('Origin',(30.5,-33.3284648380432,32.6195747449184)) ;
#53364=CARTESIAN_POINT('',(30.5,-35.5654738138976,30.1394375417177)) ;
#53365=CARTESIAN_POINT('Origin',(30.5,-34.6342645913669,31.1848319093482)) ;
#53366=CARTESIAN_POINT('Origin',(30.5,-35.9246545140139,29.7362139999149)) ;
#53367=CARTESIAN_POINT('Origin',(30.5,-35.9246545140139,29.7362139999149)) ;
#53368=CARTESIAN_POINT('',(30.5,-35.5654738138976,30.1394375417177)) ;
#53369=CARTESIAN_POINT('Origin',(30.5,-34.6342645913669,31.1848319093482)) ;
#53370=CARTESIAN_POINT('',(30.5,-33.6919348724755,32.220213337081)) ;
#53371=CARTESIAN_POINT('Origin',(30.5,-33.3284648380432,32.6195747449184)) ;
#53372=CARTESIAN_POINT('Origin',(2.5,1.73659952455823E-12,-2.25483385838873E-12)) ;
#53373=CARTESIAN_POINT('',(2.5,-28.5219414604302,36.8752963142798)) ;
#53374=CARTESIAN_POINT('Origin',(2.5,-28.9571080888325,36.5555620409762)) ;
#53375=CARTESIAN_POINT('',(2.5,-26.2567262261701,38.5210715170554)) ;
#53376=CARTESIAN_POINT('Origin',(2.5,-27.3937316830851,37.7042370228368)) ;
#53377=CARTESIAN_POINT('Origin',(2.5,-25.8181669785007,38.8361362505368)) ;
#53378=CARTESIAN_POINT('Origin',(30.5,1.73659952455823E-12,-2.25483385838873E-12)) ;
#53379=CARTESIAN_POINT('',(30.5,-26.2567262261701,38.5210715170554)) ;
#53380=CARTESIAN_POINT('Origin',(30.5,-25.8181669785007,38.8361362505368)) ;
#53381=CARTESIAN_POINT('',(30.5,-28.5219414604302,36.8752963142798)) ;
#53382=CARTESIAN_POINT('Origin',(30.5,-27.3937316830851,37.7042370228368)) ;
#53383=CARTESIAN_POINT('Origin',(30.5,-28.9571080888325,36.5555620409762)) ;
#53384=CARTESIAN_POINT('Origin',(30.5,-28.9571080888325,36.5555620409762)) ;
#53385=CARTESIAN_POINT('',(30.5,-28.5219414604302,36.8752963142798)) ;
#53386=CARTESIAN_POINT('Origin',(30.5,-27.3937316830851,37.7042370228368)) ;
#53387=CARTESIAN_POINT('',(30.5,-26.2567262261701,38.5210715170554)) ;
#53388=CARTESIAN_POINT('Origin',(30.5,-25.8181669785007,38.8361362505368)) ;
#53389=CARTESIAN_POINT('Origin',(2.5,1.49139193251805E-12,-2.42400572219872E-12)) ;
#53390=CARTESIAN_POINT('',(2.5,-24.5111772245389,39.654644293013)) ;
#53391=CARTESIAN_POINT('Origin',(2.5,-24.9773812968611,39.3821488564452)) ;
#53392=CARTESIAN_POINT('',(2.5,-22.0863407235153,41.0546242996198)) ;
#53393=CARTESIAN_POINT('Origin',(2.5,-23.3024999999952,40.3611139433656)) ;
#53394=CARTESIAN_POINT('Origin',(2.5,-21.6172507168713,41.3221211513147)) ;
#53395=CARTESIAN_POINT('Origin',(30.5,1.49139193251805E-12,-2.42400572219872E-12)) ;
#53396=CARTESIAN_POINT('',(30.5,-22.0863407235153,41.0546242996198)) ;
#53397=CARTESIAN_POINT('Origin',(30.5,-21.6172507168713,41.3221211513147)) ;
#53398=CARTESIAN_POINT('',(30.5,-24.5111772245389,39.654644293013)) ;
#53399=CARTESIAN_POINT('Origin',(30.5,-23.3024999999952,40.3611139433656)) ;
#53400=CARTESIAN_POINT('Origin',(30.5,-24.9773812968611,39.3821488564452)) ;
#53401=CARTESIAN_POINT('Origin',(30.5,-24.9773812968611,39.3821488564452)) ;
#53402=CARTESIAN_POINT('',(30.5,-24.5111772245389,39.654644293013)) ;
#53403=CARTESIAN_POINT('Origin',(30.5,-23.3024999999952,40.3611139433656)) ;
#53404=CARTESIAN_POINT('',(30.5,-22.0863407235153,41.0546242996198)) ;
#53405=CARTESIAN_POINT('Origin',(30.5,-21.6172507168713,41.3221211513147)) ;
#53406=CARTESIAN_POINT('Origin',(2.5,1.22984433837137E-12,-2.5666196720605E-12)) ;
#53407=CARTESIAN_POINT('',(2.5,-20.2318634016821,41.9995276906041)) ;
#53408=CARTESIAN_POINT('Origin',(2.5,-20.7239970885482,41.7772566077985)) ;
#53409=CARTESIAN_POINT('',(2.5,-17.6739726500298,43.1383740271251)) ;
#53410=CARTESIAN_POINT('Origin',(2.5,-18.9559612505438,42.5757860534248)) ;
#53411=CARTESIAN_POINT('Origin',(2.5,-17.1794913326873,43.355372245549)) ;
#53412=CARTESIAN_POINT('Origin',(30.5,1.22984433837137E-12,-2.5666196720605E-12)) ;
#53413=CARTESIAN_POINT('',(30.5,-17.6739726500298,43.1383740271251)) ;
#53414=CARTESIAN_POINT('Origin',(30.5,-17.1794913326873,43.355372245549)) ;
#53415=CARTESIAN_POINT('',(30.5,-20.2318634016821,41.9995276906041)) ;
#53416=CARTESIAN_POINT('Origin',(30.5,-18.9559612505438,42.5757860534248)) ;
#53417=CARTESIAN_POINT('Origin',(30.5,-20.7239970885482,41.7772566077985)) ;
#53418=CARTESIAN_POINT('Origin',(30.5,-20.7239970885482,41.7772566077985)) ;
#53419=CARTESIAN_POINT('',(30.5,-20.2318634016821,41.9995276906041)) ;
#53420=CARTESIAN_POINT('Origin',(30.5,-18.9559612505438,42.5757860534248)) ;
#53421=CARTESIAN_POINT('',(30.5,-17.6739726500298,43.1383740271251)) ;
#53422=CARTESIAN_POINT('Origin',(30.5,-17.1794913326873,43.355372245549)) ;
#53423=CARTESIAN_POINT('Origin',(2.5,9.54822312292022E-13,-2.68111319969549E-12)) ;
#53424=CARTESIAN_POINT('',(2.5,-15.7308850496067,43.8842554738508)) ;
#53425=CARTESIAN_POINT('Origin',(2.5,-16.2435564313579,43.7146439933037)) ;
#53426=CARTESIAN_POINT('',(2.5,-13.067964833674,44.7494907015041)) ;
#53427=CARTESIAN_POINT('Origin',(2.5,-14.4017370228415,44.3239889419266)) ;
#53428=CARTESIAN_POINT('Origin',(2.5,-12.5535098464227,44.9136128087662)) ;
#53429=CARTESIAN_POINT('Origin',(30.5,9.54822312292022E-13,-2.68111319969549E-12)) ;
#53430=CARTESIAN_POINT('',(30.5,-13.067964833674,44.7494907015041)) ;
#53431=CARTESIAN_POINT('Origin',(30.5,-12.5535098464227,44.9136128087662)) ;
#53432=CARTESIAN_POINT('',(30.5,-15.7308850496067,43.8842554738508)) ;
#53433=CARTESIAN_POINT('Origin',(30.5,-14.4017370228415,44.3239889419266)) ;
#53434=CARTESIAN_POINT('Origin',(30.5,-16.2435564313579,43.7146439933037)) ;
#53435=CARTESIAN_POINT('Origin',(30.5,-16.2435564313579,43.7146439933037)) ;
#53436=CARTESIAN_POINT('',(30.5,-15.7308850496067,43.8842554738508)) ;
#53437=CARTESIAN_POINT('Origin',(30.5,-14.4017370228415,44.3239889419266)) ;
#53438=CARTESIAN_POINT('',(30.5,-13.067964833674,44.7494907015041)) ;
#53439=CARTESIAN_POINT('Origin',(30.5,-12.5535098464227,44.9136128087662)) ;
#53440=CARTESIAN_POINT('Origin',(2.5,6.69339053149789E-13,-2.76623189005561E-12)) ;
#53441=CARTESIAN_POINT('',(2.5,-11.0575558290286,45.2881781707551)) ;
#53442=CARTESIAN_POINT('Origin',(2.5,-11.585147970723,45.173084591341)) ;
#53443=CARTESIAN_POINT('',(2.5,-8.3187816599531,45.8703225913245)) ;
#53444=CARTESIAN_POINT('Origin',(2.5,-9.68972435055969,45.5865689321897)) ;
#53445=CARTESIAN_POINT('Origin',(2.5,-7.78998947928983,45.9797704312729)) ;
#53446=CARTESIAN_POINT('Origin',(30.5,6.69339053149789E-13,-2.76623189005561E-12)) ;
#53447=CARTESIAN_POINT('',(30.5,-8.3187816599531,45.8703225913245)) ;
#53448=CARTESIAN_POINT('Origin',(30.5,-7.78998947928983,45.9797704312729)) ;
#53449=CARTESIAN_POINT('',(30.5,-11.0575558290286,45.2881781707551)) ;
#53450=CARTESIAN_POINT('Origin',(30.5,-9.68972435055969,45.5865689321897)) ;
#53451=CARTESIAN_POINT('Origin',(30.5,-11.585147970723,45.173084591341)) ;
#53452=CARTESIAN_POINT('Origin',(30.5,-11.585147970723,45.173084591341)) ;
#53453=CARTESIAN_POINT('',(30.5,-11.0575558290286,45.2881781707551)) ;
#53454=CARTESIAN_POINT('Origin',(30.5,-9.68972435055969,45.5865689321897)) ;
#53455=CARTESIAN_POINT('',(30.5,-8.3187816599531,45.8703225913245)) ;
#53456=CARTESIAN_POINT('Origin',(30.5,-7.78998947928983,45.9797704312729)) ;
#53457=CARTESIAN_POINT('Origin',(2.5,3.76522375273042E-13,-2.82104316495704E-12)) ;
#53458=CARTESIAN_POINT('',(2.5,-6.26307771284528,46.1959141104601)) ;
#53459=CARTESIAN_POINT('Origin',(2.5,-6.7998102045727,46.1365994215198)) ;
#53460=CARTESIAN_POINT('',(2.5,-3.47845617354868,46.4885896278522)) ;
#53461=CARTESIAN_POINT('Origin',(2.5,-4.87154903058796,46.349692933629)) ;
#53462=CARTESIAN_POINT('Origin',(2.5,-2.94112035726176,46.5421640670489)) ;
#53463=CARTESIAN_POINT('Origin',(30.5,3.76522375273042E-13,-2.82104316495704E-12)) ;
#53464=CARTESIAN_POINT('',(30.5,-3.47845617354868,46.4885896278522)) ;
#53465=CARTESIAN_POINT('Origin',(30.5,-2.94112035726176,46.5421640670489)) ;
#53466=CARTESIAN_POINT('',(30.5,-6.26307771284528,46.1959141104601)) ;
#53467=CARTESIAN_POINT('Origin',(30.5,-4.87154903058796,46.349692933629)) ;
#53468=CARTESIAN_POINT('Origin',(30.5,-6.7998102045727,46.1365994215198)) ;
#53469=CARTESIAN_POINT('Origin',(30.5,-6.7998102045727,46.1365994215198)) ;
#53470=CARTESIAN_POINT('',(30.5,-6.26307771284528,46.1959141104601)) ;
#53471=CARTESIAN_POINT('Origin',(30.5,-4.87154903058796,46.349692933629)) ;
#53472=CARTESIAN_POINT('',(30.5,-3.47845617354868,46.4885896278522)) ;
#53473=CARTESIAN_POINT('Origin',(30.5,-2.94112035726176,46.5421640670489)) ;
#53474=CARTESIAN_POINT('Origin',(2.5,7.95804394604358E-14,-2.84494650060196E-12)) ;
#53475=CARTESIAN_POINT('',(2.5,-1.39998000660682,46.5975179480543)) ;
#53476=CARTESIAN_POINT('Origin',(2.5,-1.93997229486942,46.5946320137324)) ;
#53477=CARTESIAN_POINT('',(2.5,1.39998000660682,46.5975179480543)) ;
#53478=CARTESIAN_POINT('Origin',(2.5,2.85373320371254E-15,46.6049999999905)) ;
#53479=CARTESIAN_POINT('Origin',(2.5,1.93997229486942,46.5946320137324)) ;
#53480=CARTESIAN_POINT('Origin',(30.5,7.95804394604358E-14,-2.84494650060196E-12)) ;
#53481=CARTESIAN_POINT('',(30.5,1.39998000660682,46.5975179480543)) ;
#53482=CARTESIAN_POINT('Origin',(30.5,1.93997229486942,46.5946320137324)) ;
#53483=CARTESIAN_POINT('',(30.5,-1.39998000660682,46.5975179480543)) ;
#53484=CARTESIAN_POINT('Origin',(30.5,2.85373320371254E-15,46.6049999999905)) ;
#53485=CARTESIAN_POINT('Origin',(30.5,-1.93997229486942,46.5946320137324)) ;
#53486=CARTESIAN_POINT('Origin',(30.5,-1.93997229486942,46.5946320137324)) ;
#53487=CARTESIAN_POINT('',(30.5,-1.39998000660682,46.5975179480543)) ;
#53488=CARTESIAN_POINT('Origin',(30.5,2.85373320371254E-15,46.6049999999905)) ;
#53489=CARTESIAN_POINT('',(30.5,1.39998000660682,46.5975179480543)) ;
#53490=CARTESIAN_POINT('Origin',(30.5,1.93997229486942,46.5946320137324)) ;
#53491=CARTESIAN_POINT('Origin',(2.5,-2.18233396300179E-13,-2.83768000704297E-12)) ;
#53492=CARTESIAN_POINT('',(2.5,3.47845617354871,46.4885896278521)) ;
#53493=CARTESIAN_POINT('Origin',(2.5,2.94112035726178,46.5421640670489)) ;
#53494=CARTESIAN_POINT('',(2.5,6.26307771284532,46.1959141104601)) ;
#53495=CARTESIAN_POINT('Origin',(2.5,4.871549030588,46.3496929336289)) ;
#53496=CARTESIAN_POINT('Origin',(2.5,6.79981020457273,46.1365994215199)) ;
#53497=CARTESIAN_POINT('Origin',(30.5,-2.18233396300179E-13,-2.83768000704297E-12)) ;
#53498=CARTESIAN_POINT('',(30.5,6.26307771284532,46.1959141104601)) ;
#53499=CARTESIAN_POINT('Origin',(30.5,6.79981020457273,46.1365994215199)) ;
#53500=CARTESIAN_POINT('',(30.5,3.47845617354871,46.4885896278521)) ;
#53501=CARTESIAN_POINT('Origin',(30.5,4.871549030588,46.3496929336289)) ;
#53502=CARTESIAN_POINT('Origin',(30.5,2.94112035726178,46.5421640670489)) ;
#53503=CARTESIAN_POINT('Origin',(30.5,2.94112035726178,46.5421640670489)) ;
#53504=CARTESIAN_POINT('',(30.5,3.47845617354871,46.4885896278521)) ;
#53505=CARTESIAN_POINT('Origin',(30.5,4.871549030588,46.3496929336289)) ;
#53506=CARTESIAN_POINT('',(30.5,6.26307771284532,46.1959141104601)) ;
#53507=CARTESIAN_POINT('Origin',(30.5,6.79981020457273,46.1365994215199)) ;
#53508=CARTESIAN_POINT('Origin',(2.5,-5.13656221302655E-13,-2.79932329750409E-12)) ;
#53509=CARTESIAN_POINT('',(2.5,8.31878165995311,45.8703225913244)) ;
#53510=CARTESIAN_POINT('Origin',(2.5,7.78998947928982,45.9797704312728)) ;
#53511=CARTESIAN_POINT('',(2.5,11.0575558290286,45.2881781707551)) ;
#53512=CARTESIAN_POINT('Origin',(2.5,9.68972435055971,45.5865689321897)) ;
#53513=CARTESIAN_POINT('Origin',(2.5,11.585147970723,45.173084591341)) ;
#53514=CARTESIAN_POINT('Origin',(30.5,-5.13656221302655E-13,-2.79932329750409E-12)) ;
#53515=CARTESIAN_POINT('',(30.5,11.0575558290286,45.2881781707551)) ;
#53516=CARTESIAN_POINT('Origin',(30.5,11.585147970723,45.173084591341)) ;
#53517=CARTESIAN_POINT('',(30.5,8.31878165995311,45.8703225913244)) ;
#53518=CARTESIAN_POINT('Origin',(30.5,9.68972435055971,45.5865689321897)) ;
#53519=CARTESIAN_POINT('Origin',(30.5,7.78998947928982,45.9797704312728)) ;
#53520=CARTESIAN_POINT('Origin',(30.5,7.78998947928982,45.9797704312728)) ;
#53521=CARTESIAN_POINT('',(30.5,8.31878165995311,45.8703225913244)) ;
#53522=CARTESIAN_POINT('Origin',(30.5,9.68972435055971,45.5865689321897)) ;
#53523=CARTESIAN_POINT('',(30.5,11.0575558290286,45.2881781707551)) ;
#53524=CARTESIAN_POINT('Origin',(30.5,11.585147970723,45.173084591341)) ;
#53525=CARTESIAN_POINT('Origin',(2.5,-8.03451321255064E-13,-2.73029661612169E-12)) ;
#53526=CARTESIAN_POINT('',(2.5,13.0679648336741,44.7494907015041)) ;
#53527=CARTESIAN_POINT('Origin',(2.5,12.5535098464227,44.9136128087662)) ;
#53528=CARTESIAN_POINT('',(2.5,15.7308850496068,43.8842554738508)) ;
#53529=CARTESIAN_POINT('Origin',(2.5,14.4017370228415,44.3239889419266)) ;
#53530=CARTESIAN_POINT('Origin',(2.5,16.2435564313579,43.7146439933038)) ;
#53531=CARTESIAN_POINT('Origin',(30.5,-8.03451321255064E-13,-2.73029661612169E-12)) ;
#53532=CARTESIAN_POINT('',(30.5,15.7308850496068,43.8842554738508)) ;
#53533=CARTESIAN_POINT('Origin',(30.5,16.2435564313579,43.7146439933038)) ;
#53534=CARTESIAN_POINT('',(30.5,13.0679648336741,44.7494907015041)) ;
#53535=CARTESIAN_POINT('Origin',(30.5,14.4017370228415,44.3239889419266)) ;
#53536=CARTESIAN_POINT('Origin',(30.5,12.5535098464227,44.9136128087662)) ;
#53537=CARTESIAN_POINT('Origin',(30.5,12.5535098464227,44.9136128087662)) ;
#53538=CARTESIAN_POINT('',(30.5,13.0679648336741,44.7494907015041)) ;
#53539=CARTESIAN_POINT('Origin',(30.5,14.4017370228415,44.3239889419266)) ;
#53540=CARTESIAN_POINT('',(30.5,15.7308850496068,43.8842554738508)) ;
#53541=CARTESIAN_POINT('Origin',(30.5,16.2435564313579,43.7146439933038)) ;
#53542=CARTESIAN_POINT('Origin',(2.5,-1.0844436403988E-12,-2.63135623366177E-12)) ;
#53543=CARTESIAN_POINT('',(2.5,17.6739726500298,43.1383740271251)) ;
#53544=CARTESIAN_POINT('Origin',(2.5,17.1794913326873,43.355372245549)) ;
#53545=CARTESIAN_POINT('',(2.5,20.2318634016821,41.9995276906041)) ;
#53546=CARTESIAN_POINT('Origin',(2.5,18.9559612505438,42.5757860534247)) ;
#53547=CARTESIAN_POINT('Origin',(2.5,20.7239970885482,41.7772566077985)) ;
#53548=CARTESIAN_POINT('Origin',(30.5,-1.0844436403988E-12,-2.63135623366177E-12)) ;
#53549=CARTESIAN_POINT('',(30.5,20.2318634016821,41.9995276906041)) ;
#53550=CARTESIAN_POINT('Origin',(30.5,20.7239970885482,41.7772566077985)) ;
#53551=CARTESIAN_POINT('',(30.5,17.6739726500298,43.1383740271251)) ;
#53552=CARTESIAN_POINT('Origin',(30.5,18.9559612505438,42.5757860534247)) ;
#53553=CARTESIAN_POINT('Origin',(30.5,17.1794913326873,43.355372245549)) ;
#53554=CARTESIAN_POINT('Origin',(30.5,17.1794913326873,43.355372245549)) ;
#53555=CARTESIAN_POINT('',(30.5,17.6739726500298,43.1383740271251)) ;
#53556=CARTESIAN_POINT('Origin',(30.5,18.9559612505438,42.5757860534247)) ;
#53557=CARTESIAN_POINT('',(30.5,20.2318634016821,41.9995276906041)) ;
#53558=CARTESIAN_POINT('Origin',(30.5,20.7239970885482,41.7772566077985)) ;
#53559=CARTESIAN_POINT('Origin',(2.5,-1.35355456808391E-12,-2.50358616165916E-12)) ;
#53560=CARTESIAN_POINT('',(2.5,22.0863407235153,41.0546242996198)) ;
#53561=CARTESIAN_POINT('Origin',(2.5,21.6172507168712,41.3221211513146)) ;
#53562=CARTESIAN_POINT('',(2.5,24.511177224539,39.654644293013)) ;
#53563=CARTESIAN_POINT('Origin',(2.5,23.3024999999952,40.3611139433656)) ;
#53564=CARTESIAN_POINT('Origin',(2.5,24.9773812968611,39.3821488564453)) ;
#53565=CARTESIAN_POINT('Origin',(30.5,-1.35355456808391E-12,-2.50358616165916E-12)) ;
#53566=CARTESIAN_POINT('',(30.5,24.511177224539,39.654644293013)) ;
#53567=CARTESIAN_POINT('Origin',(30.5,24.9773812968611,39.3821488564453)) ;
#53568=CARTESIAN_POINT('',(30.5,22.0863407235153,41.0546242996198)) ;
#53569=CARTESIAN_POINT('Origin',(30.5,23.3024999999952,40.3611139433656)) ;
#53570=CARTESIAN_POINT('Origin',(30.5,21.6172507168712,41.3221211513146)) ;
#53571=CARTESIAN_POINT('Origin',(30.5,21.6172507168712,41.3221211513146)) ;
#53572=CARTESIAN_POINT('',(30.5,22.0863407235153,41.0546242996198)) ;
#53573=CARTESIAN_POINT('Origin',(30.5,23.3024999999952,40.3611139433656)) ;
#53574=CARTESIAN_POINT('',(30.5,24.511177224539,39.654644293013)) ;
#53575=CARTESIAN_POINT('Origin',(30.5,24.9773812968611,39.3821488564453)) ;
#53576=CARTESIAN_POINT('Origin',(2.5,-2.25483385838873E-12,-1.73659952455823E-12)) ;
#53577=CARTESIAN_POINT('',(2.5,36.8752963142797,28.5219414604302)) ;
#53578=CARTESIAN_POINT('Origin',(2.5,36.5555620409762,28.9571080888326)) ;
#53579=CARTESIAN_POINT('',(2.5,38.5210715170554,26.2567262261701)) ;
#53580=CARTESIAN_POINT('Origin',(2.5,37.7042370228368,27.3937316830851)) ;
#53581=CARTESIAN_POINT('Origin',(2.5,38.8361362505368,25.8181669785007)) ;
#53582=CARTESIAN_POINT('Origin',(30.5,-2.25483385838873E-12,-1.73659952455823E-12)) ;
#53583=CARTESIAN_POINT('',(30.5,38.5210715170554,26.2567262261701)) ;
#53584=CARTESIAN_POINT('Origin',(30.5,38.8361362505368,25.8181669785007)) ;
#53585=CARTESIAN_POINT('',(30.5,36.8752963142797,28.5219414604302)) ;
#53586=CARTESIAN_POINT('Origin',(30.5,37.7042370228368,27.3937316830851)) ;
#53587=CARTESIAN_POINT('Origin',(30.5,36.5555620409762,28.9571080888326)) ;
#53588=CARTESIAN_POINT('Origin',(30.5,36.5555620409762,28.9571080888326)) ;
#53589=CARTESIAN_POINT('',(30.5,36.8752963142797,28.5219414604302)) ;
#53590=CARTESIAN_POINT('Origin',(30.5,37.7042370228368,27.3937316830851)) ;
#53591=CARTESIAN_POINT('',(30.5,38.5210715170554,26.2567262261701)) ;
#53592=CARTESIAN_POINT('Origin',(30.5,38.8361362505368,25.8181669785007)) ;
#53593=CARTESIAN_POINT('Origin',(2.5,-2.0609575629719E-12,-1.96278056880054E-12)) ;
#53594=CARTESIAN_POINT('',(2.5,33.6919348724754,32.220213337081)) ;
#53595=CARTESIAN_POINT('Origin',(2.5,33.3284648380432,32.6195747449183)) ;
#53596=CARTESIAN_POINT('',(2.5,35.5654738138977,30.1394375417177)) ;
#53597=CARTESIAN_POINT('Origin',(2.5,34.6342645913669,31.1848319093482)) ;
#53598=CARTESIAN_POINT('Origin',(2.5,35.924654514014,29.7362139999149)) ;
#53599=CARTESIAN_POINT('Origin',(30.5,-2.0609575629719E-12,-1.96278056880054E-12)) ;
#53600=CARTESIAN_POINT('',(30.5,35.5654738138977,30.1394375417177)) ;
#53601=CARTESIAN_POINT('Origin',(30.5,35.924654514014,29.7362139999149)) ;
#53602=CARTESIAN_POINT('',(30.5,33.6919348724754,32.220213337081)) ;
#53603=CARTESIAN_POINT('Origin',(30.5,34.6342645913669,31.1848319093482)) ;
#53604=CARTESIAN_POINT('Origin',(30.5,33.3284648380432,32.6195747449183)) ;
#53605=CARTESIAN_POINT('Origin',(30.5,33.3284648380432,32.6195747449183)) ;
#53606=CARTESIAN_POINT('',(30.5,33.6919348724754,32.220213337081)) ;
#53607=CARTESIAN_POINT('Origin',(30.5,34.6342645913669,31.1848319093482)) ;
#53608=CARTESIAN_POINT('',(30.5,35.5654738138977,30.1394375417177)) ;
#53609=CARTESIAN_POINT('Origin',(30.5,35.924654514014,29.7362139999149)) ;
#53610=CARTESIAN_POINT('Origin',(2.5,-1.84450098521206E-12,-2.16745697839283E-12)) ;
#53611=CARTESIAN_POINT('',(2.5,30.1394375417177,35.5654738138976)) ;
#53612=CARTESIAN_POINT('Origin',(2.5,29.7362139999149,35.9246545140139)) ;
#53613=CARTESIAN_POINT('',(2.5,32.2202133370811,33.6919348724755)) ;
#53614=CARTESIAN_POINT('Origin',(2.5,31.1848319093483,34.6342645913669)) ;
#53615=CARTESIAN_POINT('Origin',(2.5,32.6195747449184,33.3284648380432)) ;
#53616=CARTESIAN_POINT('Origin',(30.5,-1.84450098521206E-12,-2.16745697839283E-12)) ;
#53617=CARTESIAN_POINT('',(30.5,32.2202133370811,33.6919348724755)) ;
#53618=CARTESIAN_POINT('Origin',(30.5,32.6195747449184,33.3284648380432)) ;
#53619=CARTESIAN_POINT('',(30.5,30.1394375417177,35.5654738138976)) ;
#53620=CARTESIAN_POINT('Origin',(30.5,31.1848319093483,34.6342645913669)) ;
#53621=CARTESIAN_POINT('Origin',(30.5,29.7362139999149,35.9246545140139)) ;
#53622=CARTESIAN_POINT('Origin',(30.5,29.7362139999149,35.9246545140139)) ;
#53623=CARTESIAN_POINT('',(30.5,30.1394375417177,35.5654738138976)) ;
#53624=CARTESIAN_POINT('Origin',(30.5,31.1848319093483,34.6342645913669)) ;
#53625=CARTESIAN_POINT('',(30.5,32.2202133370811,33.6919348724755)) ;
#53626=CARTESIAN_POINT('Origin',(30.5,32.6195747449184,33.3284648380432)) ;
#53627=CARTESIAN_POINT('Origin',(2.5,-1.60783566867159E-12,-2.34838627576032E-12)) ;
#53628=CARTESIAN_POINT('',(2.5,26.2567262261701,38.5210715170554)) ;
#53629=CARTESIAN_POINT('Origin',(2.5,25.8181669785007,38.8361362505367)) ;
#53630=CARTESIAN_POINT('',(2.5,28.5219414604302,36.8752963142798)) ;
#53631=CARTESIAN_POINT('Origin',(2.5,27.3937316830851,37.7042370228368)) ;
#53632=CARTESIAN_POINT('Origin',(2.5,28.9571080888326,36.5555620409763)) ;
#53633=CARTESIAN_POINT('Origin',(30.5,-1.60783566867159E-12,-2.34838627576032E-12)) ;
#53634=CARTESIAN_POINT('',(30.5,28.5219414604302,36.8752963142798)) ;
#53635=CARTESIAN_POINT('Origin',(30.5,28.9571080888326,36.5555620409763)) ;
#53636=CARTESIAN_POINT('',(30.5,26.2567262261701,38.5210715170554)) ;
#53637=CARTESIAN_POINT('Origin',(30.5,27.3937316830851,37.7042370228368)) ;
#53638=CARTESIAN_POINT('Origin',(30.5,25.8181669785007,38.8361362505367)) ;
#53639=CARTESIAN_POINT('Origin',(30.5,25.8181669785007,38.8361362505367)) ;
#53640=CARTESIAN_POINT('',(30.5,26.2567262261701,38.5210715170554)) ;
#53641=CARTESIAN_POINT('Origin',(30.5,27.3937316830851,37.7042370228368)) ;
#53642=CARTESIAN_POINT('',(30.5,28.5219414604302,36.8752963142798)) ;
#53643=CARTESIAN_POINT('Origin',(30.5,28.9571080888326,36.5555620409763)) ;
#53644=CARTESIAN_POINT('Origin',(2.5,-2.42400572219872E-12,-1.49139193251805E-12)) ;
#53645=CARTESIAN_POINT('',(2.5,39.6546442930129,24.511177224539)) ;
#53646=CARTESIAN_POINT('Origin',(2.5,39.3821488564452,24.9773812968611)) ;
#53647=CARTESIAN_POINT('',(2.5,41.0546242996198,22.0863407235154)) ;
#53648=CARTESIAN_POINT('Origin',(2.5,40.3611139433656,23.3024999999953)) ;
#53649=CARTESIAN_POINT('Origin',(2.5,41.3221211513147,21.6172507168713)) ;
#53650=CARTESIAN_POINT('Origin',(30.5,-2.42400572219872E-12,-1.49139193251805E-12)) ;
#53651=CARTESIAN_POINT('',(30.5,41.0546242996198,22.0863407235154)) ;
#53652=CARTESIAN_POINT('Origin',(30.5,41.3221211513147,21.6172507168713)) ;
#53653=CARTESIAN_POINT('',(30.5,39.6546442930129,24.511177224539)) ;
#53654=CARTESIAN_POINT('Origin',(30.5,40.3611139433656,23.3024999999953)) ;
#53655=CARTESIAN_POINT('Origin',(30.5,39.3821488564452,24.9773812968611)) ;
#53656=CARTESIAN_POINT('Origin',(30.5,39.3821488564452,24.9773812968611)) ;
#53657=CARTESIAN_POINT('',(30.5,39.6546442930129,24.511177224539)) ;
#53658=CARTESIAN_POINT('Origin',(30.5,40.3611139433656,23.3024999999953)) ;
#53659=CARTESIAN_POINT('',(30.5,41.0546242996198,22.0863407235154)) ;
#53660=CARTESIAN_POINT('Origin',(30.5,41.3221211513147,21.6172507168713)) ;
#53661=CARTESIAN_POINT('Origin',(2.5,-2.5666196720605E-12,-1.22984433837137E-12)) ;
#53662=CARTESIAN_POINT('',(2.5,41.9995276906041,20.2318634016821)) ;
#53663=CARTESIAN_POINT('Origin',(2.5,41.7772566077985,20.7239970885482)) ;
#53664=CARTESIAN_POINT('',(2.5,43.1383740271251,17.6739726500298)) ;
#53665=CARTESIAN_POINT('Origin',(2.5,42.5757860534247,18.9559612505438)) ;
#53666=CARTESIAN_POINT('Origin',(2.5,43.355372245549,17.1794913326873)) ;
#53667=CARTESIAN_POINT('Origin',(30.5,-2.5666196720605E-12,-1.22984433837137E-12)) ;
#53668=CARTESIAN_POINT('',(30.5,43.1383740271251,17.6739726500298)) ;
#53669=CARTESIAN_POINT('Origin',(30.5,43.355372245549,17.1794913326873)) ;
#53670=CARTESIAN_POINT('',(30.5,41.9995276906041,20.2318634016821)) ;
#53671=CARTESIAN_POINT('Origin',(30.5,42.5757860534247,18.9559612505438)) ;
#53672=CARTESIAN_POINT('Origin',(30.5,41.7772566077985,20.7239970885482)) ;
#53673=CARTESIAN_POINT('Origin',(30.5,41.7772566077985,20.7239970885482)) ;
#53674=CARTESIAN_POINT('',(30.5,41.9995276906041,20.2318634016821)) ;
#53675=CARTESIAN_POINT('Origin',(30.5,42.5757860534247,18.9559612505438)) ;
#53676=CARTESIAN_POINT('',(30.5,43.1383740271251,17.6739726500298)) ;
#53677=CARTESIAN_POINT('Origin',(30.5,43.355372245549,17.1794913326873)) ;
#53678=CARTESIAN_POINT('Origin',(2.5,-2.68111319969549E-12,-9.54822312292023E-13)) ;
#53679=CARTESIAN_POINT('',(2.5,43.8842554738508,15.7308850496067)) ;
#53680=CARTESIAN_POINT('Origin',(2.5,43.7146439933037,16.2435564313579)) ;
#53681=CARTESIAN_POINT('',(2.5,44.7494907015041,13.0679648336741)) ;
#53682=CARTESIAN_POINT('Origin',(2.5,44.3239889419266,14.4017370228415)) ;
#53683=CARTESIAN_POINT('Origin',(2.5,44.9136128087662,12.5535098464227)) ;
#53684=CARTESIAN_POINT('Origin',(30.5,-2.68111319969549E-12,-9.54822312292023E-13)) ;
#53685=CARTESIAN_POINT('',(30.5,44.7494907015041,13.0679648336741)) ;
#53686=CARTESIAN_POINT('Origin',(30.5,44.9136128087662,12.5535098464227)) ;
#53687=CARTESIAN_POINT('',(30.5,43.8842554738508,15.7308850496067)) ;
#53688=CARTESIAN_POINT('Origin',(30.5,44.3239889419266,14.4017370228415)) ;
#53689=CARTESIAN_POINT('Origin',(30.5,43.7146439933037,16.2435564313579)) ;
#53690=CARTESIAN_POINT('Origin',(30.5,43.7146439933037,16.2435564313579)) ;
#53691=CARTESIAN_POINT('',(30.5,43.8842554738508,15.7308850496067)) ;
#53692=CARTESIAN_POINT('Origin',(30.5,44.3239889419266,14.4017370228415)) ;
#53693=CARTESIAN_POINT('',(30.5,44.7494907015041,13.0679648336741)) ;
#53694=CARTESIAN_POINT('Origin',(30.5,44.9136128087662,12.5535098464227)) ;
#53695=CARTESIAN_POINT('Origin',(2.5,-2.76623189005561E-12,-6.69339053149789E-13)) ;
#53696=CARTESIAN_POINT('',(2.5,45.2881781707551,11.0575558290286)) ;
#53697=CARTESIAN_POINT('Origin',(2.5,45.173084591341,11.585147970723)) ;
#53698=CARTESIAN_POINT('',(2.5,45.8703225913245,8.31878165995311)) ;
#53699=CARTESIAN_POINT('Origin',(2.5,45.5865689321897,9.6897243505597)) ;
#53700=CARTESIAN_POINT('Origin',(2.5,45.9797704312729,7.78998947928984)) ;
#53701=CARTESIAN_POINT('Origin',(30.5,-2.76623189005561E-12,-6.69339053149789E-13)) ;
#53702=CARTESIAN_POINT('',(30.5,45.8703225913245,8.31878165995311)) ;
#53703=CARTESIAN_POINT('Origin',(30.5,45.9797704312729,7.78998947928984)) ;
#53704=CARTESIAN_POINT('',(30.5,45.2881781707551,11.0575558290286)) ;
#53705=CARTESIAN_POINT('Origin',(30.5,45.5865689321897,9.6897243505597)) ;
#53706=CARTESIAN_POINT('Origin',(30.5,45.173084591341,11.585147970723)) ;
#53707=CARTESIAN_POINT('Origin',(30.5,45.173084591341,11.585147970723)) ;
#53708=CARTESIAN_POINT('',(30.5,45.2881781707551,11.0575558290286)) ;
#53709=CARTESIAN_POINT('Origin',(30.5,45.5865689321897,9.6897243505597)) ;
#53710=CARTESIAN_POINT('',(30.5,45.8703225913245,8.31878165995311)) ;
#53711=CARTESIAN_POINT('Origin',(30.5,45.9797704312729,7.78998947928984)) ;
#53712=CARTESIAN_POINT('Origin',(45.,0.,0.)) ;
#63800=UNCERTAINTY_MEASURE_WITH_UNIT(LENGTH_MEASURE(0.01),#63825,
'DISTANCE_ACCURACY_VALUE',
'Maximum model space distance between geometric entities at asserted c
onnectivities') ;
#63807=UNCERTAINTY_MEASURE_WITH_UNIT(LENGTH_MEASURE(0.01),#63825,
'DISTANCE_ACCURACY_VALUE',
'Maximum model space distance between geometric entities at asserted c
onnectivities') ;
#63817=(
GEOMETRIC_REPRESENTATION_CONTEXT(3)
GLOBAL_UNCERTAINTY_ASSIGNED_CONTEXT((#63800))
GLOBAL_UNIT_ASSIGNED_CONTEXT((#63825,#63827,#63828))
REPRESENTATION_CONTEXT('','3D')
) ;
#63824=(
GEOMETRIC_REPRESENTATION_CONTEXT(3)
GLOBAL_UNCERTAINTY_ASSIGNED_CONTEXT((#63807))
GLOBAL_UNIT_ASSIGNED_CONTEXT((#63825,#63827,#63828))
REPRESENTATION_CONTEXT('','3D')
) ;
#63825=(
LENGTH_UNIT()
NAMED_UNIT(*)
SI_UNIT(.MILLI.,.METRE.)
) ;
#63827=(
NAMED_UNIT(*)
PLANE_ANGLE_UNIT()
SI_UNIT($,.RADIAN.)
) ;
#63828=(
NAMED_UNIT(*)
SI_UNIT($,.STERADIAN.)
SOLID_ANGLE_UNIT()
) ;
#63838=SHAPE_DEFINITION_REPRESENTATION(#63854,#63887) ;
#63854=PRODUCT_DEFINITION_SHAPE('',$,#63904) ;
#63887=SHAPE_REPRESENTATION('',(#16208),#63817) ;
#63894=PRODUCT_DEFINITION_CONTEXT('part definition',#63944,'design') ;
#63904=PRODUCT_DEFINITION('Drive_Pulley','Drive_Pulley',#63920,#63894) ;
#63920=PRODUCT_DEFINITION_FORMATION('',$,#63955) ;
#63944=APPLICATION_CONTEXT(
'Core Data for Automotive Mechanical Design Process') ;
#63945=PRODUCT_CONTEXT('part definition',#63944,'mechanical') ;
#63955=PRODUCT('Drive_Pulley','Drive_Pulley',$,(#63945)) ;
#63965=PRESENTATION_STYLE_ASSIGNMENT((#63970)) ;
#63970=SURFACE_STYLE_USAGE(.BOTH.,#63975) ;
#63975=SURFACE_SIDE_STYLE('',(#63980)) ;
#63980=SURFACE_STYLE_FILL_AREA(#63985) ;
#63985=FILL_AREA_STYLE('Opaque(245,245,246)',(#63990)) ;
#63990=FILL_AREA_STYLE_COLOUR('Opaque(245,245,246)',#63995) ;
#63995=COLOUR_RGB('Opaque(245,245,246)', 0.31764706, 0.68627451, 0.89019608) ;
ENDSEC;
END-ISO-10303-21;
